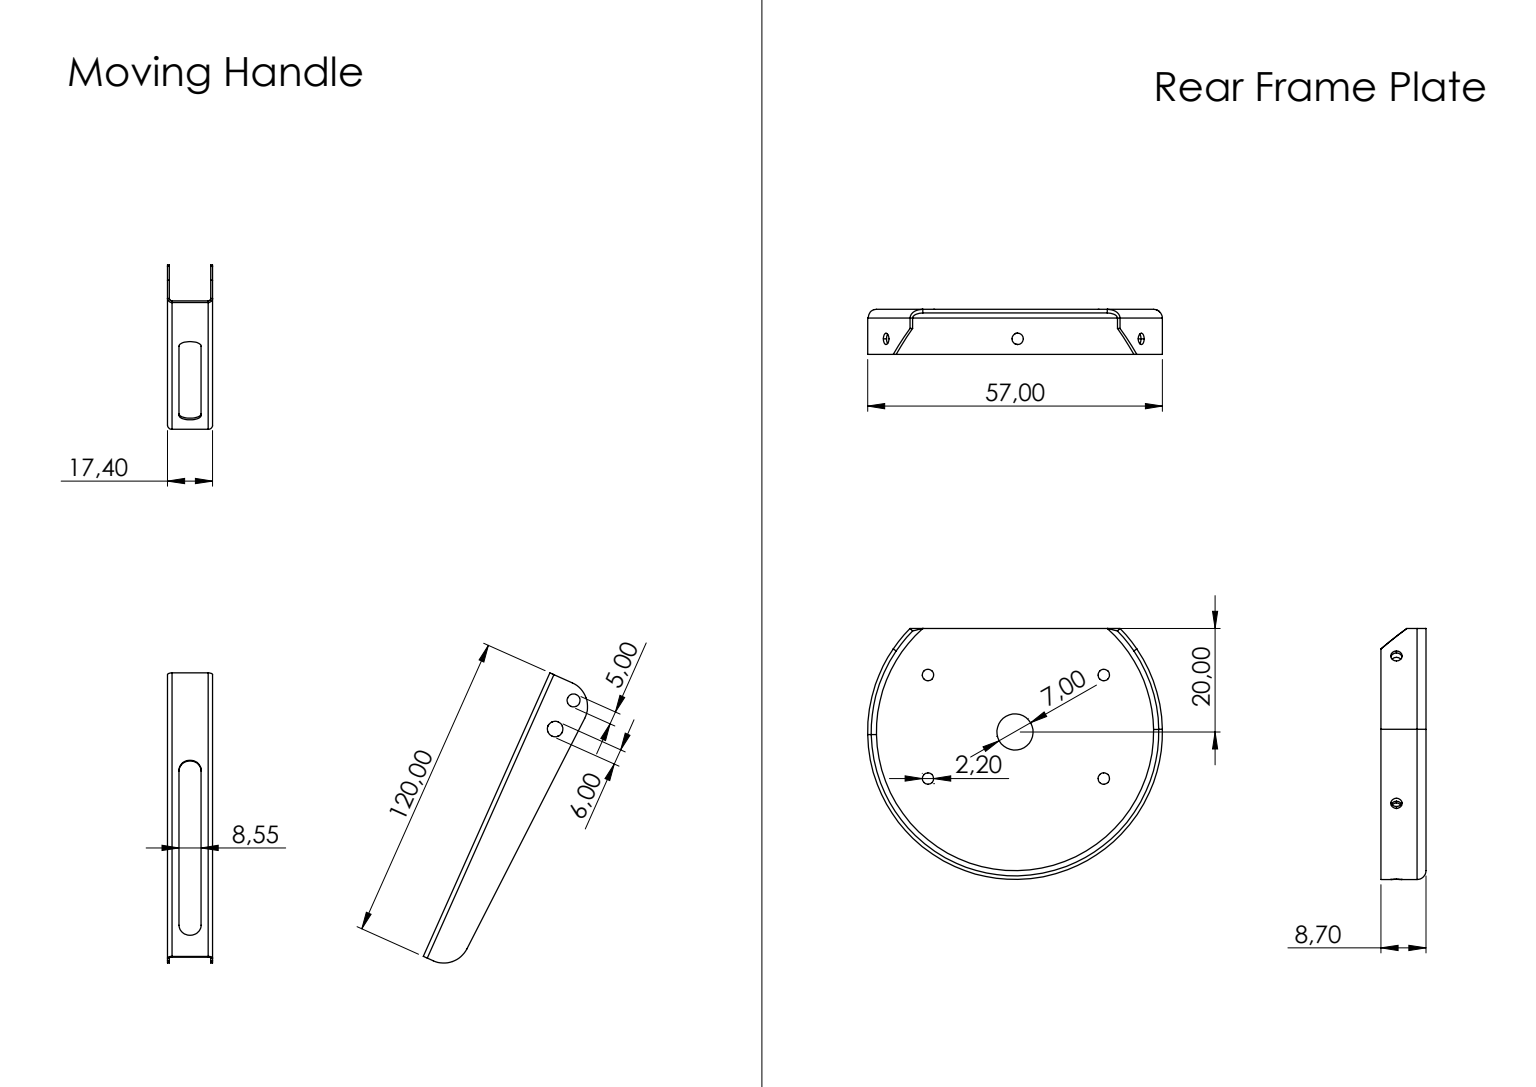
ISO-10303-21;
HEADER;
FILE_DESCRIPTION (('STEP AP214'),
    '1' );
FILE_NAME ('Rear Frame Plate.step',
    '2026-10-06T09:00:30',
    ( '' ),
    ( '' ),
    'SwSTEP 2.0',
    'SolidWorks 2020',
    '' );
FILE_SCHEMA (( 'AUTOMOTIVE_DESIGN' ));
ENDSEC;

DATA;
#10=CARTESIAN_POINT ( 'NONE',  ( -15.86372219731129896, -9.538245303637634009, -0.6999999999999785283 ) ) ;
#12=ORIENTED_EDGE ( 'NONE', *, *, #12651, .T. ) ;
#13=CARTESIAN_POINT ( 'NONE',  ( 25.25401215818320821, -13.21081861402980273, 4.098596794000014754 ) ) ;
#24=FACE_OUTER_BOUND ( 'NONE', #15323, .T. ) ;
#26=CARTESIAN_POINT ( 'NONE',  ( 18.18796211431769549, 19.99998853575082336, -0.6839386825886580867 ) ) ;
#31=ORIENTED_EDGE ( 'NONE', *, *, #12379, .F. ) ;
#36=B_SPLINE_CURVE_WITH_KNOTS ( 'NONE', 3,
 ( #5890, #1034, #22739, #5586, #10623, #27300 ),
 .UNSPECIFIED., .F., .F.,
 ( 4, 2, 4 ),
 ( 0.000000000000000000, 0.5000000000000000000, 1.000000000000000000 ),
 .UNSPECIFIED. ) ;
#37=CARTESIAN_POINT ( 'NONE',  ( 24.70074545475921823, -14.21822122957610368, 6.002806299999996043 ) ) ;
#38=CARTESIAN_POINT ( 'NONE',  ( 19.56389002122311638, 19.56882009050699622, 0.5006759800000037952 ) ) ;
#43=CARTESIAN_POINT ( 'NONE',  ( -24.83401023410189623, -13.98326748962921329, 4.239871886000001311 ) ) ;
#47=CARTESIAN_POINT ( 'NONE',  ( 0.5184513693225318853, -28.49550581263314086, 3.899998581000013509 ) ) ;
#51=CARTESIAN_POINT ( 'NONE',  ( -20.30403093128963476, 20.00000000003735323, 3.000000106999994642 ) ) ;
#65=CARTESIAN_POINT ( 'NONE',  ( 17.83929014045347827, 20.00000000006149392, -1.000005633855494125E-09 ) ) ;
#69=CARTESIAN_POINT ( 'NONE',  ( -18.27629205756926822, 19.99998488772503080, -0.6746503638753708065 ) ) ;
#72=MANIFOLD_SOLID_BREP ( 'PartBody', #5507 ) ;
#77=CARTESIAN_POINT ( 'NONE',  ( 16.21564467631812789, 10.42862492216662318, -0.6999999999999785283 ) ) ;
#88=CARTESIAN_POINT ( 'NONE',  ( -27.88265104574380260, 4.289521473631270787, 0.8585786439999909536 ) ) ;
#92=AXIS2_PLACEMENT_3D ( 'NONE', #8995, #11519, #1614 ) ;
#101=ADVANCED_FACE ( 'NONE', ( #28332 ), #9497, .F. ) ;
#103=CARTESIAN_POINT ( 'NONE',  ( 17.95841148951064525, -9.763538383420391042, -0.6999999999999784173 ) ) ;
#119=CARTESIAN_POINT ( 'NONE',  ( -24.32472894358752313, 13.45989150749028873, 3.899998581000013509 ) ) ;
#123=CARTESIAN_POINT ( 'NONE',  ( 17.93011078765611543, -8.208160914697428368, -0.6999999999999784173 ) ) ;
#126=CARTESIAN_POINT ( 'NONE',  ( 19.80526555972147307, 19.50877392102524155, 1.800000000000023803 ) ) ;
#144=DIRECTION ( 'NONE',  ( -0.6941258031311203780, -0.7198537139083029945, 0.000000000000000000 ) ) ;
#153=CARTESIAN_POINT ( 'NONE',  ( -18.31085446006445494, 19.88197403644849004, 0.02160863700001458554 ) ) ;
#164=FACE_OUTER_BOUND ( 'NONE', #30752, .T. ) ;
#170=VERTEX_POINT ( 'NONE', #24397 ) ;
#171=CARTESIAN_POINT ( 'NONE',  ( -17.59696554489119080, -9.791838634853515799, 0.000000000000000000 ) ) ;
#174=CARTESIAN_POINT ( 'NONE',  ( 23.47715715134837211, -20.00370206646827498, 1.000000000000000888 ) ) ;
#176=CARTESIAN_POINT ( 'NONE',  ( 19.80526555972147307, 19.50877392102524155, 8.000000000000007105 ) ) ;
#178=CARTESIAN_POINT ( 'NONE',  ( 19.37011161855012986, 20.00004249230521935, -0.3429596948707999693 ) ) ;
#179=CARTESIAN_POINT ( 'NONE',  ( -24.00289803497245700, 14.02635913871703011, 5.901399683999997592 ) ) ;
#198=CARTESIAN_POINT ( 'NONE',  ( 16.37473331889771089, 11.76353838340827984, 0.000000000000000000 ) ) ;
#214=CARTESIAN_POINT ( 'NONE',  ( -24.82162973577514364, 12.51998933611906573, 5.310645680000003921 ) ) ;
#219=CARTESIAN_POINT ( 'NONE',  ( 3.040504021322313122, 1.733590290792417887, 0.000000000000000000 ) ) ;
#245=ADVANCED_FACE ( 'NONE', ( #491 ), #28838, .T. ) ;
#250=LINE ( 'NONE', #26663, #23008 ) ;
#254=CARTESIAN_POINT ( 'NONE',  ( -18.80686365405603055, 19.99999823163966184, -0.5856999480000069092 ) ) ;
#257=B_SPLINE_SURFACE_WITH_KNOTS ( 'NONE', 5, 1, ( 
 ( #21157, #21469 ),
 ( #23836, #30754 ),
 ( #16430, #9183 ),
 ( #14231, #2282 ),
 ( #11866, #28394 ),
 ( #6831, #11711 ),
 ( #21312, #7144 ),
 ( #26039, #4479 ),
 ( #11245, #28076 ),
 ( #9342, #20853 ),
 ( #18943, #26346 ),
 ( #4794, #7602 ),
 ( #19727, #10128 ),
 ( #21937, #19414 ),
 ( #26800, #17195 ) ),
 .UNSPECIFIED., .F., .F., .F.,
 ( 6, 3, 3, 3, 6 ),
 ( 2, 2 ),
 ( 0.000000000000000000, 0.5239015562240000312, 1.047803112450000018, 1.571704668670000027, 1.746338520749999956 ),
 ( -0.7000000000009999335, 2.556819966299999618E-06 ),
 .UNSPECIFIED. ) ;
#269=CARTESIAN_POINT ( 'NONE',  ( -23.23277126416379801, -15.26692729116844482, 5.104183903000020450 ) ) ;
#272=STYLED_ITEM ( 'NONE', ( #2224 ), #72 ) ;
#275=CARTESIAN_POINT ( 'NONE',  ( -4.583497702006505747, -30.37373325290905868, -0.6577119969999878357 ) ) ;
#279=CARTESIAN_POINT ( 'NONE',  ( 28.49528339128749366, 0.5184828350247753237, 8.000000000000007105 ) ) ;
#282=CARTESIAN_POINT ( 'NONE',  ( -16.81618662976075740, -7.899504219251200610, 0.000000000000000000 ) ) ;
#283=CARTESIAN_POINT ( 'NONE',  ( 24.86822223037987456, 13.92223202030449691, 5.680679506000013923 ) ) ;
#284=EDGE_CURVE ( 'NONE', #12548, #25224, #27851, .T. ) ;
#286=CARTESIAN_POINT ( 'NONE',  ( 20.30396079662882158, 20.00000000004802203, 2.200000000000007283 ) ) ;
#291=EDGE_CURVE ( 'NONE', #28488, #24538, #21849, .T. ) ;
#295=ORIENTED_EDGE ( 'NONE', *, *, #24858, .F. ) ;
#301=CARTESIAN_POINT ( 'NONE',  ( -27.79539923781684507, -0.5057481689249115897, 6.600000000000022737 ) ) ;
#307=ORIENTED_EDGE ( 'NONE', *, *, #28551, .T. ) ;
#309=CARTESIAN_POINT ( 'NONE',  ( -24.96253706803760153, -13.75225324404262572, 4.689458291000009105 ) ) ;
#325=ORIENTED_EDGE ( 'NONE', *, *, #21114, .F. ) ;
#326=CARTESIAN_POINT ( 'NONE',  ( 25.05552768372066907, -13.58331698798256504, 3.920132093000017193 ) ) ;
#335=CARTESIAN_POINT ( 'NONE',  ( 17.14656078599760392, 12.09981795542235439, -0.6999999999999784173 ) ) ;
#347=CARTESIAN_POINT ( 'NONE',  ( -1.108738578190967550, -3.350312884103880950, 0.000000000000000000 ) ) ;
#349=CARTESIAN_POINT ( 'NONE',  ( 23.83639842146205368, 14.30623132797946084, 6.099998581000020792 ) ) ;
#353=EDGE_CURVE ( 'NONE', #27389, #17896, #14711, .T. ) ;
#365=ORIENTED_EDGE ( 'NONE', *, *, #11993, .F. ) ;
#367=ORIENTED_EDGE ( 'NONE', *, *, #29552, .F. ) ;
#415=CARTESIAN_POINT ( 'NONE',  ( -23.47637529058820860, -14.89020704899713365, 4.098700198000015504 ) ) ;
#416=B_SPLINE_SURFACE_WITH_KNOTS ( 'NONE', 5, 1, ( 
 ( #8599, #18199 ),
 ( #6254, #14591 ),
 ( #24030, #21979 ),
 ( #14278, #7033 ),
 ( #4834, #16622 ),
 ( #17088, #24179 ),
 ( #30954, #26082 ),
 ( #19146, #23884 ),
 ( #18832, #2323 ),
 ( #2471, #16469 ),
 ( #21669, #26392 ),
 ( #16775, #28434 ),
 ( #9549, #14431 ),
 ( #2781, #4521 ),
 ( #14119, #119 ) ),
 .UNSPECIFIED., .F., .F., .F.,
 ( 6, 3, 3, 3, 6 ),
 ( 2, 2 ),
 ( 0.000000000000000000, 0.5239049113340000785, 1.047809822670000113, 1.571714733999999947, 1.746349704450000040 ),
 ( -0.7000000000009999335, 2.557518061549999935E-06 ),
 .UNSPECIFIED. ) ;
#417=CARTESIAN_POINT ( 'NONE',  ( -19.80535397421925481, 19.50875616500616871, 0.9999999989999952543 ) ) ;
#434=CARTESIAN_POINT ( 'NONE',  ( -28.35945636591989683, -7.983396444576476902, 0.7595836940000044724 ) ) ;
#442=VECTOR ( 'NONE', #12389, 1000.000000000000000 ) ;
#443=CARTESIAN_POINT ( 'NONE',  ( 19.80526555962148549, 19.50877392102342256, 1.000000000000000888 ) ) ;
#455=CARTESIAN_POINT ( 'NONE',  ( -16.66884554142874464, -10.09718743908464234, -0.6999999999999783062 ) ) ;
#479=ORIENTED_EDGE ( 'NONE', *, *, #10437, .F. ) ;
#490=CARTESIAN_POINT ( 'NONE',  ( -16.83342759575507586, 10.99999999997565503, -0.6999999999999784173 ) ) ;
#491=FACE_OUTER_BOUND ( 'NONE', #749, .T. ) ;
#510=CARTESIAN_POINT ( 'NONE',  ( 0.5057536231481192246, -27.79562098839016571, 6.099998581000020792 ) ) ;
#511=CARTESIAN_POINT ( 'NONE',  ( -23.81866173682177390, -14.33570044646243247, 3.899998581000013509 ) ) ;
#512=CARTESIAN_POINT ( 'NONE',  ( 16.27478637877570833, 11.65988689034672809, -4.336808689942018722E-16 ) ) ;
#519=B_SPLINE_CURVE_WITH_KNOTS ( 'NONE', 5,
 ( #763, #19799, #26878, #10508, #7824, #14617, #22156, #5319, #27336, #14923, #24519, #22311, #2956, #20108, #29696 ),
 .UNSPECIFIED., .F., .F.,
 ( 6, 3, 3, 3, 6 ),
 ( 0.000000000000000000, 0.3000000000005726419, 0.6000000000000000888, 0.9000000000028631764, 1.000000000000000000 ),
 .UNSPECIFIED. ) ;
#534=CARTESIAN_POINT ( 'NONE',  ( -24.78870452935070290, 12.58522324297991268, 5.507123707999994622 ) ) ;
#535=FACE_BOUND ( 'NONE', #29200, .T. ) ;
#539=AXIS2_PLACEMENT_3D ( 'NONE', #23049, #13598, #18623 ) ;
#556=CARTESIAN_POINT ( 'NONE',  ( -26.39324905318550307, 9.701294701415816846, 8.000000000000007105 ) ) ;
#573=CARTESIAN_POINT ( 'NONE',  ( -25.38146355678814814, 12.59839640969361696, 1.000000000000000888 ) ) ;
#581=CARTESIAN_POINT ( 'NONE',  ( -23.25311087912443853, -15.23597700045676895, 5.310552105000033052 ) ) ;
#586=CARTESIAN_POINT ( 'NONE',  ( -4.785279987089964493, -31.71089578132167119, 1.000000000000000888 ) ) ;
#601=ORIENTED_EDGE ( 'NONE', *, *, #21982, .T. ) ;
#603=CARTESIAN_POINT ( 'NONE',  ( -24.29138540600951046, 13.52003710149997140, 3.901342110999989288 ) ) ;
#609=AXIS2_PLACEMENT_3D ( 'NONE', #4921, #21294, #28527 ) ;
#623=EDGE_CURVE ( 'NONE', #12633, #11464, #6060, .T. ) ;
#654=CARTESIAN_POINT ( 'NONE',  ( 24.92013865993870425, -13.82966158318416738, 6.099998581000020792 ) ) ;
#655=CARTESIAN_POINT ( 'NONE',  ( 24.66346747934004568, 14.28208995973567141, 6.002748562000004284 ) ) ;
#672=ORIENTED_EDGE ( 'NONE', *, *, #1632, .F. ) ;
#678=CARTESIAN_POINT ( 'NONE',  ( -16.06988921231594603, 11.79183908526949054, -0.6999999999999784173 ) ) ;
#681=CARTESIAN_POINT ( 'NONE',  ( -24.83827471527357744, 12.48687850854618198, 4.999998581000003384 ) ) ;
#693=B_SPLINE_CURVE_WITH_KNOTS ( 'NONE', 1,
 ( #19992, #29587 ),
 .UNSPECIFIED., .F., .F.,
 ( 2, 2 ),
 ( -3.500000000000000000, -1.499999893000000029 ),
 .UNSPECIFIED. ) ;
#698=CARTESIAN_POINT ( 'NONE',  ( -3.415131430766694010, -0.8926240818011570433, -0.6999999999999785283 ) ) ;
#699=CARTESIAN_POINT ( 'NONE',  ( 18.26639035964474900, 11.02001161816309072, -0.6999999989999727834 ) ) ;
#704=CARTESIAN_POINT ( 'NONE',  ( -18.48840142452550594, 20.72769736509012262, 0.7069223289999926330 ) ) ;
#711=ORIENTED_EDGE ( 'NONE', *, *, #9275, .F. ) ;
#718=CARTESIAN_POINT ( 'NONE',  ( -28.49528339128749366, -0.5184828350247461248, 0.7595836940000044724 ) ) ;
#732=CARTESIAN_POINT ( 'NONE',  ( 28.49528339128749366, 0.5184828350247212558, 1.000000000000000888 ) ) ;
#736=CARTESIAN_POINT ( 'NONE',  ( -27.29371452669260734, -0.4966198192113812637, -0.6577119969999878357 ) ) ;
#743=ORIENTED_EDGE ( 'NONE', *, *, #1777, .T. ) ;
#748=EDGE_LOOP ( 'NONE', ( #15033, #19487, #856, #4347 ) ) ;
#749=EDGE_LOOP ( 'NONE', ( #24404, #672, #17249, #8267 ) ) ;
#750=CARTESIAN_POINT ( 'NONE',  ( -20.06986697712849121, -20.94709743681733727, 0.2686753820000109538 ) ) ;
#751=EDGE_LOOP ( 'NONE', ( #2180, #29405, #19550, #13095 ) ) ;
#756=CARTESIAN_POINT ( 'NONE',  ( -19.80535357367646654, 19.50875577052770993, 5.200000000000009948 ) ) ;
#763=CARTESIAN_POINT ( 'NONE',  ( 24.98081130624543889, 13.71897605842228529, 4.999998581000003384 ) ) ;
#772=ADVANCED_FACE ( 'NONE', ( #6236 ), #4729, .F. ) ;
#777=CARTESIAN_POINT ( 'NONE',  ( -16.95738181130097288, -10.10243747011873872, -0.6999999999999783062 ) ) ;
#792=CARTESIAN_POINT ( 'NONE',  ( 24.66346747934186112, 14.28208995963568739, 3.997248600000002927 ) ) ;
#795=EDGE_CURVE ( 'NONE', #974, #18728, #25586, .T. ) ;
#805=EDGE_CURVE ( 'NONE', #28870, #3434, #12807, .T. ) ;
#818=ORIENTED_EDGE ( 'NONE', *, *, #11201, .T. ) ;
#830=LINE ( 'NONE', #18100, #19769 ) ;
#833=CARTESIAN_POINT ( 'NONE',  ( 0.5184513693225726305, -28.49550581263314086, 6.099998581000020792 ) ) ;
#834=CARTESIAN_POINT ( 'NONE',  ( 19.76603533419210734, 19.51852340513930173, 0.7754612589999931860 ) ) ;
#847=CARTESIAN_POINT ( 'NONE',  ( -3.046043134630462390, 1.783682052046422939, -0.6999999999999784173 ) ) ;
#850=ORIENTED_EDGE ( 'NONE', *, *, #20772, .T. ) ;
#852=CARTESIAN_POINT ( 'NONE',  ( 26.71513120331084679, 4.908099852734520319, 0.000000000000000000 ) ) ;
#856=ORIENTED_EDGE ( 'NONE', *, *, #2374, .F. ) ;
#862=CARTESIAN_POINT ( 'NONE',  ( 17.18658402241074867, -10.09981795543446736, -0.6999999989999727834 ) ) ;
#865=CARTESIAN_POINT ( 'NONE',  ( 0.8057560762813021915, -28.48917411425644275, 6.073787920303829857 ) ) ;
#867=CARTESIAN_POINT ( 'NONE',  ( -27.61404081990094994, 9.332834367751024374, 0.7595836940000044724 ) ) ;
#884=CARTESIAN_POINT ( 'NONE',  ( 14.58748419594687817, -28.00135611681330516, 0.5017677510000262409 ) ) ;
#887=ORIENTED_EDGE ( 'NONE', *, *, #20994, .F. ) ;
#904=CARTESIAN_POINT ( 'NONE',  ( 14.23756994129695030, -27.32973605077160073, 0.7069240339999949274 ) ) ;
#907=CARTESIAN_POINT ( 'NONE',  ( 16.59368952141597831, 11.95034963011661944, -0.6999999999999784173 ) ) ;
#909=CARTESIAN_POINT ( 'NONE',  ( 24.95427444975690889, -13.76797447160702070, 3.899998581000013509 ) ) ;
#921=CARTESIAN_POINT ( 'NONE',  ( 20.30396079652883756, 20.00000000004620304, 1.000000000000000888 ) ) ;
#931=VERTEX_POINT ( 'NONE', #12655 ) ;
#946=CARTESIAN_POINT ( 'NONE',  ( 24.96253706050071131, 13.75225324050492581, 4.689458287000014991 ) ) ;
#948=CARTESIAN_POINT ( 'NONE',  ( 0.5057536231481192246, -27.79562098839016571, 6.099998581000020792 ) ) ;
#960=ADVANCED_FACE ( 'NONE', ( #23523 ), #10927, .F. ) ;
#961=CARTESIAN_POINT ( 'NONE',  ( 18.92356420714367360, 19.72862907665551546, 0.1494310229999962214 ) ) ;
#966=CARTESIAN_POINT ( 'NONE',  ( 25.80996960090668679, 10.85703805089278617, 1.000000000000000888 ) ) ;
#967=EDGE_LOOP ( 'NONE', ( #12615, #17366 ) ) ;
#968=AXIS2_PLACEMENT_3D ( 'NONE', #3100, #14920, #144 ) ;
#974=VERTEX_POINT ( 'NONE', #13912 ) ;
#980=CARTESIAN_POINT ( 'NONE',  ( -17.49331448440255343, 10.10821397335649152, -0.6999999999999784173 ) ) ;
#984=FILL_AREA_STYLE_COLOUR ( '', #18846 ) ;
#986=CARTESIAN_POINT ( 'NONE',  ( -24.70450124751183552, 12.74984379616985386, 5.760266710000017554 ) ) ;
#987=CARTESIAN_POINT ( 'NONE',  ( 4.785280386522178020, 31.71089591180988876, 1.000000000000000888 ) ) ;
#1011=VERTEX_POINT ( 'NONE', #27918 ) ;
#1014=EDGE_LOOP ( 'NONE', ( #29479, #29790, #6627, #16562 ) ) ;
#1021=CARTESIAN_POINT ( 'NONE',  ( -25.96688743241739061, 8.776138983998601262, -0.6999999999999784173 ) ) ;
#1026=ORIENTED_EDGE ( 'NONE', *, *, #11785, .F. ) ;
#1033=CARTESIAN_POINT ( 'NONE',  ( 21.36643726116283659, 17.24662705154594988, 0.02487530000000459651 ) ) ;
#1034=CARTESIAN_POINT ( 'NONE',  ( 16.29899378166743062, -9.691472637822489133, 0.000000000000000000 ) ) ;
#1036=CARTESIAN_POINT ( 'NONE',  ( -23.23277431133845994, -15.26692929363520257, 4.999998581000003384 ) ) ;
#1051=EDGE_LOOP ( 'NONE', ( #1208, #22338, #9654, #26005 ) ) ;
#1053=FACE_OUTER_BOUND ( 'NONE', #3329, .T. ) ;
#1060=CARTESIAN_POINT ( 'NONE',  ( 24.83827472153076599, -12.48687851163286133, 5.104216618000034345 ) ) ;
#1089=CARTESIAN_POINT ( 'NONE',  ( 24.14840829003316003, 13.77363891342296043, 4.098702612000016288 ) ) ;
#1090=CARTESIAN_POINT ( 'NONE',  ( 17.33054985630230505, 9.902801559281119381, -4.336808689942018722E-16 ) ) ;
#1097=CARTESIAN_POINT ( 'NONE',  ( -22.97593529893700648, 15.65128280014837081, 8.000000000000007105 ) ) ;
#1103=FACE_BOUND ( 'NONE', #21065, .T. ) ;
#1108=CARTESIAN_POINT ( 'NONE',  ( 17.99934522968721495, 20.17941515401252417, -0.6999999999999784173 ) ) ;
#1111=EDGE_LOOP ( 'NONE', ( #26780, #25862, #20091, #12457 ) ) ;
#1114=CYLINDRICAL_SURFACE ( 'NONE', #26357, 1.100000000000002309 ) ;
#1123=ORIENTED_EDGE ( 'NONE', *, *, #11315, .F. ) ;
#1124=B_SPLINE_CURVE_WITH_KNOTS ( 'NONE', 3,
 ( #23450, #1880, #6119, #11478, #30363, #30677, #8791, #22968, #3599, #6436, #1259, #28303 ),
 .UNSPECIFIED., .F., .F.,
 ( 4, 2, 2, 2, 2, 4 ),
 ( 0.000000000000000000, 0.2500000000000007216, 0.5000000000000014433, 0.6250000000000013323, 0.7500000000000012212, 1.000000000000000000 ),
 .UNSPECIFIED. ) ;
#1129=CARTESIAN_POINT ( 'NONE',  ( -24.34137756212881953, 13.42980562992878646, 6.099998581000020792 ) ) ;
#1130=FACE_OUTER_BOUND ( 'NONE', #3387, .T. ) ;
#1137=DIRECTION ( 'NONE',  ( 0.000000000000000000, 0.000000000000000000, -1.000000000000000000 ) ) ;
#1152=ORIENTED_EDGE ( 'NONE', *, *, #20095, .T. ) ;
#1153=CARTESIAN_POINT ( 'NONE',  ( -25.96688743241757535, 8.776138984008598598, 0.000000000000000000 ) ) ;
#1160=ORIENTED_EDGE ( 'NONE', *, *, #22690, .F. ) ;
#1170=CARTESIAN_POINT ( 'NONE',  ( -24.73836043327892042, 13.50621019268970713, -0.5592437529999827461 ) ) ;
#1171=DIRECTION ( 'NONE',  ( 0.000000000000000000, 0.000000000000000000, -1.000000000000000000 ) ) ;
#1179=CARTESIAN_POINT ( 'NONE',  ( 23.55411374389282386, 16.04538543799059980, 8.000000000000007105 ) ) ;
#1183=CARTESIAN_POINT ( 'NONE',  ( -24.16679028379773797, -15.10730798416152609, 6.002747143000003227 ) ) ;
#1184=CARTESIAN_POINT ( 'NONE',  ( 24.71356588429207690, 13.94368305229924232, 0.8585785770000020634 ) ) ;
#1196=CARTESIAN_POINT ( 'NONE',  ( -16.83342759582943060, -8.999999999996580513, -0.6999999999999784173 ) ) ;
#1207=CARTESIAN_POINT ( 'NONE',  ( 27.11703666554969416, -9.406552224315994692, 0.000000000000000000 ) ) ;
#1208=ORIENTED_EDGE ( 'NONE', *, *, #5748, .F. ) ;
#1211=CARTESIAN_POINT ( 'NONE',  ( 16.37473331889771089, 11.76353838340827984, -0.6999999999999784173 ) ) ;
#1214=CARTESIAN_POINT ( 'NONE',  ( -15.75643827148868681, 10.73282780873525866, -0.6999999999999784173 ) ) ;
#1217=CARTESIAN_POINT ( 'NONE',  ( 25.46368747440213198, -12.80129684534102807, 5.104216618000034345 ) ) ;
#1220=CARTESIAN_POINT ( 'NONE',  ( 4.785280386522178020, 31.71089591180988876, 1.000000000000000888 ) ) ;
#1237=CARTESIAN_POINT ( 'NONE',  ( 18.26639035967037827, -8.979988381807324060, -1.000005633855494125E-09 ) ) ;
#1250=CARTESIAN_POINT ( 'NONE',  ( -17.64325308166371542, -9.745514112911177307, 0.000000000000000000 ) ) ;
#1251=CARTESIAN_POINT ( 'NONE',  ( -0.04427422412647075145, -27.80047756270342063, 5.964026387038768640 ) ) ;
#1259=CARTESIAN_POINT ( 'NONE',  ( 25.46368747440757474, -12.80129684534242074, 5.147587687417541247 ) ) ;
#1260=VECTOR ( 'NONE', #28010, 1000.000000000000000 ) ;
#1268=CYLINDRICAL_SURFACE ( 'NONE', #30824, 1.099999999999999867 ) ;
#1275=CARTESIAN_POINT ( 'NONE',  ( 24.38199545065365115, 14.75707034588002564, 6.098654095000016540 ) ) ;
#1283=ORIENTED_EDGE ( 'NONE', *, *, #28659, .F. ) ;
#1285=B_SPLINE_CURVE_WITH_KNOTS ( 'NONE', 1,
 ( #3231, #27001 ),
 .UNSPECIFIED., .F., .F.,
 ( 2, 2 ),
 ( -2.555885125540000124E-06, 0.7000000000009999335 ),
 .UNSPECIFIED. ) ;
#1291=CARTESIAN_POINT ( 'NONE',  ( -24.63376349509220731, 12.88634507999193701, 5.901400367999992902 ) ) ;
#1301=CARTESIAN_POINT ( 'NONE',  ( 24.36724931188768650, 13.38201648792073684, 4.999998581000003384 ) ) ;
#1317=ORIENTED_EDGE ( 'NONE', *, *, #28659, .T. ) ;
#1334=EDGE_LOOP ( 'NONE', ( #21837, #26282, #22665, #4141 ) ) ;
#1342=CARTESIAN_POINT ( 'NONE',  ( 18.50495734104858414, 20.74627095498905049, 0.8585787200000027930 ) ) ;
#1349=CARTESIAN_POINT ( 'NONE',  ( 24.09407739349445876, -13.86899051613567480, 3.997190862000010725 ) ) ;
#1355=CARTESIAN_POINT ( 'NONE',  ( 26.19759702725205486, 6.104572563141537955, -0.6999999999999784173 ) ) ;
#1364=CARTESIAN_POINT ( 'NONE',  ( -20.24759346773182855, -21.13259110598446355, 0.7069231350000093617 ) ) ;
#1367=CARTESIAN_POINT ( 'NONE',  ( -23.25311087902445450, -15.23597700045494996, 4.689445057000002137 ) ) ;
#1369=CARTESIAN_POINT ( 'NONE',  ( 2.635643612059070051, 2.346759556412466363, 0.000000000000000000 ) ) ;
#1376=LINE ( 'NONE', #30160, #4251 ) ;
#1384=CARTESIAN_POINT ( 'NONE',  ( 17.16657240419154462, 10.99999999996915179, -0.6999999999999784173 ) ) ;
#1385=CARTESIAN_POINT ( 'NONE',  ( -15.76765990785340676, -8.693620616903867671, -0.6999999999999785283 ) ) ;
#1391=CARTESIAN_POINT ( 'NONE',  ( -17.37135892817496696, 10.02943855699536613, -0.000000000000000000 ) ) ;
#1406=CARTESIAN_POINT ( 'NONE',  ( -17.92646393081800582, -9.131743399318690280, 0.000000000000000000 ) ) ;
#1422=CARTESIAN_POINT ( 'NONE',  ( -14.55829176637774935, -23.98013756361786974, 8.000000000000007105 ) ) ;
#1426=CARTESIAN_POINT ( 'NONE',  ( 0.1319790757220171973, -27.80015609199433158, 3.957670871000018575 ) ) ;
#1430=CARTESIAN_POINT ( 'NONE',  ( 23.87963657767028280, 15.55698410313905988, 5.506989593000027661 ) ) ;
#1460=B_SPLINE_CURVE_WITH_KNOTS ( 'NONE', 3,
 ( #24696, #12889, #8581, #3131, #3879, #3285 ),
 .UNSPECIFIED., .F., .F.,
 ( 4, 2, 4 ),
 ( 0.000000000000000000, 0.5000000000000000000, 1.000000000000000000 ),
 .UNSPECIFIED. ) ;
#1482=EDGE_CURVE ( 'NONE', #3709, #30998, #2661, .T. ) ;
#1494=CARTESIAN_POINT ( 'NONE',  ( -25.25401215124432852, 13.21081861195569296, 4.098596794000014754 ) ) ;
#1504=CARTESIAN_POINT ( 'NONE',  ( 18.32611613475859258, 20.54576746904009710, 0.2686742950000209351 ) ) ;
#1525=CARTESIAN_POINT ( 'NONE',  ( -24.64719444845753671, -14.72745526642161451, 0.08279798700003282441 ) ) ;
#1531=LINE ( 'NONE', #30484, #20482 ) ;
#1532=CARTESIAN_POINT ( 'NONE',  ( -0.4969045691571343237, -28.49594262166996828, 4.493528488000025689 ) ) ;
#1549=CARTESIAN_POINT ( 'NONE',  ( -17.59696597919420213, 10.20816091468181774, 0.000000000000000000 ) ) ;
#1550=CARTESIAN_POINT ( 'NONE',  ( 17.95841148948556310, 10.23646161652002817, -0.6999999999999784173 ) ) ;
#1557=VERTEX_POINT ( 'NONE', #11725 ) ;
#1565=CARTESIAN_POINT ( 'NONE',  ( -0.1620084139599508588, -27.79990535609617197, 5.886603267324479027 ) ) ;
#1580=CARTESIAN_POINT ( 'NONE',  ( -19.06860189597471944, 19.69237645765742073, 0.2003674019999956979 ) ) ;
#1581=CARTESIAN_POINT ( 'NONE',  ( 25.74138181328865826, -11.15269228347309038, 8.000000000000007105 ) ) ;
#1583=CARTESIAN_POINT ( 'NONE',  ( -23.23277431133845994, -15.26692929363520257, 4.999998581000003384 ) ) ;
#1614=DIRECTION ( 'NONE',  ( 0.7198537139083028835, -0.6941258031311204890, 0.000000000000000000 ) ) ;
#1619=CARTESIAN_POINT ( 'NONE',  ( -17.72558663072204155, 11.65945330601512175, -0.6999999999999783062 ) ) ;
#1625=EDGE_CURVE ( 'NONE', #3626, #8936, #3622, .T. ) ;
#1632=EDGE_CURVE ( 'NONE', #30700, #30026, #3779, .T. ) ;
#1637=EDGE_LOOP ( 'NONE', ( #5645, #24469, #17522, #7195 ) ) ;
#1647=VERTEX_POINT ( 'NONE', #27238 ) ;
#1657=CARTESIAN_POINT ( 'NONE',  ( 26.79556473285982321, 0.4875557887249727385, 0.000000000000000000 ) ) ;
#1660=CARTESIAN_POINT ( 'NONE',  ( -23.76534794678204321, -14.42397063190348483, 6.095965061000018892 ) ) ;
#1664=CARTESIAN_POINT ( 'NONE',  ( -17.83930458849792089, 19.99999999999597478, -1.000005633855494125E-09 ) ) ;
#1666=EDGE_CURVE ( 'NONE', #17343, #27013, #22991, .T. ) ;
#1667=CARTESIAN_POINT ( 'NONE',  ( 3.046043134278133557, -1.783682052637085125, -0.6999999999999784173 ) ) ;
#1674=CARTESIAN_POINT ( 'NONE',  ( 24.77037083723135780, -12.62110030509766645, 4.441416311653765270 ) ) ;
#1682=DIRECTION ( 'NONE',  ( 0.000000000000000000, 0.000000000000000000, -1.000000000000000000 ) ) ;
#1683=CARTESIAN_POINT ( 'NONE',  ( 0.5057536231481327693, -27.79562098839016571, 3.899998581000013509 ) ) ;
#1684=CARTESIAN_POINT ( 'NONE',  ( -16.09019580745308176, -9.813945847455975979, 0.000000000000000000 ) ) ;
#1686=ORIENTED_EDGE ( 'NONE', *, *, #20758, .T. ) ;
#1687=FACE_BOUND ( 'NONE', #30689, .T. ) ;
#1688=CARTESIAN_POINT ( 'NONE',  ( 27.51770821245201759, 4.728187301810311105, 8.000000000000007105 ) ) ;
#1698=CARTESIAN_POINT ( 'NONE',  ( 27.08859402333790101, 0.4928875713652651203, 0.02487529600000981667 ) ) ;
#1725=LINE ( 'NONE', #21080, #29557 ) ;
#1731=CARTESIAN_POINT ( 'NONE',  ( 27.55801272791059731, 0.5014288284349825986, -0.5592437529999827461 ) ) ;
#1734=CARTESIAN_POINT ( 'NONE',  ( -28.34732274966954790, -3.134629491153491987, 8.000000000000007105 ) ) ;
#1740=CARTESIAN_POINT ( 'NONE',  ( -0.5944614571882205212, -27.79380703160649446, 4.895947184000021046 ) ) ;
#1761=CARTESIAN_POINT ( 'NONE',  ( -24.29089620838935204, -14.90695587844356673, 3.920145809000019632 ) ) ;
#1763=CARTESIAN_POINT ( 'NONE',  ( -0.3076636919694037964, -28.49867017228337573, 4.240370246000018994 ) ) ;
#1764=EDGE_CURVE ( 'NONE', #30855, #1904, #14298, .T. ) ;
#1773=FACE_BOUND ( 'NONE', #1786, .T. ) ;
#1777=EDGE_CURVE ( 'NONE', #23829, #25431, #8605, .T. ) ;
#1779=CARTESIAN_POINT ( 'NONE',  ( 0.8794532062938354988, -27.78659480101258694, 6.042323509000024906 ) ) ;
#1783=CARTESIAN_POINT ( 'NONE',  ( -23.83437493864195389, -15.62616283475966661, 5.290530235267004500 ) ) ;
#1786=EDGE_LOOP ( 'NONE', ( #12509, #4725, #14097, #22822, #2263, #20982, #11767, #26636 ) ) ;
#1799=CARTESIAN_POINT ( 'NONE',  ( 27.79539923781684507, 0.5057481689249235801, 8.000000000000007105 ) ) ;
#1804=EDGE_CURVE ( 'NONE', #13930, #18290, #10758, .T. ) ;
#1821=CARTESIAN_POINT ( 'NONE',  ( 16.37473331889771089, 11.76353838340827984, -0.6999999999999784173 ) ) ;
#1826=CARTESIAN_POINT ( 'NONE',  ( 1.335589245615521836, -3.267430459516901475, -0.6999999999999783062 ) ) ;
#1839=CARTESIAN_POINT ( 'NONE',  ( 0.5184513693225318853, -28.49550581263314086, 3.899998581000013509 ) ) ;
#1843=ORIENTED_EDGE ( 'NONE', *, *, #15798, .F. ) ;
#1844=CARTESIAN_POINT ( 'NONE',  ( -28.68577476999353237, 9.950727454195712696, 1.000000000000000888 ) ) ;
#1847=CARTESIAN_POINT ( 'NONE',  ( -16.01886467873034547, -9.739971655381781446, 0.000000000000000000 ) ) ;
#1854=DIRECTION ( 'NONE',  ( 0.000000000000000000, 0.000000000000000000, -1.000000000000000000 ) ) ;
#1875=CARTESIAN_POINT ( 'NONE',  ( -16.99740504728543655, 12.09719844076589013, -4.336808689942018722E-16 ) ) ;
#1880=CARTESIAN_POINT ( 'NONE',  ( 25.00848081462686068, -13.67001763210799758, 6.099998580999997699 ) ) ;
#1885=CARTESIAN_POINT ( 'NONE',  ( 1.498515220174240659, -28.61801908170006925, 8.000000000000007105 ) ) ;
#1889=CARTESIAN_POINT ( 'NONE',  ( 26.79556473285982321, 0.4875557887249821198, -0.6999999999999784173 ) ) ;
#1897=CARTESIAN_POINT ( 'NONE',  ( -17.83908356944316864, -8.536708948802910868, 0.000000000000000000 ) ) ;
#1904=VERTEX_POINT ( 'NONE', #22573 ) ;
#1908=CARTESIAN_POINT ( 'NONE',  ( 23.77307027441306531, -14.41181805765238444, 4.999998581000003384 ) ) ;
#1909=CARTESIAN_POINT ( 'NONE',  ( 24.41841038956698640, 14.69667349781389376, 3.899998581000013509 ) ) ;
#1910=CARTESIAN_POINT ( 'NONE',  ( -24.21906834513991313, -15.02342241408235068, 3.957526371000025023 ) ) ;
#1913=B_SPLINE_CURVE_WITH_KNOTS ( 'NONE', 1,
 ( #30730, #51 ),
 .UNSPECIFIED., .F., .F.,
 ( 2, 2 ),
 ( -0.0003775010496399999857, 0.7000000000080000007 ),
 .UNSPECIFIED. ) ;
#1915=VECTOR ( 'NONE', #13110, 1000.000000000000000 ) ;
#1927=FACE_OUTER_BOUND ( 'NONE', #29291, .T. ) ;
#1928=DIRECTION ( 'NONE',  ( -3.018418848199642865E-16, -1.000000000000000000, 0.000000000000000000 ) ) ;
#1931=CARTESIAN_POINT ( 'NONE',  ( 1.645560275461343203, -28.45273235261698019, 5.104056378000016103 ) ) ;
#1935=CARTESIAN_POINT ( 'NONE',  ( -24.43008698341936835, 14.67811372381255630, 5.507121130000014020 ) ) ;
#1937=CARTESIAN_POINT ( 'NONE',  ( 1.186786632755666426, -28.47586096821117252, 4.099089508000003157 ) ) ;
#1940=CARTESIAN_POINT ( 'NONE',  ( -17.83930458849792089, 19.99999999999597478, -1.000005633855494125E-09 ) ) ;
#1946=EDGE_LOOP ( 'NONE', ( #26278, #25673, #20554, #24299 ) ) ;
#1948=CARTESIAN_POINT ( 'NONE',  ( 24.43008698959658176, -14.67811372800087000, 5.507121129000008608 ) ) ;
#1955=CARTESIAN_POINT ( 'NONE',  ( -17.83930458829795640, 19.99999999999961631, -0.6999999999999784173 ) ) ;
#1956=FACE_OUTER_BOUND ( 'NONE', #2093, .T. ) ;
#1960=CARTESIAN_POINT ( 'NONE',  ( -19.00669913905015918, 20.00027147608937028, -0.5056402829912918229 ) ) ;
#1962=EDGE_CURVE ( 'NONE', #4471, #28870, #27131, .T. ) ;
#1976=CARTESIAN_POINT ( 'NONE',  ( 16.06675444873834380, 10.97998838177521286, -0.6999999989999727834 ) ) ;
#1984=CARTESIAN_POINT ( 'NONE',  ( 17.83931306984926835, 20.00000000000176570, -0.6999999999999784173 ) ) ;
#1997=CARTESIAN_POINT ( 'NONE',  ( -23.23955040174346465, -15.25661106733265981, 4.791628272000025390 ) ) ;
#2000=CARTESIAN_POINT ( 'NONE',  ( -0.5821515579339680002, -27.79407096281863687, 4.791896188000022150 ) ) ;
#2013=AXIS2_PLACEMENT_3D ( 'NONE', #490, #2676, #5037 ) ;
#2015=CARTESIAN_POINT ( 'NONE',  ( 27.24406355354254217, 0.4957164003247224726, 0.08279779300002232389 ) ) ;
#2023=EDGE_CURVE ( 'NONE', #2398, #16829, #7123, .T. ) ;
#2032=CARTESIAN_POINT ( 'NONE',  ( -27.07233446963630996, 8.380005019355408535, 3.799999999999998046 ) ) ;
#2035=CARTESIAN_POINT ( 'NONE',  ( -4.667733413579616908, -30.93201666723582122, 1.000000000000000888 ) ) ;
#2039=ORIENTED_EDGE ( 'NONE', *, *, #17060, .F. ) ;
#2044=CARTESIAN_POINT ( 'NONE',  ( 27.47617339892474675, -9.531132158558678569, -0.6577119969999878357 ) ) ;
#2046=CARTESIAN_POINT ( 'NONE',  ( -26.07456367145396214, -11.88770200349126327, 8.000000000000007105 ) ) ;
#2048=CARTESIAN_POINT ( 'NONE',  ( 28.45300238704230367, 0.5177135156027404816, 0.5017677510000262409 ) ) ;
#2052=ORIENTED_EDGE ( 'NONE', *, *, #16040, .T. ) ;
#2065=ORIENTED_EDGE ( 'NONE', *, *, #19134, .T. ) ;
#2067=CARTESIAN_POINT ( 'NONE',  ( 23.25311087529421172, 15.23597699658644800, 4.689445052000001724 ) ) ;
#2070=CARTESIAN_POINT ( 'NONE',  ( 18.62828648731074921, 19.99998815318511092, -0.6147320732107522945 ) ) ;
#2086=CARTESIAN_POINT ( 'NONE',  ( 0.5537481963840298338, -28.49486543565700813, 6.099998581000020792 ) ) ;
#2087=CARTESIAN_POINT ( 'NONE',  ( -17.93324555108848628, -9.020011617866936504, 0.000000000000000000 ) ) ;
#2091=CARTESIAN_POINT ( 'NONE',  ( 18.26639035964474900, 11.02001161816309072, -1.000005633855494125E-09 ) ) ;
#2093=EDGE_LOOP ( 'NONE', ( #29555, #27466, #14678, #7835 ) ) ;
#2095=CARTESIAN_POINT ( 'NONE',  ( 24.38199545065365115, 14.75707034588002564, 3.901343066999990228 ) ) ;
#2097=ORIENTED_EDGE ( 'NONE', *, *, #25278, .F. ) ;
#2099=VERTEX_POINT ( 'NONE', #11390 ) ;
#2100=CARTESIAN_POINT ( 'NONE',  ( 24.93720649360215802, -13.79881813812812297, 6.099998581000020792 ) ) ;
#2140=CARTESIAN_POINT ( 'NONE',  ( 1.311146135404979818, -27.76947565989378219, 4.240358041999986227 ) ) ;
#2141=ORIENTED_EDGE ( 'NONE', *, *, #30800, .T. ) ;
#2144=CARTESIAN_POINT ( 'NONE',  ( -27.63815568848399451, -7.780344951885712845, 0.7069222069999991920 ) ) ;
#2156=CARTESIAN_POINT ( 'NONE',  ( 22.97559295603346285, 15.65128684871516818, 8.000000000000007105 ) ) ;
#2159=CARTESIAN_POINT ( 'NONE',  ( -15.78883365603684474, -9.367159789388974644, 0.000000000000000000 ) ) ;
#2164=DIRECTION ( 'NONE',  ( 0.000000000000000000, 0.000000000000000000, -1.000000000000000000 ) ) ;
#2180=ORIENTED_EDGE ( 'NONE', *, *, #19887, .F. ) ;
#2190=CARTESIAN_POINT ( 'NONE',  ( -19.80535357377644701, 19.50875577052588739, 1.800000043000016259 ) ) ;
#2206=CARTESIAN_POINT ( 'NONE',  ( -24.61381496323305740, -14.36755986783201777, 6.042472825000033687 ) ) ;
#2224=PRESENTATION_STYLE_ASSIGNMENT (( #30702 ) ) ;
#2225=CYLINDRICAL_SURFACE ( 'NONE', #23013, 1.099999999999999867 ) ;
#2227=CARTESIAN_POINT ( 'NONE',  ( 17.83931306984926835, 20.00000000000176570, -0.6999999999999784173 ) ) ;
#2228=CARTESIAN_POINT ( 'NONE',  ( -24.37165444408190851, 14.77472139917419369, 4.999998581000003384 ) ) ;
#2231=CARTESIAN_POINT ( 'NONE',  ( 17.73794748038870139, -9.950927728802978933, -4.336808689942017243E-16 ) ) ;
#2232=ORIENTED_EDGE ( 'NONE', *, *, #3090, .T. ) ;
#2234=EDGE_CURVE ( 'NONE', #29242, #170, #14064, .T. ) ;
#2240=EDGE_CURVE ( 'NONE', #10529, #27389, #10891, .T. ) ;
#2242=CARTESIAN_POINT ( 'NONE',  ( 24.96253706050071131, 13.75225324050492581, 5.310538874999992665 ) ) ;
#2243=CARTESIAN_POINT ( 'NONE',  ( -25.40918998211758861, 12.90916337393047009, 5.498574322615646714 ) ) ;
#2245=CARTESIAN_POINT ( 'NONE',  ( 23.85073401102529900, -14.28298790920352879, 5.558590095350946392 ) ) ;
#2257=VECTOR ( 'NONE', #29780, 1000.000000000000000 ) ;
#2263=ORIENTED_EDGE ( 'NONE', *, *, #25435, .F. ) ;
#2267=ADVANCED_FACE ( 'NONE', ( #12150 ), #16414, .F. ) ;
#2281=CARTESIAN_POINT ( 'NONE',  ( -23.74433668060337155, -14.45919608462527606, 3.899998580999992193 ) ) ;
#2282=CARTESIAN_POINT ( 'NONE',  ( 1.568292632099254291, -27.75603058367145692, 4.689797669000017599 ) ) ;
#2284=CARTESIAN_POINT ( 'NONE',  ( 20.30396079652883756, 20.00000000004620304, 1.000000000000000888 ) ) ;
#2300=CARTESIAN_POINT ( 'NONE',  ( 24.26927060809864400, 14.94229634074801361, 6.073751781078700951 ) ) ;
#2301=CARTESIAN_POINT ( 'NONE',  ( 23.81866167241657806, 14.33570040768432996, 6.099998581000020792 ) ) ;
#2303=EDGE_CURVE ( 'NONE', #25231, #6269, #9777, .T. ) ;
#2308=CARTESIAN_POINT ( 'NONE',  ( 17.33115445884845229, -10.09718743895510151, -0.6999999999999783062 ) ) ;
#2314=CARTESIAN_POINT ( 'NONE',  ( 22.97695743748386832, 16.89262754991261062, 7.000000000000006217 ) ) ;
#2323=CARTESIAN_POINT ( 'NONE',  ( -24.54884434681240890, 13.04717673402245914, 3.997190761000024573 ) ) ;
#2327=CARTESIAN_POINT ( 'NONE',  ( 17.70481771267368032, -8.030294603601026537, -0.6999999999999785283 ) ) ;
#2337=CARTESIAN_POINT ( 'NONE',  ( -15.73360964030186970, 11.02001161816959396, -0.6999999999999784173 ) ) ;
#2345=CARTESIAN_POINT ( 'NONE',  ( 23.47715715134837211, -20.00370206646827498, 1.000000000000000888 ) ) ;
#2346=CARTESIAN_POINT ( 'NONE',  ( -20.30403093128963476, 20.00000000003735323, 2.200000064000007249 ) ) ;
#2374=EDGE_CURVE ( 'NONE', #10752, #5681, #11247, .T. ) ;
#2376=CARTESIAN_POINT ( 'NONE',  ( -17.28486482095781085, -10.01258675972073675, 0.000000000000000000 ) ) ;
#2383=CARTESIAN_POINT ( 'NONE',  ( 19.19680082505102447, 20.00027389960937185, -0.4288677566865453650 ) ) ;
#2384=FACE_OUTER_BOUND ( 'NONE', #17339, .T. ) ;
#2398=VERTEX_POINT ( 'NONE', #7588 ) ;
#2402=B_SPLINE_CURVE_WITH_KNOTS ( 'NONE', 3,
 ( #12371, #5441, #19925, #5297, #24950, #17240 ),
 .UNSPECIFIED., .F., .F.,
 ( 4, 2, 4 ),
 ( 0.000000000000000000, 0.5000000000000000000, 1.000000000000000000 ),
 .UNSPECIFIED. ) ;
#2416=ORIENTED_EDGE ( 'NONE', *, *, #3677, .T. ) ;
#2423=CARTESIAN_POINT ( 'NONE',  ( -18.82786841510930742, 20.00005837762122241, -0.5634673906915752539 ) ) ;
#2428=CARTESIAN_POINT ( 'NONE',  ( 16.40303402075260308, 10.20816091466531716, -0.6999999999999784173 ) ) ;
#2448=EDGE_LOOP ( 'NONE', ( #6764, #479, #13207, #29754 ) ) ;
#2449=CARTESIAN_POINT ( 'NONE',  ( 23.81776757409229361, 15.65134803726813217, 4.999998581000003384 ) ) ;
#2471=CARTESIAN_POINT ( 'NONE',  ( -25.12046394328327281, 13.46291001840482160, 3.957489296000010981 ) ) ;
#2475=B_SPLINE_SURFACE_WITH_KNOTS ( 'NONE', 5, 1, ( 
 ( #9573, #21220 ),
 ( #30821, #28297 ),
 ( #2345, #18314 ),
 ( #11929, #26413 ),
 ( #2035, #24056 ),
 ( #14145, #23445 ),
 ( #19171, #18858 ),
 ( #16342, #4387 ),
 ( #30976, #23910 ) ),
 .UNSPECIFIED., .F., .F., .F.,
 ( 6, 3, 6 ),
 ( 2, 2 ),
 ( 0.000000000000000000, 53.95537973340000093, 92.42745556099998794 ),
 ( -3.500000000000000000, 3.500000000000000000 ),
 .UNSPECIFIED. ) ;
#2477=CARTESIAN_POINT ( 'NONE',  ( 17.82602571118884427, -8.107840965023857649, -0.6999999999999783062 ) ) ;
#2478=CYLINDRICAL_SURFACE ( 'NONE', #7762, 1.100000000000002309 ) ;
#2494=FACE_BOUND ( 'NONE', #9502, .T. ) ;
#2505=CARTESIAN_POINT ( 'NONE',  ( 24.63375101535647360, -12.88633855010671247, 5.901400366999986602 ) ) ;
#2508=CARTESIAN_POINT ( 'NONE',  ( -20.28771362240119913, 20.00000013994726089, 0.7458731309999966363 ) ) ;
#2514=ORIENTED_EDGE ( 'NONE', *, *, #22485, .F. ) ;
#2520=CARTESIAN_POINT ( 'NONE',  ( 24.95427444975690889, -13.76797447160702070, 3.899998581000013509 ) ) ;
#2528=CARTESIAN_POINT ( 'NONE',  ( -4.667733413579616908, -30.93201666723582122, 1.000000000000000888 ) ) ;
#2533=CARTESIAN_POINT ( 'NONE',  ( -24.90302310912370132, 13.86047864606265279, 6.098655051000018368 ) ) ;
#2548=CARTESIAN_POINT ( 'NONE',  ( -23.87170005649112525, -14.24726900567271493, 3.904031772999999816 ) ) ;
#2549=CARTESIAN_POINT ( 'NONE',  ( 16.19548821459394716, 11.53640331831526744, -4.336808689942018722E-16 ) ) ;
#2550=ORIENTED_EDGE ( 'NONE', *, *, #5836, .T. ) ;
#2552=CARTESIAN_POINT ( 'NONE',  ( 17.93011078765611543, -8.208160914697428368, -0.6999999999999784173 ) ) ;
#2559=ORIENTED_EDGE ( 'NONE', *, *, #5934, .F. ) ;
#2566=CARTESIAN_POINT ( 'NONE',  ( -24.83827471527357744, 12.48687850854618198, 4.999998581000003384 ) ) ;
#2575=CARTESIAN_POINT ( 'NONE',  ( 18.05873143933198577, -9.659453306092730784, -0.6999999999999783062 ) ) ;
#2581=CARTESIAN_POINT ( 'NONE',  ( 27.51421515662130446, 9.168494879182089718, 1.000000000000000888 ) ) ;
#2591=ORIENTED_EDGE ( 'NONE', *, *, #25415, .T. ) ;
#2592=CARTESIAN_POINT ( 'NONE',  ( 17.83929014045347827, 20.00000000006149392, -1.000005633855494125E-09 ) ) ;
#2594=VERTEX_POINT ( 'NONE', #5140 ) ;
#2603=CARTESIAN_POINT ( 'NONE',  ( 17.18658402241074867, -10.09981795543446736, -0.6999999999999784173 ) ) ;
#2617=CARTESIAN_POINT ( 'NONE',  ( 24.06826093652101051, -20.50742065841456707, 0.7595836940000044724 ) ) ;
#2623=CARTESIAN_POINT ( 'NONE',  ( -16.37013654256265482, -7.994344025985067326, 0.000000000000000000 ) ) ;
#2627=CARTESIAN_POINT ( 'NONE',  ( 0.000000000000000000, 0.000000000000000000, 0.000000000000000000 ) ) ;
#2640=CARTESIAN_POINT ( 'NONE',  ( -24.37821945910799926, 14.76389285725497125, 4.791564337000009388 ) ) ;
#2649=FACE_OUTER_BOUND ( 'NONE', #5464, .T. ) ;
#2655=B_SPLINE_SURFACE_WITH_KNOTS ( 'NONE', 5, 1, ( 
 ( #19492, #26719 ),
 ( #30830, #18866 ),
 ( #28463, #26112 ),
 ( #6899, #16501 ),
 ( #4550, #14152 ),
 ( #30984, #3107 ),
 ( #17272, #7826 ),
 ( #24367, #29849 ),
 ( #29699, #17878 ) ),
 .UNSPECIFIED., .F., .F., .F.,
 ( 6, 3, 6 ),
 ( 2, 2 ),
 ( 72.29952875009999502, 84.34563975540000058, 88.66903727190000950 ),
 ( -3.307798128770000356E-15, 0.7016521142910000508 ),
 .UNSPECIFIED. ) ;
#2657=CARTESIAN_POINT ( 'NONE',  ( -15.88249986683283232, 11.57137507597117754, -4.336808689942017243E-16 ) ) ;
#2659=CARTESIAN_POINT ( 'NONE',  ( -24.49145440957854802, 14.57548795260905550, 5.680829343999993952 ) ) ;
#2661=B_SPLINE_CURVE_WITH_KNOTS ( 'NONE', 3,
 ( #25590, #4025, #20545, #29978, #4340, #23395, #13622, #13459, #18173, #27774 ),
 .UNSPECIFIED., .F., .F.,
 ( 4, 2, 2, 2, 4 ),
 ( 0.000000000000000000, 0.2500000000000000000, 0.5000000000000000000, 0.7500000000000000000, 1.000000000000000000 ),
 .UNSPECIFIED. ) ;
#2676=DIRECTION ( 'NONE',  ( 0.000000000000000000, 0.000000000000000000, -1.000000000000000000 ) ) ;
#2681=CARTESIAN_POINT ( 'NONE',  ( 18.79419193508953967, 19.99998513589524407, -0.5771770174943486875 ) ) ;
#2682=CARTESIAN_POINT ( 'NONE',  ( -24.92013865347427171, 13.82966157970119525, 6.099998581000020792 ) ) ;
#2687=CARTESIAN_POINT ( 'NONE',  ( 3.350725639037565706, -1.107490566386527986, 0.000000000000000000 ) ) ;
#2688=FACE_OUTER_BOUND ( 'NONE', #11071, .T. ) ;
#2690=CARTESIAN_POINT ( 'NONE',  ( 24.75645985066559263, 14.12045945726143970, 5.901294549000013490 ) ) ;
#2702=CARTESIAN_POINT ( 'NONE',  ( 1.607747500013188446, -28.45491842328731025, 4.689797669000017599 ) ) ;
#2703=CARTESIAN_POINT ( 'NONE',  ( 16.85920661257417663, 12.06595463936088208, -4.336808689942018722E-16 ) ) ;
#2704=VERTEX_POINT ( 'NONE', #2337 ) ;
#2706=CARTESIAN_POINT ( 'NONE',  ( -16.14314806408744118, 10.13116291470765162, -0.6999999999999784173 ) ) ;
#2709=VERTEX_POINT ( 'NONE', #21528 ) ;
#2730=CARTESIAN_POINT ( 'NONE',  ( 18.13627780309760595, -9.538245302789915669, -0.6999999999999785283 ) ) ;
#2732=COLOUR_RGB ( '', 0.09019608, 0.27058824, 0.51372549) ;
#2735=CARTESIAN_POINT ( 'NONE',  ( -24.32472894358752313, 13.45989150749028873, 3.899998581000013509 ) ) ;
#2746=CARTESIAN_POINT ( 'NONE',  ( -27.17362711782706342, 4.180443856937215763, 0.02487529600000981667 ) ) ;
#2750=SHAPE_REPRESENTATION_RELATIONSHIP ( 'NONE' , 'NONE' ,  #3523, #18548 ) ;
#2759=ADVANCED_FACE ( 'NONE', ( #1053 ), #7242, .T. ) ;
#2760=B_SPLINE_SURFACE_WITH_KNOTS ( 'NONE', 5, 1, ( 
 ( #19820, #9748 ),
 ( #19355, #16830 ),
 ( #14939, #5028 ),
 ( #11955, #24539 ),
 ( #7684, #29403 ),
 ( #28946, #21564 ),
 ( #10217, #17441 ),
 ( #13, #22031 ),
 ( #19661, #7542 ),
 ( #29245, #26735 ),
 ( #326, #16984 ),
 ( #17133, #9907 ),
 ( #9596, #2978 ),
 ( #2520, #7838 ),
 ( #4877, #19195 ) ),
 .UNSPECIFIED., .F., .F., .F.,
 ( 6, 3, 3, 3, 6 ),
 ( 2, 2 ),
 ( 0.000000000000000000, 0.5239049114710000454, 1.047809822950000136, 1.571714734409999981, 1.746349704900000077 ),
 ( -0.7000000000009999335, 2.557517314480000010E-06 ),
 .UNSPECIFIED. ) ;
#2766=CARTESIAN_POINT ( 'NONE',  ( 17.18658402241074867, -10.09981795543446736, -1.000005633855494125E-09 ) ) ;
#2773=CARTESIAN_POINT ( 'NONE',  ( -24.36725163763869162, -13.38201776504303986, 4.999998581000003384 ) ) ;
#2776=CARTESIAN_POINT ( 'NONE',  ( -17.15915740090245123, -7.941754552259828515, 0.000000000000000000 ) ) ;
#2777=CARTESIAN_POINT ( 'NONE',  ( -28.31737690039761901, -7.971550764210702411, 0.5017677510000262409 ) ) ;
#2781=CARTESIAN_POINT ( 'NONE',  ( -24.95427444319612675, 13.76797446832583560, 3.899998581000013509 ) ) ;
#2806=CARTESIAN_POINT ( 'NONE',  ( -24.41841039498785193, -14.69667350221323865, 3.899998581000013509 ) ) ;
#2808=CARTESIAN_POINT ( 'NONE',  ( 17.95841148951064525, -9.763538383420391042, 0.000000000000000000 ) ) ;
#2811=CARTESIAN_POINT ( 'NONE',  ( -16.01948174858000229, -8.256768211624056164, 0.000000000000000000 ) ) ;
#2830=CARTESIAN_POINT ( 'NONE',  ( -16.83342759582943060, -8.999999999996580513, -0.6999999999999784173 ) ) ;
#2834=CARTESIAN_POINT ( 'NONE',  ( -24.43008698341936835, 14.67811372381255630, 5.507121130000014020 ) ) ;
#2841=B_SPLINE_CURVE_WITH_KNOTS ( 'NONE', 5,
 ( #7349, #4526, #4984, #24183, #9387, #2623, #18991, #12802, #28597, #26235, #282, #14283 ),
 .UNSPECIFIED., .F., .F.,
 ( 6, 3, 3, 6 ),
 ( 1.224410041430000096, 1.456395031030000009, 2.184590861730000277, 2.448622038789999955 ),
 .UNSPECIFIED. ) ;
#2842=CARTESIAN_POINT ( 'NONE',  ( 24.37821946547973084, -14.76389286113969490, 5.208432824000020389 ) ) ;
#2843=EDGE_CURVE ( 'NONE', #21789, #11577, #18355, .T. ) ;
#2848=ADVANCED_FACE ( 'NONE', ( #20362 ), #16778, .F. ) ;
#2851=CARTESIAN_POINT ( 'NONE',  ( -24.97472003774791816, -13.73006752753317450, 4.791638085000021974 ) ) ;
#2853=ORIENTED_EDGE ( 'NONE', *, *, #9275, .T. ) ;
#2863=EDGE_LOOP ( 'NONE', ( #28361, #29445, #9175, #18503 ) ) ;
#2870=CARTESIAN_POINT ( 'NONE',  ( -25.25401215124432852, 13.21081861195569296, 5.901400367999992902 ) ) ;
#2872=CARTESIAN_POINT ( 'NONE',  ( 28.49528339128749366, 0.5184828350247233653, 1.000000000000000888 ) ) ;
#2885=CARTESIAN_POINT ( 'NONE',  ( -16.83342759575507586, 10.99999999997565503, -0.6999999999999784173 ) ) ;
#2894=CARTESIAN_POINT ( 'NONE',  ( -22.04938731152978448, 17.55153357857029306, 0.7069229489999884208 ) ) ;
#2896=ORIENTED_EDGE ( 'NONE', *, *, #3349, .F. ) ;
#2904=ORIENTED_EDGE ( 'NONE', *, *, #10367, .T. ) ;
#2921=DIRECTION ( 'NONE',  ( 0.000000000000000000, 0.000000000000000000, -1.000000000000000000 ) ) ;
#2926=CARTESIAN_POINT ( 'NONE',  ( -24.69211139838770208, -14.75429553128187798, -0.6577119969999878357 ) ) ;
#2928=CARTESIAN_POINT ( 'NONE',  ( 24.37821946547973084, -14.76389286113969490, 4.791564337000009388 ) ) ;
#2947=CARTESIAN_POINT ( 'NONE',  ( -24.20792486932886689, 13.66932879934886813, 3.920132063000014710 ) ) ;
#2951=CARTESIAN_POINT ( 'NONE',  ( 24.44014313072642963, -13.24968496497942105, 6.079865069000017996 ) ) ;
#2956=CARTESIAN_POINT ( 'NONE',  ( 24.45473033137484720, 14.63622297804190175, 3.901342939999996595 ) ) ;
#2978=CARTESIAN_POINT ( 'NONE',  ( 24.35797964201644561, -13.39969403546014703, 3.901342130000013064 ) ) ;
#2987=CARTESIAN_POINT ( 'NONE',  ( 24.36724935763797006, 13.38201651305720574, 4.999998581000003384 ) ) ;
#2988=CARTESIAN_POINT ( 'NONE',  ( 19.80526555962148549, 19.50877392102342256, 1.000000000000000888 ) ) ;
#3000=CARTESIAN_POINT ( 'NONE',  ( 19.76603533419210734, 19.51852340513930173, 0.7754612589999931860 ) ) ;
#3007=EDGE_LOOP ( 'NONE', ( #29827, #3088, #16719, #9279 ) ) ;
#3010=ORIENTED_EDGE ( 'NONE', *, *, #30863, .T. ) ;
#3011=CARTESIAN_POINT ( 'NONE',  ( 28.43512364494067413, 3.824800618850225931, 8.000000000000007105 ) ) ;
#3019=CARTESIAN_POINT ( 'NONE',  ( -16.56625540809453057, 12.07698932566918160, -0.6999999999999784173 ) ) ;
#3023=CARTESIAN_POINT ( 'NONE',  ( -24.44014312407112399, 13.24968496200000523, 6.079865069000017996 ) ) ;
#3025=CARTESIAN_POINT ( 'NONE',  ( 0.4125558677674681096, -28.49726274111934998, 6.095949245000009675 ) ) ;
#3040=ORIENTED_EDGE ( 'NONE', *, *, #20095, .F. ) ;
#3045=CARTESIAN_POINT ( 'NONE',  ( -18.03439342504434606, 20.21871256385842841, 0.02487531600001147147 ) ) ;
#3051=CARTESIAN_POINT ( 'NONE',  ( -24.37165444408190851, 14.77472139917419369, 4.999998581000003384 ) ) ;
#3056=CARTESIAN_POINT ( 'NONE',  ( -28.45300238704230367, -0.5177135156027357077, 0.5017677510000262409 ) ) ;
#3060=CARTESIAN_POINT ( 'NONE',  ( -27.79539923781770483, -0.5057481688778011630, 1.000000000000000888 ) ) ;
#3073=CARTESIAN_POINT ( 'NONE',  ( -27.42665334337451455, -7.720805503521760649, -0.5592437529999827461 ) ) ;
#3088=ORIENTED_EDGE ( 'NONE', *, *, #24827, .T. ) ;
#3089=CARTESIAN_POINT ( 'NONE',  ( 23.40723432809949855, -19.94412562524615140, 0.5514312830000311916 ) ) ;
#3090=EDGE_CURVE ( 'NONE', #18763, #3434, #12155, .T. ) ;
#3091=ORIENTED_EDGE ( 'NONE', *, *, #11250, .T. ) ;
#3093=CARTESIAN_POINT ( 'NONE',  ( 17.00199035030329497, 12.09718743885649950, -0.6999999999999783062 ) ) ;
#3099=CARTESIAN_POINT ( 'NONE',  ( 24.82162974202869421, -12.51998933900577349, 5.310645680000003921 ) ) ;
#3100=CARTESIAN_POINT ( 'NONE',  ( -16.83342759575507586, 10.99999999997565503, -0.6999999999999784173 ) ) ;
#3104=CARTESIAN_POINT ( 'NONE',  ( -24.92639508767336309, -13.81781708088548122, 4.493023692000025271 ) ) ;
#3107=CARTESIAN_POINT ( 'NONE',  ( 27.65104940643587383, 3.057637721010480814, 8.000000000000007105 ) ) ;
#3108=CARTESIAN_POINT ( 'NONE',  ( -0.6094664100040195764, -28.49364619262437870, 4.999998581000003384 ) ) ;
#3116=VECTOR ( 'NONE', #15262, 1000.000000000000000 ) ;
#3131=CARTESIAN_POINT ( 'NONE',  ( 16.09014176772306826, -8.731615745635396664, -4.336808689942017243E-16 ) ) ;
#3132=CARTESIAN_POINT ( 'NONE',  ( 24.86822223037987456, 13.92223202030449691, 4.319317656000021266 ) ) ;
#3142=CARTESIAN_POINT ( 'NONE',  ( -21.81271764029508731, 17.27884132338922285, 6.000000042999998229 ) ) ;
#3146=CARTESIAN_POINT ( 'NONE',  ( 24.32472894995379420, -13.45989151107506387, 6.099998581000020792 ) ) ;
#3148=FACE_OUTER_BOUND ( 'NONE', #1111, .T. ) ;
#3150=B_SPLINE_CURVE_WITH_KNOTS ( 'NONE', 3,
 ( #8507, #10890, #30082, #13559, #6001, #15915, #27875, #25370, #20639, #15600, #25051, #28026 ),
 .UNSPECIFIED., .F., .F.,
 ( 4, 2, 2, 2, 2, 4 ),
 ( 0.000000000000000000, 0.1250000000000004441, 0.2500000000000008882, 0.5000000000000005551, 0.7500000000000003331, 1.000000000000000000 ),
 .UNSPECIFIED. ) ;
#3153=CARTESIAN_POINT ( 'NONE',  ( 23.80322556508107112, 14.59355840047072661, 1.000000000000000888 ) ) ;
#3169=DIRECTION ( 'NONE',  ( -1.000000000000000000, -8.816454510895967384E-12, 0.000000000000000000 ) ) ;
#3173=CARTESIAN_POINT ( 'NONE',  ( 25.77914806503467560, 15.40383291000323318, 1.000000000000000888 ) ) ;
#3179=VECTOR ( 'NONE', #11020, 1000.000000000000000 ) ;
#3195=B_SPLINE_CURVE_WITH_KNOTS ( 'NONE', 1,
 ( #25574, #11405 ),
 .UNSPECIFIED., .F., .F.,
 ( 2, 2 ),
 ( -2.557517314480000010E-06, 0.7000000000009999335 ),
 .UNSPECIFIED. ) ;
#3196=CARTESIAN_POINT ( 'NONE',  ( -22.00340350502675690, 17.51493346882343261, 0.5514279790000131687 ) ) ;
#3211=CARTESIAN_POINT ( 'NONE',  ( -26.70575606321611062, 9.025857534248860503, -0.5592437529999827461 ) ) ;
#3218=VERTEX_POINT ( 'NONE', #27404 ) ;
#3220=CARTESIAN_POINT ( 'NONE',  ( -24.86822223968197321, -13.92223202027371975, 5.680679499000030219 ) ) ;
#3223=CARTESIAN_POINT ( 'NONE',  ( -23.57322167415998138, -14.73624932338542060, 6.002747143000003227 ) ) ;
#3229=CARTESIAN_POINT ( 'NONE',  ( -24.24144457387483698, -14.48500828217274439, -0.6999999999999784173 ) ) ;
#3231=CARTESIAN_POINT ( 'NONE',  ( 23.81866167241657806, 14.33570040768432996, 6.099998581000020792 ) ) ;
#3232=EDGE_CURVE ( 'NONE', #12806, #10592, #10253, .T. ) ;
#3242=AXIS2_PLACEMENT_3D ( 'NONE', #13971, #16166, #14125 ) ;
#3246=CARTESIAN_POINT ( 'NONE',  ( -19.86374233096328012, -20.73196311662712077, 0.08279834900001836751 ) ) ;
#3247=ORIENTED_EDGE ( 'NONE', *, *, #11490, .F. ) ;
#3254=CARTESIAN_POINT ( 'NONE',  ( 24.37450210455010335, -13.36961646745188759, 6.095967861000000987 ) ) ;
#3257=ORIENTED_EDGE ( 'NONE', *, *, #27456, .F. ) ;
#3271=ADVANCED_FACE ( 'NONE', ( #535, #1130 ), #26340, .F. ) ;
#3273=ORIENTED_EDGE ( 'NONE', *, *, #22485, .T. ) ;
#3285=CARTESIAN_POINT ( 'NONE',  ( 16.06675444876397307, -9.020011618195203695, -1.000005633855494125E-09 ) ) ;
#3286=CARTESIAN_POINT ( 'NONE',  ( 24.22405392119105016, 13.63981656816893739, 4.239871879999995485 ) ) ;
#3307=EDGE_CURVE ( 'NONE', #18124, #11650, #30139, .T. ) ;
#3310=CARTESIAN_POINT ( 'NONE',  ( 23.23955039760055641, 15.25661106415676471, 5.208368893000026034 ) ) ;
#3321=CARTESIAN_POINT ( 'NONE',  ( -17.10181184887932915, 9.923569363214987504, -0.6999999999999785283 ) ) ;
#3325=CARTESIAN_POINT ( 'NONE',  ( -24.50348397099046593, 13.13223627435659857, 6.042507865999996675 ) ) ;
#3329=EDGE_LOOP ( 'NONE', ( #23056, #9288, #9756, #21374 ) ) ;
#3332=CARTESIAN_POINT ( 'NONE',  ( -17.80313298963281099, -8.461754685791088804, -0.6999999999999785283 ) ) ;
#3333=CARTESIAN_POINT ( 'NONE',  ( 24.15903335124918527, 13.75473836089376434, 5.881930534969080249 ) ) ;
#3341=EDGE_CURVE ( 'NONE', #3626, #3424, #23423, .T. ) ;
#3344=CARTESIAN_POINT ( 'NONE',  ( 23.82458380820737531, 13.44211522811278314, 0.000000000000000000 ) ) ;
#3347=CARTESIAN_POINT ( 'NONE',  ( -26.93580492059415121, 9.103810007694223216, 0.8585786479999857335 ) ) ;
#3349=EDGE_CURVE ( 'NONE', #11650, #24241, #8732, .T. ) ;
#3350=ORIENTED_EDGE ( 'NONE', *, *, #26240, .T. ) ;
#3360=CARTESIAN_POINT ( 'NONE',  ( -26.79556473285982321, -0.4875557887250224209, -0.6999999999999784173 ) ) ;
#3365=EDGE_LOOP ( 'NONE', ( #23151, #1317, #5964, #18332 ) ) ;
#3372=CARTESIAN_POINT ( 'NONE',  ( -23.81866173682177390, -14.33570044646243247, 6.099998581000020792 ) ) ;
#3373=CARTESIAN_POINT ( 'NONE',  ( -24.21906834513991313, -15.02342241408235068, 6.042470790000031400 ) ) ;
#3377=CARTESIAN_POINT ( 'NONE',  ( -16.85343921422224156, -7.900182044607009679, 0.000000000000000000 ) ) ;
#3378=CARTESIAN_POINT ( 'NONE',  ( -23.80092421055088892, -14.36517094966330710, 6.099998581000020792 ) ) ;
#3386=CARTESIAN_POINT ( 'NONE',  ( 0.2655682516138271887, -27.79918151443131791, 6.079792140000011891 ) ) ;
#3387=EDGE_LOOP ( 'NONE', ( #2559, #25724, #23401, #3625, #5181 ) ) ;
#3397=CARTESIAN_POINT ( 'NONE',  ( 27.08859402333790101, 0.4928875713652628443, 0.02487529600000981667 ) ) ;
#3404=CARTESIAN_POINT ( 'NONE',  ( -24.16205483806062304, 15.15351638958479086, 8.000000000000007105 ) ) ;
#3406=CARTESIAN_POINT ( 'NONE',  ( 25.44662323365202639, -12.83524168329857318, 5.310645680000003921 ) ) ;
#3424=VERTEX_POINT ( 'NONE', #9450 ) ;
#3427=ORIENTED_EDGE ( 'NONE', *, *, #16208, .F. ) ;
#3434=VERTEX_POINT ( 'NONE', #23785 ) ;
#3444=CARTESIAN_POINT ( 'NONE',  ( -18.52981556209221381, 19.99998962372823996, -0.6359626486881121421 ) ) ;
#3451=CARTESIAN_POINT ( 'NONE',  ( -4.785279987099964494, -31.71089578132184883, 8.000000000000007105 ) ) ;
#3459=EDGE_CURVE ( 'NONE', #4259, #25869, #27510, .T. ) ;
#3479=B_SPLINE_CURVE_WITH_KNOTS ( 'NONE', 5,
 ( #19332, #24516, #14763, #12696, #7663, #16960, #19943, #22153, #21695 ),
 .UNSPECIFIED., .F., .F.,
 ( 6, 3, 6 ),
 ( 0.000000000000000000, 53.95537973340000093, 92.42745556099998794 ),
 .UNSPECIFIED. ) ;
#3480=CARTESIAN_POINT ( 'NONE',  ( -28.49528339128749366, -0.5184828350247786544, 8.000000000000007105 ) ) ;
#3504=CARTESIAN_POINT ( 'NONE',  ( -26.66783967069105898, -7.507193849635574345, -0.6999999999999784173 ) ) ;
#3506=ORIENTED_EDGE ( 'NONE', *, *, #17090, .T. ) ;
#3514=CARTESIAN_POINT ( 'NONE',  ( 1.199983934731101209, -28.47518316922301196, 5.888828386639105794 ) ) ;
#3516=CARTESIAN_POINT ( 'NONE',  ( -27.61404081990094994, 9.332834367751024374, 1.000000000000000888 ) ) ;
#3523=SHAPE_REPRESENTATION ( 'Rear Frame Plate', ( #17722 ), #16292 ) ;
#3533=FACE_OUTER_BOUND ( 'NONE', #23808, .T. ) ;
#3537=CYLINDRICAL_SURFACE ( 'NONE', #29338, 1.100000000000002309 ) ;
#3554=ORIENTED_EDGE ( 'NONE', *, *, #26182, .T. ) ;
#3566=CARTESIAN_POINT ( 'NONE',  ( -28.68577477009351995, 9.950727454193893706, 8.000000000000007105 ) ) ;
#3579=CARTESIAN_POINT ( 'NONE',  ( 18.24300304086109747, -9.268384253839881737, -4.336808689942017243E-16 ) ) ;
#3590=ORIENTED_EDGE ( 'NONE', *, *, #805, .F. ) ;
#3591=CARTESIAN_POINT ( 'NONE',  ( -17.70061747236281491, 10.30810785442435495, -0.6999999999999783062 ) ) ;
#3599=CARTESIAN_POINT ( 'NONE',  ( 25.40918998824096420, -12.90916337733692920, 5.498574324082793119 ) ) ;
#3603=LINE ( 'NONE', #29582, #30262 ) ;
#3605=CARTESIAN_POINT ( 'NONE',  ( 28.49528339128749366, 0.5184828350247823181, 8.000000000000007105 ) ) ;
#3610=CARTESIAN_POINT ( 'NONE',  ( 21.73669719418043300, 17.54549339080899273, -0.5592437529999827461 ) ) ;
#3613=EDGE_LOOP ( 'NONE', ( #6859, #10343, #6323, #8305 ) ) ;
#3616=CARTESIAN_POINT ( 'NONE',  ( 24.06750537016302971, 15.26514225575640360, 5.901296968999991677 ) ) ;
#3622=LINE ( 'NONE', #12921, #23058 ) ;
#3625=ORIENTED_EDGE ( 'NONE', *, *, #23068, .T. ) ;
#3626=VERTEX_POINT ( 'NONE', #8787 ) ;
#3642=CARTESIAN_POINT ( 'NONE',  ( 24.10026512741646698, 13.85771999287294598, 5.960845917926949511 ) ) ;
#3645=CARTESIAN_POINT ( 'NONE',  ( -28.57800709146147256, 4.027926662255243428, 1.000000000000000888 ) ) ;
#3662=CARTESIAN_POINT ( 'NONE',  ( -16.04158851053540857, -9.763538383445707680, -0.6999999999999784173 ) ) ;
#3677=EDGE_CURVE ( 'NONE', #15540, #27013, #17374, .T. ) ;
#3690=CARTESIAN_POINT ( 'NONE',  ( 21.71205242481305930, 17.52560354592457870, 0.2686741030000217023 ) ) ;
#3702=CARTESIAN_POINT ( 'NONE',  ( 24.96433005672375316, 10.36502315879739022, -0.6999999999999784173 ) ) ;
#3709=VERTEX_POINT ( 'NONE', #11623 ) ;
#3712=CARTESIAN_POINT ( 'NONE',  ( -4.667733413672338294, -30.93201666653739323, 0.8585780189999947520 ) ) ;
#3716=CARTESIAN_POINT ( 'NONE',  ( -23.23277126416379801, -15.26692729116844482, 4.999998581000003384 ) ) ;
#3734=CARTESIAN_POINT ( 'NONE',  ( 27.79539923781684507, 0.5057481689249130330, 1.000000000000000888 ) ) ;
#3751=ADVANCED_FACE ( 'NONE', ( #25950, #21384, #14457, #13833 ), #2475, .T. ) ;
#3760=CARTESIAN_POINT ( 'NONE',  ( 28.49528339128749366, 0.5184828350247212558, 1.000000000000000888 ) ) ;
#3761=CARTESIAN_POINT ( 'NONE',  ( -0.5653960855887967263, -27.79447351536211741, 5.289252711543936947 ) ) ;
#3773=CARTESIAN_POINT ( 'NONE',  ( -16.04158851053540857, -9.763538383445707680, -0.6999999999999784173 ) ) ;
#3774=CARTESIAN_POINT ( 'NONE',  ( 18.15349680648220954, 19.92137135063213549, 0.007031429000020628095 ) ) ;
#3779=B_SPLINE_CURVE_WITH_KNOTS ( 'NONE', 1,
 ( #10412, #22530 ),
 .UNSPECIFIED., .F., .F.,
 ( 2, 2 ),
 ( -2.555897717360000054E-06, 0.7000000000009999335 ),
 .UNSPECIFIED. ) ;
#3780=CARTESIAN_POINT ( 'NONE',  ( 23.82458380820737531, 13.44211522811278314, -0.6999999999999784173 ) ) ;
#3781=CARTESIAN_POINT ( 'NONE',  ( 17.95841148948556310, 10.23646161652002817, -0.6999999989999727834 ) ) ;
#3785=FACE_OUTER_BOUND ( 'NONE', #14012, .T. ) ;
#3808=EDGE_CURVE ( 'NONE', #7280, #9797, #18494, .T. ) ;
#3809=VERTEX_POINT ( 'NONE', #26105 ) ;
#3817=CARTESIAN_POINT ( 'NONE',  ( 17.85685193732696519, 10.13116291529594371, -0.6999999999999784173 ) ) ;
#3820=CARTESIAN_POINT ( 'NONE',  ( -17.89998469250338431, 10.69382497388279063, -0.000000000000000000 ) ) ;
#3833=ORIENTED_EDGE ( 'NONE', *, *, #13547, .T. ) ;
#3847=CARTESIAN_POINT ( 'NONE',  ( -25.46368746804859740, 12.80129684245613575, 4.999998581000003384 ) ) ;
#3853=CARTESIAN_POINT ( 'NONE',  ( -24.29089620838935204, -14.90695587844356673, 6.079851352000009257 ) ) ;
#3854=EDGE_CURVE ( 'NONE', #14604, #25327, #26740, .T. ) ;
#3856=CARTESIAN_POINT ( 'NONE',  ( 16.37473331892315542, -8.236461616552139375, -0.6999999989999727834 ) ) ;
#3857=CARTESIAN_POINT ( 'NONE',  ( -17.57665938409742523, -8.186054152995293265, 0.000000000000000000 ) ) ;
#3874=DIRECTION ( 'NONE',  ( 0.000000000000000000, 0.000000000000000000, -1.000000000000000000 ) ) ;
#3879=CARTESIAN_POINT ( 'NONE',  ( 16.06413493411159976, -8.876045783929967570, -4.336808689942017736E-16 ) ) ;
#3881=DIRECTION ( 'NONE',  ( 0.000000000000000000, 0.000000000000000000, -1.000000000000000000 ) ) ;
#3883=CARTESIAN_POINT ( 'NONE',  ( 0.1319790757220171973, -27.80015609199433158, 3.957670871000018575 ) ) ;
#3887=ORIENTED_EDGE ( 'NONE', *, *, #1625, .T. ) ;
#3888=CARTESIAN_POINT ( 'NONE',  ( 20.77600629922060449, 21.68409807857484140, 1.000000000000000888 ) ) ;
#3892=CARTESIAN_POINT ( 'NONE',  ( -17.93392337644938905, -8.982759033125498505, 0.000000000000000000 ) ) ;
#3896=CARTESIAN_POINT ( 'NONE',  ( 22.63260994176697238, -19.28417101125922883, 0.000000000000000000 ) ) ;
#3934=CARTESIAN_POINT ( 'NONE',  ( 22.55330502899744616, -17.67890025412993182, 8.000000000000007105 ) ) ;
#3940=ORIENTED_EDGE ( 'NONE', *, *, #14083, .F. ) ;
#4011=CARTESIAN_POINT ( 'NONE',  ( 27.62942886422533917, 5.076074465521874579, 0.5514269430000329208 ) ) ;
#4021=B_SPLINE_CURVE_WITH_KNOTS ( 'NONE', 5,
 ( #3060, #12656, #19907, #573, #26524, #417 ),
 .UNSPECIFIED., .F., .F.,
 ( 6, 6 ),
 ( 0.000000000000000000, 22.42544452799999988 ),
 .UNSPECIFIED. ) ;
#4025=CARTESIAN_POINT ( 'NONE',  ( -24.25455085227292784, 13.58673930470784796, 6.099998580999935527 ) ) ;
#4031=CARTESIAN_POINT ( 'NONE',  ( 24.46020335245677657, -13.21278628519231546, 3.926747916559686136 ) ) ;
#4033=CARTESIAN_POINT ( 'NONE',  ( -27.52676963214412353, -0.5008603480660347440, 0.2686740700000300741 ) ) ;
#4038=CARTESIAN_POINT ( 'NONE',  ( -3.040504021322313122, -1.733590290792417887, 0.000000000000000000 ) ) ;
#4039=CARTESIAN_POINT ( 'NONE',  ( 0.1352650258312465548, -28.50015511220833986, 3.957670871000018575 ) ) ;
#4045=EDGE_CURVE ( 'NONE', #1904, #17421, #22788, .T. ) ;
#4054=CARTESIAN_POINT ( 'NONE',  ( -15.73360964037622622, -8.979988381802643360, -0.6999999999999784173 ) ) ;
#4058=CARTESIAN_POINT ( 'NONE',  ( 18.03376228222516886, 11.69189214368329743, -4.336808689942017736E-16 ) ) ;
#4067=ORIENTED_EDGE ( 'NONE', *, *, #15423, .T. ) ;
#4078=CARTESIAN_POINT ( 'NONE',  ( -16.85343921394901301, 12.09981795542885585, -1.000005633855494125E-09 ) ) ;
#4088=CARTESIAN_POINT ( 'NONE',  ( 27.83860951759415059, -1.869044369023509899, 8.000000000000007105 ) ) ;
#4107=ORIENTED_EDGE ( 'NONE', *, *, #27923, .T. ) ;
#4109=CARTESIAN_POINT ( 'NONE',  ( 23.23955039760055641, 15.25661106415676471, 4.791628269000009155 ) ) ;
#4110=CARTESIAN_POINT ( 'NONE',  ( -23.83861932771936765, -15.61961844720760340, 4.689445057000002137 ) ) ;
#4118=B_SPLINE_CURVE_WITH_KNOTS ( 'NONE', 5,
 ( #30487, #6703, #10967, #6078, #27957, #16307, #13638, #1684, #15999 ),
 .UNSPECIFIED., .F., .F.,
 ( 6, 3, 6 ),
 ( 0.000000000000000000, 0.7281981532490000575, 1.224410044450000123 ),
 .UNSPECIFIED. ) ;
#4125=CARTESIAN_POINT ( 'NONE',  ( -25.00848080823378083, 13.67001762859745639, 6.099998581000005693 ) ) ;
#4128=CARTESIAN_POINT ( 'NONE',  ( 1.000415564672181512, -28.48292217092965828, 6.002515439000016606 ) ) ;
#4134=CARTESIAN_POINT ( 'NONE',  ( 18.26900987428666667, 10.87604578382501330, -4.336808689942017736E-16 ) ) ;
#4137=B_SPLINE_CURVE_WITH_KNOTS ( 'NONE', 1,
 ( #28887, #16615 ),
 .UNSPECIFIED., .F., .F.,
 ( 2, 2 ),
 ( -2.557514682700000071E-06, 0.7000000000009999335 ),
 .UNSPECIFIED. ) ;
#4141=ORIENTED_EDGE ( 'NONE', *, *, #13915, .F. ) ;
#4155=CARTESIAN_POINT ( 'NONE',  ( -18.66687140124644984, 20.92780155647522378, -0.2432540810000105580 ) ) ;
#4165=VERTEX_POINT ( 'NONE', #28756 ) ;
#4169=CARTESIAN_POINT ( 'NONE',  ( 26.85610471403804311, 4.933999481336595494, 0.000000000000000000 ) ) ;
#4186=CARTESIAN_POINT ( 'NONE',  ( -25.12347730974626714, -15.01204873981462384, 0.7069225330000039609 ) ) ;
#4192=CARTESIAN_POINT ( 'NONE',  ( -0.3076636919694037964, -28.49867017228337573, 4.240370246000018994 ) ) ;
#4194=CARTESIAN_POINT ( 'NONE',  ( -24.41841039498785193, -14.69667350221323865, 6.099998581000020792 ) ) ;
#4195=ORIENTED_EDGE ( 'NONE', *, *, #30349, .F. ) ;
#4196=CARTESIAN_POINT ( 'NONE',  ( 28.35945635826399780, 7.983396865336832349, 1.000000000000000888 ) ) ;
#4206=CARTESIAN_POINT ( 'NONE',  ( -24.24144457387483698, -14.48500828217274439, 0.000000000000000000 ) ) ;
#4220=ORIENTED_EDGE ( 'NONE', *, *, #9740, .F. ) ;
#4221=VECTOR ( 'NONE', #14826, 1000.000000000000000 ) ;
#4241=ADVANCED_FACE ( 'NONE', ( #10650 ), #14541, .F. ) ;
#4246=CARTESIAN_POINT ( 'NONE',  ( -20.08700151986557358, -19.43868425012845336, 8.000000000000007105 ) ) ;
#4251=VECTOR ( 'NONE', #18365, 1000.000000000000000 ) ;
#4252=CARTESIAN_POINT ( 'NONE',  ( 28.40974773466432168, 5.219434544874079762, 0.7595836940000044724 ) ) ;
#4254=CARTESIAN_POINT ( 'NONE',  ( -17.90985823243290298, 11.26838425369655816, -4.336808689942017243E-16 ) ) ;
#4259=VERTEX_POINT ( 'NONE', #27474 ) ;
#4271=CARTESIAN_POINT ( 'NONE',  ( 23.82471740507292068, 15.64077205896351508, 4.791628269000009155 ) ) ;
#4298=CARTESIAN_POINT ( 'NONE',  ( 0.9015611980529183445, -28.48625233387473799, 3.957673652000032405 ) ) ;
#4308=ORIENTED_EDGE ( 'NONE', *, *, #13149, .T. ) ;
#4309=CARTESIAN_POINT ( 'NONE',  ( 24.92013865993870425, -13.82966158318416738, 6.099998581000020792 ) ) ;
#4318=CARTESIAN_POINT ( 'NONE',  ( -19.98350515471250688, 19.99996606751605555, 0.1429766398601999555 ) ) ;
#4321=ADVANCED_FACE ( 'NONE', ( #25917 ), #9753, .T. ) ;
#4326=CARTESIAN_POINT ( 'NONE',  ( 18.03540948931063070, 11.69027953332313352, -0.6999999999999784173 ) ) ;
#4336=CARTESIAN_POINT ( 'NONE',  ( 24.43008698959658176, -14.67811372800087000, 4.492876031999992748 ) ) ;
#4337=CARTESIAN_POINT ( 'NONE',  ( 16.29938252748853245, -9.691892145436083794, -0.6999999999999783062 ) ) ;
#4339=CARTESIAN_POINT ( 'NONE',  ( 2.484315071036837352, -2.507604248800407554, -0.6999999999999783062 ) ) ;
#4340=CARTESIAN_POINT ( 'NONE',  ( -23.99239029816459734, 14.04409902692776591, 5.882927410969883475 ) ) ;
#4346=CARTESIAN_POINT ( 'NONE',  ( -27.79539923781770483, -0.5057481688778118212, 0.8585786439999909536 ) ) ;
#4347=ORIENTED_EDGE ( 'NONE', *, *, #25464, .F. ) ;
#4357=CARTESIAN_POINT ( 'NONE',  ( 19.80526555972147307, 19.50877392102524155, 3.000000000000002665 ) ) ;
#4387=CARTESIAN_POINT ( 'NONE',  ( -27.66290831536081285, -7.787312998891453120, 8.000000000000007105 ) ) ;
#4399=B_SPLINE_SURFACE_WITH_KNOTS ( 'NONE', 5, 1, ( 
 ( #24970, #24665 ),
 ( #1217, #1060 ),
 ( #17571, #29535 ),
 ( #3406, #3099 ),
 ( #17714, #12695 ),
 ( #13008, #10813 ),
 ( #10651, #27177 ),
 ( #17870, #27475 ),
 ( #7661, #24514 ),
 ( #22307, #20242 ),
 ( #29842, #2951 ),
 ( #5616, #3254 ),
 ( #15216, #24821 ),
 ( #17417, #29377 ),
 ( #22151, #27332 ) ),
 .UNSPECIFIED., .F., .F., .F.,
 ( 6, 3, 3, 3, 6 ),
 ( 2, 2 ),
 ( 0.000000000000000000, 0.5239049114029999954, 1.047809822800000124, 1.571714734209999964, 1.746349704670000058 ),
 ( -0.7000000000009999335, 2.557514682700000071E-06 ),
 .UNSPECIFIED. ) ;
#4400=CARTESIAN_POINT ( 'NONE',  ( 27.95444821424234405, 5.135786986018160860, -0.2432540810000105580 ) ) ;
#4427=CARTESIAN_POINT ( 'NONE',  ( 19.95603390318983372, 20.00015565088524738, 0.1175284324535141589 ) ) ;
#4439=CARTESIAN_POINT ( 'NONE',  ( 24.98081130624543889, 13.71897605842228529, 4.999998581000003384 ) ) ;
#4443=CARTESIAN_POINT ( 'NONE',  ( 24.05407933487299132, -13.93841814072233909, 5.964141603158990002 ) ) ;
#4444=CARTESIAN_POINT ( 'NONE',  ( 0.7646642646963620615, -28.49022165133369455, 6.079790450999988494 ) ) ;
#4446=ORIENTED_EDGE ( 'NONE', *, *, #1962, .T. ) ;
#4448=CARTESIAN_POINT ( 'NONE',  ( -24.74993094845043018, 14.13250375615880117, 6.042507811999997536 ) ) ;
#4450=EDGE_LOOP ( 'NONE', ( #26699, #29595, #28166, #24278 ) ) ;
#4456=CARTESIAN_POINT ( 'NONE',  ( -16.04158851046123502, 10.23646161653652875, -0.6999999999999784173 ) ) ;
#4471=VERTEX_POINT ( 'NONE', #2766 ) ;
#4477=EDGE_LOOP ( 'NONE', ( #20975, #14371, #15583, #26180 ) ) ;
#4478=CARTESIAN_POINT ( 'NONE',  ( -23.31496426210264516, -15.14116962587117143, 4.441687039633147371 ) ) ;
#4479=CARTESIAN_POINT ( 'NONE',  ( 1.157672466085042151, -27.77645868488912484, 4.099089508000003157 ) ) ;
#4480=CARTESIAN_POINT ( 'NONE',  ( 18.26639035964474900, 11.02001161816309072, -0.6999999999999784173 ) ) ;
#4487=ORIENTED_EDGE ( 'NONE', *, *, #353, .T. ) ;
#4501=CARTESIAN_POINT ( 'NONE',  ( 24.83827260354858524, -12.48687744687322621, 4.852954933405435156 ) ) ;
#4505=CARTESIAN_POINT ( 'NONE',  ( -24.36936511100012481, -14.56144439311391636, 0.000000000000000000 ) ) ;
#4511=CARTESIAN_POINT ( 'NONE',  ( 0.4024591535043843260, -27.79733476267318437, 3.904047916000019658 ) ) ;
#4515=DIRECTION ( 'NONE',  ( -0.000000000000000000, 0.000000000000000000, 1.000000000000000000 ) ) ;
#4521=CARTESIAN_POINT ( 'NONE',  ( -24.34137756212881953, 13.42980562992878646, 3.899998581000013509 ) ) ;
#4526=CARTESIAN_POINT ( 'NONE',  ( -16.09345594084761188, -8.185437083264902824, 0.000000000000000000 ) ) ;
#4535=EDGE_CURVE ( 'NONE', #8375, #24893, #22444, .T. ) ;
#4539=CARTESIAN_POINT ( 'NONE',  ( -27.87609112763790975, 3.928995115430390150, 1.000000000000000888 ) ) ;
#4550=CARTESIAN_POINT ( 'NONE',  ( 27.90810418749530086, 6.414199157211339042, 8.000000000000007105 ) ) ;
#4551=CARTESIAN_POINT ( 'NONE',  ( 24.73568148353697183, -12.68911065183860920, 5.680831396999986183 ) ) ;
#4552=B_SPLINE_CURVE_WITH_KNOTS ( 'NONE', 3,
 ( #20897, #8921, #28273, #10979, #20732, #27966, #16008, #25621, #18521, #28123 ),
 .UNSPECIFIED., .F., .F.,
 ( 4, 2, 2, 2, 4 ),
 ( 0.000000000000000000, 0.2500000000000000000, 0.5000000000000000000, 0.7500000000000000000, 1.000000000000000000 ),
 .UNSPECIFIED. ) ;
#4554=CARTESIAN_POINT ( 'NONE',  ( -15.73360964030186970, 11.02001161816959396, -0.6999999999999784173 ) ) ;
#4555=CARTESIAN_POINT ( 'NONE',  ( -19.79264346680938758, 19.51191464210150173, 0.8505138480000007384 ) ) ;
#4556=CARTESIAN_POINT ( 'NONE',  ( 27.55801272791059731, 0.5014288284349612823, -0.5592437529999827461 ) ) ;
#4573=CARTESIAN_POINT ( 'NONE',  ( 23.78314118259453380, 14.39461387841678608, 3.901343066999990228 ) ) ;
#4576=CARTESIAN_POINT ( 'NONE',  ( 20.04888805111184524, 19.99998387947535861, 0.2364017625693574376 ) ) ;
#4583=FACE_BOUND ( 'NONE', #7581, .T. ) ;
#4584=CARTESIAN_POINT ( 'NONE',  ( 24.36724935763797006, 13.38201651305720574, 5.104178997000024864 ) ) ;
#4585=PLANE ( 'NONE',  #21690 ) ;
#4590=CARTESIAN_POINT ( 'NONE',  ( 1.607747500023186893, -28.45491842328712551, 5.310199493000017590 ) ) ;
#4596=DIRECTION ( 'NONE',  ( -0.000000000000000000, 0.000000000000000000, 1.000000000000000000 ) ) ;
#4599=CARTESIAN_POINT ( 'NONE',  ( 23.87963657767028280, 15.55698410313905988, 4.493007569000006640 ) ) ;
#4603=B_SPLINE_CURVE_WITH_KNOTS ( 'NONE', 5,
 ( #13439, #16117, #21309, #13603, #23209, #18320, #16268, #15962, #8714 ),
 .UNSPECIFIED., .F., .F.,
 ( 6, 3, 6 ),
 ( 8.011061266649999624, 9.405960541640000727, 10.80085981660000094 ),
 .UNSPECIFIED. ) ;
#4617=CARTESIAN_POINT ( 'NONE',  ( -20.30403093138962234, 20.00000000003553424, 1.000000000000000888 ) ) ;
#4627=CYLINDRICAL_SURFACE ( 'NONE', #17977, 1.099999999999999867 ) ;
#4629=EDGE_CURVE ( 'NONE', #3424, #13976, #8146, .T. ) ;
#4631=DIRECTION ( 'NONE',  ( 0.000000000000000000, 0.000000000000000000, -1.000000000000000000 ) ) ;
#4632=CYLINDRICAL_SURFACE ( 'NONE', #12252, 1.099999999999999867 ) ;
#4633=VERTEX_POINT ( 'NONE', #20210 ) ;
#4644=CARTESIAN_POINT ( 'NONE',  ( 1.605176535610508326, -27.75389821387976852, 4.895940783000013674 ) ) ;
#4646=CARTESIAN_POINT ( 'NONE',  ( -19.38902494840800017, 18.61775191683619823, 0.000000000000000000 ) ) ;
#4653=CARTESIAN_POINT ( 'NONE',  ( -24.40022624598054435, -14.72688605908970239, 3.899998581000013509 ) ) ;
#4663=CARTESIAN_POINT ( 'NONE',  ( -15.73632211102524181, -9.091892911704846370, 0.000000000000000000 ) ) ;
#4666=CARTESIAN_POINT ( 'NONE',  ( -16.04158851046123502, 10.23646161653652875, -0.6999999999999784173 ) ) ;
#4674=CARTESIAN_POINT ( 'NONE',  ( 24.92639507930385889, 13.81781707913292934, 5.506973475999988210 ) ) ;
#4680=B_SPLINE_CURVE_WITH_KNOTS ( 'NONE', 3,
 ( #24026, #31104, #18669, #9545 ),
 .UNSPECIFIED., .F., .F.,
 ( 4, 4 ),
 ( 0.000000000000000000, 1.000000000000000000 ),
 .UNSPECIFIED. ) ;
#4706=CARTESIAN_POINT ( 'NONE',  ( -16.06988921231594603, 11.79183908526949054, -0.6999999999999784173 ) ) ;
#4708=CARTESIAN_POINT ( 'NONE',  ( 24.37165445055180157, -14.77472140295711434, 4.999998581000003384 ) ) ;
#4711=CARTESIAN_POINT ( 'NONE',  ( -24.96253706803760153, -13.75225324404262572, 5.310538869999992251 ) ) ;
#4725=ORIENTED_EDGE ( 'NONE', *, *, #291, .T. ) ;
#4728=B_SPLINE_CURVE_WITH_KNOTS ( 'NONE', 3,
 ( #24508, #455, #24197, #5001, #19327, #7207 ),
 .UNSPECIFIED., .F., .F.,
 ( 4, 2, 4 ),
 ( 0.000000000000000000, 0.5000000000000000000, 1.000000000000000000 ),
 .UNSPECIFIED. ) ;
#4729=B_SPLINE_SURFACE_WITH_KNOTS ( 'NONE', 5, 1, ( 
 ( #20882, #3716 ),
 ( #13315, #25914 ),
 ( #22926, #1997 ),
 ( #30781, #1367 ),
 ( #25447, #30482 ),
 ( #20557, #11119 ),
 ( #14416, #23710 ),
 ( #21341, #415 ),
 ( #19129, #28880 ),
 ( #4962, #14106 ),
 ( #7478, #11890 ),
 ( #26216, #26522 ),
 ( #21493, #7329 ),
 ( #4653, #16914 ),
 ( #16608, #24162 ) ),
 .UNSPECIFIED., .F., .F., .F.,
 ( 6, 3, 3, 3, 6 ),
 ( 2, 2 ),
 ( 0.000000000000000000, 0.5238999883129999979, 1.047799976630000129, 1.571699964940000083, 1.746333294380000067 ),
 ( -0.7000000000009999335, 2.555882144480000001E-06 ),
 .UNSPECIFIED. ) ;
#4736=CARTESIAN_POINT ( 'NONE',  ( 20.04510529260553042, 19.99998683332297489, 0.2311123248240848915 ) ) ;
#4756=CARTESIAN_POINT ( 'NONE',  ( 23.77307027438277842, -14.41181805763364210, 5.147042609327748153 ) ) ;
#4776=CARTESIAN_POINT ( 'NONE',  ( 28.49528339128749366, 0.5184828350247757678, 0.7595836940000044724 ) ) ;
#4778=CARTESIAN_POINT ( 'NONE',  ( 18.11750013295242212, -8.428624923737988439, -4.336808689942017243E-16 ) ) ;
#4793=CARTESIAN_POINT ( 'NONE',  ( -23.67228571422688788, -14.57675966245750665, 3.926818800612126292 ) ) ;
#4794=CARTESIAN_POINT ( 'NONE',  ( 0.6243462152986178904, -28.49342029039284085, 3.904048352000033528 ) ) ;
#4804=CARTESIAN_POINT ( 'NONE',  ( -16.81341597763548990, -10.09981795544978311, -0.6999999999999784173 ) ) ;
#4813=CARTESIAN_POINT ( 'NONE',  ( 24.06001628433582695, 15.27670955088212068, 5.888744266207340594 ) ) ;
#4828=CARTESIAN_POINT ( 'NONE',  ( -23.81776757772072983, -15.65134804123479917, 4.999998581000003384 ) ) ;
#4834=CARTESIAN_POINT ( 'NONE',  ( -25.41286868644903763, 12.90211872717319430, 4.492873454000012146 ) ) ;
#4839=CARTESIAN_POINT ( 'NONE',  ( 24.61381495442905276, 14.36755986797187923, 6.042472827000016977 ) ) ;
#4854=CARTESIAN_POINT ( 'NONE',  ( -27.87609112763790975, 3.928995115430390150, 2.400000000000013234 ) ) ;
#4877=CARTESIAN_POINT ( 'NONE',  ( 24.93720649360215802, -13.79881813812812297, 3.899998581000013509 ) ) ;
#4888=CARTESIAN_POINT ( 'NONE',  ( 24.36724935763797006, 13.38201651305720574, 4.895818164000031558 ) ) ;
#4892=EDGE_CURVE ( 'NONE', #3434, #19387, #30298, .T. ) ;
#4893=CARTESIAN_POINT ( 'NONE',  ( 19.40982886648660255, 20.00003049653962606, -0.3209631320504065521 ) ) ;
#4897=CYLINDRICAL_SURFACE ( 'NONE', #24062, 1.099999999999999867 ) ;
#4901=CARTESIAN_POINT ( 'NONE',  ( 24.43008698959658176, -14.67811372800087000, 5.507121129000008608 ) ) ;
#4902=CARTESIAN_POINT ( 'NONE',  ( 24.83401022448529005, 13.98326749045440032, 5.760125282000011282 ) ) ;
#4907=CARTESIAN_POINT ( 'NONE',  ( -24.98081131316241255, -13.71897606304888662, 4.895818166000015736 ) ) ;
#4914=CARTESIAN_POINT ( 'NONE',  ( 24.40022624086872938, 14.72688605419589614, 3.899998581000013509 ) ) ;
#4915=ORIENTED_EDGE ( 'NONE', *, *, #25016, .T. ) ;
#4921=CARTESIAN_POINT ( 'NONE',  ( 17.16657240419154462, 10.99999999996915179, -0.6999999999999784173 ) ) ;
#4924=CARTESIAN_POINT ( 'NONE',  ( 26.79556473285982321, 0.4875557887249851730, -0.6999999999999784173 ) ) ;
#4933=CARTESIAN_POINT ( 'NONE',  ( 17.95841148951064525, -9.763538383420391042, -0.6999999999999784173 ) ) ;
#4962=CARTESIAN_POINT ( 'NONE',  ( -24.21906834513991313, -15.02342241408235068, 3.957526371000025023 ) ) ;
#4978=CARTESIAN_POINT ( 'NONE',  ( 23.27660429769468919, -19.83288784532059168, -0.5592437529999827461 ) ) ;
#4984=CARTESIAN_POINT ( 'NONE',  ( -16.11786738712100941, -8.163589694621649073, 0.000000000000000000 ) ) ;
#4987=CARTESIAN_POINT ( 'NONE',  ( 19.80526555972147307, 19.50877392102524155, 1.000000000000000888 ) ) ;
#4989=EDGE_LOOP ( 'NONE', ( #16987, #24151, #27357, #3350 ) ) ;
#5001=CARTESIAN_POINT ( 'NONE',  ( -16.26054471315379857, -9.950349629747549329, -0.6999999999999784173 ) ) ;
#5004=CARTESIAN_POINT ( 'NONE',  ( -20.30403093128963476, 20.00000000003735323, 1.800000043000016259 ) ) ;
#5006=CYLINDRICAL_SURFACE ( 'NONE', #968, 1.099999999999999867 ) ;
#5014=B_SPLINE_SURFACE_WITH_KNOTS ( 'NONE', 5, 1, ( 
 ( #4439, #16543 ),
 ( #26152, #4584 ),
 ( #14192, #23795 ),
 ( #2242, #11832 ),
 ( #12436, #14964 ),
 ( #26762, #19379 ),
 ( #4902, #5197 ),
 ( #2690, #28660 ),
 ( #655, #12291 ),
 ( #21736, #14507 ),
 ( #16691, #29120 ),
 ( #9619, #17010 ),
 ( #21903, #10242 ),
 ( #14814, #349 ),
 ( #24103, #7564 ) ),
 .UNSPECIFIED., .F., .F., .F.,
 ( 6, 3, 3, 3, 6 ),
 ( 2, 2 ),
 ( 0.000000000000000000, 0.5239010159489999596, 1.047802031900000097, 1.571703047840000034, 1.746336719830000161 ),
 ( -0.7000000000009999335, 2.556023102059999913E-06 ),
 .UNSPECIFIED. ) ;
#5022=CARTESIAN_POINT ( 'NONE',  ( -24.39135169139800041, 14.74223402946396000, 5.310643621000004977 ) ) ;
#5028=CARTESIAN_POINT ( 'NONE',  ( 24.83272649506304219, -12.49791454618707398, 4.791562841999996714 ) ) ;
#5031=EDGE_CURVE ( 'NONE', #26158, #6269, #13397, .T. ) ;
#5037=DIRECTION ( 'NONE',  ( 0.6941258031311203780, 0.7198537139083029945, 0.000000000000000000 ) ) ;
#5039=CARTESIAN_POINT ( 'NONE',  ( 27.75695160390876737, 2.618790587933454983, 8.000000000000007105 ) ) ;
#5041=CARTESIAN_POINT ( 'NONE',  ( 19.88917888186078997, 20.00030014464526218, 0.04289124618241111492 ) ) ;
#5042=EDGE_CURVE ( 'NONE', #13946, #7965, #20023, .T. ) ;
#5043=CARTESIAN_POINT ( 'NONE',  ( -23.92481352202500489, 14.15879617713575911, 5.760265123000013254 ) ) ;
#5050=CARTESIAN_POINT ( 'NONE',  ( 23.92481352800953331, -14.15879618172764509, 5.760265122000007842 ) ) ;
#5063=AXIS2_PLACEMENT_3D ( 'NONE', #14348, #25990, #23950 ) ;
#5072=EDGE_LOOP ( 'NONE', ( #26318, #22829 ) ) ;
#5077=CARTESIAN_POINT ( 'NONE',  ( -24.73568147689258367, 12.68911064945909217, 5.680831397999991594 ) ) ;
#5095=CARTESIAN_POINT ( 'NONE',  ( 17.83929014045347827, 20.00000000006149392, -1.000005633855494125E-09 ) ) ;
#5096=CARTESIAN_POINT ( 'NONE',  ( -27.71261514784112379, -0.5042418800003600765, 0.5514269430000329208 ) ) ;
#5101=B_SPLINE_SURFACE_WITH_KNOTS ( 'NONE', 5, 1, ( 
 ( #21847, #21688 ),
 ( #28918, #14757 ),
 ( #2640, #12232 ),
 ( #23368, #9878 ),
 ( #26707, #26410 ),
 ( #10038, #19478 ),
 ( #29069, #7514 ),
 ( #19631, #29214 ),
 ( #17258, #26868 ),
 ( #19790, #5311 ),
 ( #14914, #2947 ),
 ( #12540, #22148 ),
 ( #5459, #603 ),
 ( #10189, #29373 ),
 ( #17412, #27020 ) ),
 .UNSPECIFIED., .F., .F., .F.,
 ( 6, 3, 3, 3, 6 ),
 ( 2, 2 ),
 ( 0.000000000000000000, 0.5239055193140000899, 1.047811038630000136, 1.571716557940000092, 1.746351731040000077 ),
 ( -0.7000000000009999335, 2.557301831960000071E-06 ),
 .UNSPECIFIED. ) ;
#5103=( LENGTH_UNIT ( ) NAMED_UNIT ( * ) SI_UNIT ( .MILLI., .METRE. ) );
#5110=B_SPLINE_CURVE_WITH_KNOTS ( 'NONE', 3,
 ( #18658, #8906, #13472, #1214, #25759, #13791 ),
 .UNSPECIFIED., .F., .F.,
 ( 4, 2, 4 ),
 ( 0.000000000000000000, 0.5000000000000000000, 1.000000000000000000 ),
 .UNSPECIFIED. ) ;
#5116=ORIENTED_EDGE ( 'NONE', *, *, #10597, .F. ) ;
#5125=CARTESIAN_POINT ( 'NONE',  ( -20.77600556904588913, -21.68409854326813146, 1.000000000000000888 ) ) ;
#5130=CARTESIAN_POINT ( 'NONE',  ( -16.06988921231594603, 11.79183908526949054, -0.6999999989999727834 ) ) ;
#5140=CARTESIAN_POINT ( 'NONE',  ( 17.18658402238548533, 9.900182044515950963, -1.000005633855494125E-09 ) ) ;
#5144=CARTESIAN_POINT ( 'NONE',  ( -27.07233446881492611, 8.380004974212880597, 1.000000000000000888 ) ) ;
#5146=B_SPLINE_CURVE_WITH_KNOTS ( 'NONE', 5,
 ( #12288, #9616, #7562, #7408, #14190, #16851, #2687, #21587, #19530, #21900, #16689, #14504, #24101, #9457, #26457, #347, #30873, #7262, #12127, #17153, #9929 ),
 .UNSPECIFIED., .F., .F.,
 ( 6, 3, 3, 3, 3, 3, 6 ),
 ( -15.54987830269999982, -12.96130453750000022, -10.36904362289999959, -7.776782722820000160, -5.184521831719999696, -2.592260920730000251, 0.000000000000000000 ),
 .UNSPECIFIED. ) ;
#5161=CARTESIAN_POINT ( 'NONE',  ( -20.15224477982290452, 20.00000015333570857, 0.3713946529999845314 ) ) ;
#5162=B_SPLINE_SURFACE_WITH_KNOTS ( 'NONE', 5, 1, ( 
 ( #20146, #3605 ),
 ( #25019, #15115 ),
 ( #17763, #10396 ),
 ( #5819, #18075 ),
 ( #15417, #3451 ),
 ( #6126, #8320 ),
 ( #13053, #29894 ),
 ( #17915, #27524 ),
 ( #22200, #22813 ) ),
 .UNSPECIFIED., .F., .F., .F.,
 ( 6, 3, 6 ),
 ( 2, 2 ),
 ( 0.000000000000000000, 55.31395627319999875, 94.75474476520000167 ),
 ( -3.500000000000000000, 3.500000000000000000 ),
 .UNSPECIFIED. ) ;
#5166=CARTESIAN_POINT ( 'NONE',  ( -24.37165444408190851, 14.77472139917419369, 5.104215870000011535 ) ) ;
#5169=ORIENTED_EDGE ( 'NONE', *, *, #9740, .T. ) ;
#5181=ORIENTED_EDGE ( 'NONE', *, *, #23655, .F. ) ;
#5185=CARTESIAN_POINT ( 'NONE',  ( 23.80322556508107112, 14.59355840047072661, 1.000000000000000888 ) ) ;
#5195=CARTESIAN_POINT ( 'NONE',  ( -27.79539923781770128, -0.5057481688779147389, 8.000000000000007105 ) ) ;
#5196=CARTESIAN_POINT ( 'NONE',  ( 23.79228474585360686, -14.38012950158411662, 5.310643619999999565 ) ) ;
#5197=CARTESIAN_POINT ( 'NONE',  ( 24.22405392119105016, 13.63981656816893739, 5.760125282000011282 ) ) ;
#5205=CARTESIAN_POINT ( 'NONE',  ( -24.96253706803760153, -13.75225324404262572, 4.689458291000009105 ) ) ;
#5210=CARTESIAN_POINT ( 'NONE',  ( 1.645560275461343203, -28.45273235261698019, 4.895940783000013674 ) ) ;
#5228=CARTESIAN_POINT ( 'NONE',  ( -25.35851007062240114, 13.00862288638852959, 5.680831397999991594 ) ) ;
#5246=EDGE_CURVE ( 'NONE', #5717, #13930, #5146, .T. ) ;
#5249=DIRECTION ( 'NONE',  ( 0.000000000000000000, 0.000000000000000000, -1.000000000000000000 ) ) ;
#5257=CARTESIAN_POINT ( 'NONE',  ( -26.93580492059415121, 9.103810007694223216, 1.000000000000000888 ) ) ;
#5273=B_SPLINE_CURVE_WITH_KNOTS ( 'NONE', 5,
 ( #9704, #12216, #18992, #7038, #19617, #4839, #11910, #21827, #16628, #283, #4674, #26236, #14284, #19463, #14436 ),
 .UNSPECIFIED., .F., .F.,
 ( 6, 3, 3, 3, 6 ),
 ( 0.000000000000000000, 0.1000000000040084519, 0.3999999999988547716, 0.6999999999999999556, 1.000000000000000000 ),
 .UNSPECIFIED. ) ;
#5274=B_SPLINE_CURVE_WITH_KNOTS ( 'NONE', 1,
 ( #23840, #6678 ),
 .UNSPECIFIED., .F., .F.,
 ( 2, 2 ),
 ( -2.556026163500000058E-06, 0.7000000000009999335 ),
 .UNSPECIFIED. ) ;
#5287=CARTESIAN_POINT ( 'NONE',  ( -23.81776757772072983, -15.65134804123479917, 5.104183903000020450 ) ) ;
#5289=CARTESIAN_POINT ( 'NONE',  ( -23.89302272057183885, -14.21215728459360150, 3.899998580999983311 ) ) ;
#5292=CARTESIAN_POINT ( 'NONE',  ( -26.90707039800299327, -7.574539066456210001, -0.6999999999999784173 ) ) ;
#5297=CARTESIAN_POINT ( 'NONE',  ( 17.43495665862128874, 12.07643063644571946, 1.385610376436474414E-13 ) ) ;
#5299=CARTESIAN_POINT ( 'NONE',  ( 18.26639035964474900, 11.02001161816309072, -0.6999999999999784173 ) ) ;
#5311=CARTESIAN_POINT ( 'NONE',  ( -24.14205448738587023, 13.78537896750705194, 3.957489350000009676 ) ) ;
#5319=CARTESIAN_POINT ( 'NONE',  ( 24.75645985066740806, 14.12045945716145390, 4.098702612000016288 ) ) ;
#5339=VERTEX_POINT ( 'NONE', #28656 ) ;
#5347=CARTESIAN_POINT ( 'NONE',  ( 27.51770821235203357, 4.728187301808492116, 1.000000000000000888 ) ) ;
#5358=CARTESIAN_POINT ( 'NONE',  ( 24.88589369718092215, -13.89120818692358483, 6.095967889000020179 ) ) ;
#5359=CARTESIAN_POINT ( 'NONE',  ( 20.25359293946302941, 20.00000005145030002, 0.6182840029999858711 ) ) ;
#5363=B_SPLINE_SURFACE_WITH_KNOTS ( 'NONE', 5, 1, ( 
 ( #18192, #25454 ),
 ( #1844, #3566 ),
 ( #20563, #6248 ),
 ( #13160, #29995 ),
 ( #1220, #15851 ),
 ( #3888, #27636 ),
 ( #6081, #11127 ),
 ( #4196, #20724 ),
 ( #15679, #25289 ) ),
 .UNSPECIFIED., .F., .F., .F.,
 ( 6, 3, 6 ),
 ( 2, 2 ),
 ( 0.000000000000000000, 55.31395511720000258, 94.75474465359999954 ),
 ( -3.500000000000000000, 3.500000000000000000 ),
 .UNSPECIFIED. ) ;
#5364=CARTESIAN_POINT ( 'NONE',  ( 0.9758793681798838549, -27.78334643822867633, 6.002515439000016606 ) ) ;
#5371=ORIENTED_EDGE ( 'NONE', *, *, #26182, .F. ) ;
#5372=CARTESIAN_POINT ( 'NONE',  ( 23.55411374389282386, 16.04538543799059980, 8.000000000000007105 ) ) ;
#5385=CARTESIAN_POINT ( 'NONE',  ( 0.4478609109052260062, -28.49673184309145668, 6.098651241000007772 ) ) ;
#5397=B_SPLINE_CURVE_WITH_KNOTS ( 'NONE', 5,
 ( #29540, #29384, #21858, #309, #3104, #22466, #7666, #24365, #15073, #29076, #27030, #26717, #7522, #24826, #2806 ),
 .UNSPECIFIED., .F., .F.,
 ( 6, 3, 3, 3, 6 ),
 ( 0.000000000000000000, 0.2999999999994274469, 0.6000000000000000888, 0.8999999999971368680, 1.000000000000000000 ),
 .UNSPECIFIED. ) ;
#5404=CARTESIAN_POINT ( 'NONE',  ( -24.95150188576097960, 13.62250486154599294, 1.000000000000000888 ) ) ;
#5405=EDGE_CURVE ( 'NONE', #931, #3809, #10010, .T. ) ;
#5413=CARTESIAN_POINT ( 'NONE',  ( -24.49145440958036701, 14.57548795270903774, 4.319167817000008291 ) ) ;
#5420=CARTESIAN_POINT ( 'NONE',  ( -22.26220695934820171, 17.72099999758041378, -0.2432540810000105580 ) ) ;
#5425=B_SPLINE_CURVE_WITH_KNOTS ( 'NONE', 3,
 ( #21762, #17182, #24434, #12151, #26479, #10114 ),
 .UNSPECIFIED., .F., .F.,
 ( 4, 2, 4 ),
 ( 0.000000000000000000, 0.5000000000000000000, 1.000000000000000000 ),
 .UNSPECIFIED. ) ;
#5438=CARTESIAN_POINT ( 'NONE',  ( -27.03594125075309762, -0.4919295335571663430, -0.6999999999999784173 ) ) ;
#5441=CARTESIAN_POINT ( 'NONE',  ( 17.82645929468907298, 11.89178602526930817, 1.385610376436474667E-13 ) ) ;
#5443=CARTESIAN_POINT ( 'NONE',  ( -0.1464386042498656837, -27.80011885101298930, 5.900904413000008120 ) ) ;
#5456=CARTESIAN_POINT ( 'NONE',  ( 27.89787437582684859, -9.677414786515893041, 0.5514269430000329208 ) ) ;
#5459=CARTESIAN_POINT ( 'NONE',  ( -24.90302310912370132, 13.86047864606265279, 3.901342110999989288 ) ) ;
#5463=CARTESIAN_POINT ( 'NONE',  ( -23.81866442513004856, -14.33570206453694240, 6.099998581000020792 ) ) ;
#5464=EDGE_LOOP ( 'NONE', ( #6335, #14608, #8373, #8852 ) ) ;
#5485=ORIENTED_EDGE ( 'NONE', *, *, #25016, .F. ) ;
#5494=CARTESIAN_POINT ( 'NONE',  ( 24.45473033137484720, 14.63622297804190175, 3.901342939999996595 ) ) ;
#5503=CARTESIAN_POINT ( 'NONE',  ( -21.02347494288676444, 19.26966991725469214, 4.000000085000010586 ) ) ;
#5507=CLOSED_SHELL ( 'NONE', ( #28429, #14817, #24150, #7508, #9986, #22534, #15077, #15194, #6951, #26124, #12842, #22434, #21444, #14875, #6897, #15867, #20612, #20588, #12531, #20010, #23916, #13038, #2267, #9320, #21326, #960, #26760, #7656, #30412, #18005, #22339, #19436, #18350, #16036, #25526, #20667, #6380, #22676, #16756, #19261, #28327, #245, #101, #30474, #16107, #26480, #18032, #15998, #7988, #11945, #21408, #10580, #8252, #15543, #2848, #18734, #4241, #11078, #2759, #15297, #16883, #21597, #27136, #8346, #27876, #29077, #772, #5621, #28997, #3271, #28612, #15978, #19490, #22543, #3751, #28061, #20941, #4321 ) ) ;
#5508=CARTESIAN_POINT ( 'NONE',  ( 27.79539923781684507, 0.5057481689249235801, 8.000000000000007105 ) ) ;
#5510=FACE_BOUND ( 'NONE', #12271, .T. ) ;
#5516=CARTESIAN_POINT ( 'NONE',  ( -24.92639508767336309, -13.81781708088548122, 4.493023692000025271 ) ) ;
#5519=CARTESIAN_POINT ( 'NONE',  ( 1.344125205454980154, -28.46870209102154448, 4.240358041999986227 ) ) ;
#5529=ORIENTED_EDGE ( 'NONE', *, *, #6615, .F. ) ;
#5536=CARTESIAN_POINT ( 'NONE',  ( -23.89299059146159010, -14.21221066648391052, 6.099998581000002140 ) ) ;
#5543=CARTESIAN_POINT ( 'NONE',  ( 24.26032293416166041, 13.57529002140354812, 5.676497403531009844 ) ) ;
#5555=B_SPLINE_CURVE_WITH_KNOTS ( 'NONE', 5,
 ( #23629, #21254, #21417, #31007, #2376, #7088, #11810, #21573, #171 ),
 .UNSPECIFIED., .F., .F.,
 ( 6, 3, 6 ),
 ( 0.000000000000000000, 0.7281981214720000262, 1.224410003600000074 ),
 .UNSPECIFIED. ) ;
#5556=CARTESIAN_POINT ( 'NONE',  ( -21.63136441776463315, 17.21881425927816878, 0.08279823700002575393 ) ) ;
#5566=CARTESIAN_POINT ( 'NONE',  ( 23.23955039760055641, 15.25661106415676471, 5.208368893000026034 ) ) ;
#5572=CARTESIAN_POINT ( 'NONE',  ( -27.03594125075309762, -0.4919295335570806893, -0.6999999999999784173 ) ) ;
#5578=CARTESIAN_POINT ( 'NONE',  ( 16.85920661228352557, -7.934045360712157269, -4.336808689942018722E-16 ) ) ;
#5586=CARTESIAN_POINT ( 'NONE',  ( 16.10001530720865759, -9.306175026709254894, -0.000000000000000000 ) ) ;
#5588=CARTESIAN_POINT ( 'NONE',  ( 23.68253874081223387, -20.17876519719180095, -0.2432540810000105580 ) ) ;
#5607=CARTESIAN_POINT ( 'NONE',  ( 23.47715715134837211, -20.00370206646827498, 1.000000001000006522 ) ) ;
#5614=CARTESIAN_POINT ( 'NONE',  ( -27.84772847483668912, 6.760385877827641110, 8.000000000000007105 ) ) ;
#5616=CARTESIAN_POINT ( 'NONE',  ( 24.98823331316959440, -13.70626928515100573, 6.095967861000000987 ) ) ;
#5621=ADVANCED_FACE ( 'NONE', ( #26387 ), #14281, .T. ) ;
#5645=ORIENTED_EDGE ( 'NONE', *, *, #19399, .F. ) ;
#5649=CARTESIAN_POINT ( 'NONE',  ( -25.77914833258148164, -15.40383343755785361, 1.000000000000000888 ) ) ;
#5650=CARTESIAN_POINT ( 'NONE',  ( -0.3637587985824408121, -27.79782236981992583, 5.677349366198735758 ) ) ;
#5658=CARTESIAN_POINT ( 'NONE',  ( -26.87967798701711786, 4.135222155429991275, -0.6999999999999784173 ) ) ;
#5663=EDGE_CURVE ( 'NONE', #17781, #4165, #10788, .T. ) ;
#5664=CARTESIAN_POINT ( 'NONE',  ( 17.18658402238548533, 9.900182044515950963, -0.6999999989999727834 ) ) ;
#5668=CARTESIAN_POINT ( 'NONE',  ( 24.26750084572334032, 13.69201430750461412, -0.6577119969999878357 ) ) ;
#5670=CARTESIAN_POINT ( 'NONE',  ( 27.51770821235203357, 4.728187301808492116, 1.000000000000000888 ) ) ;
#5672=CARTESIAN_POINT ( 'NONE',  ( 17.16657240421717390, -9.000000000001264766, -0.6999999999999784173 ) ) ;
#5681=VERTEX_POINT ( 'NONE', #29807 ) ;
#5685=CARTESIAN_POINT ( 'NONE',  ( -17.70061747254754181, -9.691892145441446615, -0.6999999999999783062 ) ) ;
#5686=CARTESIAN_POINT ( 'NONE',  ( 16.06675444876397307, -9.020011618195203695, -0.6999999999999784173 ) ) ;
#5689=LINE ( 'NONE', #19873, #16444 ) ;
#5690=CARTESIAN_POINT ( 'NONE',  ( -24.36725163762951851, -13.38201776504032381, 5.146975365592536988 ) ) ;
#5702=CARTESIAN_POINT ( 'NONE',  ( 1.783682052046414057, 3.046043134630439297, -0.6999999999999784173 ) ) ;
#5707=LINE ( 'NONE', #12952, #2257 ) ;
#5710=CARTESIAN_POINT ( 'NONE',  ( -24.24144457387483698, -14.48500828217274439, -0.6999999999999784173 ) ) ;
#5714=AXIS2_PLACEMENT_3D ( 'NONE', #12100, #17285, #21708 ) ;
#5717=VERTEX_POINT ( 'NONE', #16431 ) ;
#5721=CARTESIAN_POINT ( 'NONE',  ( -24.70074544867652122, 14.21822122508601716, 3.997190861000005313 ) ) ;
#5724=EDGE_CURVE ( 'NONE', #16061, #24893, #3195, .T. ) ;
#5725=CARTESIAN_POINT ( 'NONE',  ( 1.645560275461679600, -28.45273235262772005, 5.147476193076592210 ) ) ;
#5726=B_SPLINE_CURVE_WITH_KNOTS ( 'NONE', 3,
 ( #28802, #21737, #9462, #19064, #17156, #17011 ),
 .UNSPECIFIED., .F., .F.,
 ( 4, 2, 4 ),
 ( 0.000000000000000000, 0.5000000000000000000, 1.000000000000000000 ),
 .UNSPECIFIED. ) ;
#5727=B_SPLINE_CURVE_WITH_KNOTS ( 'NONE', 5,
 ( #15377, #27961, #1688, #27799, #18515, #6249, #25455, #6401, #10655 ),
 .UNSPECIFIED., .F., .F.,
 ( 6, 3, 6 ),
 ( -88.40979499649999696, -77.81866039000000512, -72.24467995679999888 ),
 .UNSPECIFIED. ) ;
#5728=CARTESIAN_POINT ( 'NONE',  ( -21.27524652179786457, 16.93536700441368126, -0.6999999999999784173 ) ) ;
#5733=CARTESIAN_POINT ( 'NONE',  ( 16.37473331892315542, -8.236461616552139375, 0.000000000000000000 ) ) ;
#5736=VERTEX_POINT ( 'NONE', #26040 ) ;
#5738=CARTESIAN_POINT ( 'NONE',  ( -23.85408962131194954, -14.27673465746016213, 6.098654221000004760 ) ) ;
#5742=CARTESIAN_POINT ( 'NONE',  ( 17.14656078599760392, 12.09981795542235439, -0.6999999989999727834 ) ) ;
#5743=CARTESIAN_POINT ( 'NONE',  ( -26.79556473285982321, -0.4875557887250224209, 0.000000000000000000 ) ) ;
#5745=CARTESIAN_POINT ( 'NONE',  ( -4.708590264754340282, -31.20269148734607256, -0.2432540810000105580 ) ) ;
#5748=EDGE_CURVE ( 'NONE', #14021, #14792, #23113, .T. ) ;
#5751=CARTESIAN_POINT ( 'NONE',  ( 0.4125558677674681096, -28.49726274111934998, 6.095949245000009675 ) ) ;
#5753=CARTESIAN_POINT ( 'NONE',  ( 24.98081130624543889, 13.71897605842228529, 4.999998581000003384 ) ) ;
#5760=ORIENTED_EDGE ( 'NONE', *, *, #13547, .F. ) ;
#5763=CARTESIAN_POINT ( 'NONE',  ( 13.88796284031055706, -26.65861513498057178, 0.02487559100000646950 ) ) ;
#5767=CARTESIAN_POINT ( 'NONE',  ( -22.90527192528401201, 16.36193184990112570, 5.200000000000009948 ) ) ;
#5772=CYLINDRICAL_SURFACE ( 'NONE', #29592, 1.099999999999999867 ) ;
#5786=B_SPLINE_CURVE_WITH_KNOTS ( 'NONE', 3,
 ( #4054, #23255, #1385, #10980, #30497, #6561 ),
 .UNSPECIFIED., .F., .F.,
 ( 4, 2, 4 ),
 ( 0.000000000000000000, 0.5000000000000000000, 1.000000000000000000 ),
 .UNSPECIFIED. ) ;
#5804=CARTESIAN_POINT ( 'NONE',  ( 24.43659368183839931, 14.66646236428692340, 3.899998581000013509 ) ) ;
#5806=CARTESIAN_POINT ( 'NONE',  ( 0.2237522039478089808, -27.79962635424878314, 6.073211979320773501 ) ) ;
#5813=CARTESIAN_POINT ( 'NONE',  ( -22.97723753882890918, 16.89265275057793403, 7.000000021000013284 ) ) ;
#5819=CARTESIAN_POINT ( 'NONE',  ( 14.60916111670818474, -28.04296597385482315, 1.000000000000000888 ) ) ;
#5822=CARTESIAN_POINT ( 'NONE',  ( 24.50249477284852517, 13.82460068605435666, -0.5592437529999827461 ) ) ;
#5823=CARTESIAN_POINT ( 'NONE',  ( 27.75695160380879045, 2.618790587931635994, 1.000000000000000888 ) ) ;
#5835=EDGE_LOOP ( 'NONE', ( #4195, #17599, #15897, #3887 ) ) ;
#5836=EDGE_CURVE ( 'NONE', #25912, #6569, #26119, .T. ) ;
#5844=CARTESIAN_POINT ( 'NONE',  ( -24.23284209150707369, -13.62399916074796202, 5.732688422242026682 ) ) ;
#5845=CARTESIAN_POINT ( 'NONE',  ( 19.80526555982327608, 19.50877392092707296, 0.9260799790000162623 ) ) ;
#5862=CARTESIAN_POINT ( 'NONE',  ( 26.97469346668950152, -9.357175201752722771, -0.6999999999999784173 ) ) ;
#5876=CARTESIAN_POINT ( 'NONE',  ( -27.64451936256318376, 4.252886846324511083, -0.5592437529999827461 ) ) ;
#5887=CARTESIAN_POINT ( 'NONE',  ( -24.47278419579111386, -14.60601539740217092, 6.095965388000001539 ) ) ;
#5889=CARTESIAN_POINT ( 'NONE',  ( 23.95030481189679605, 13.51304758006065043, 0.000000000000000000 ) ) ;
#5890=CARTESIAN_POINT ( 'NONE',  ( 16.40303402077768169, -9.791839085275103827, 0.000000000000000000 ) ) ;
#5896=CARTESIAN_POINT ( 'NONE',  ( 23.77947513710800109, -14.40125623032519719, 4.791564337000009388 ) ) ;
#5913=CARTESIAN_POINT ( 'NONE',  ( 13.96766655902600185, -26.81162144411387160, 0.08279888700002402402 ) ) ;
#5934=EDGE_CURVE ( 'NONE', #25869, #27389, #7332, .T. ) ;
#5936=DIRECTION ( 'NONE',  ( 0.000000000000000000, 0.000000000000000000, -1.000000000000000000 ) ) ;
#5940=CARTESIAN_POINT ( 'NONE',  ( 18.13765659380263884, -9.536403318364705228, -4.336808689942018722E-16 ) ) ;
#5953=CARTESIAN_POINT ( 'NONE',  ( 24.97472003062369694, 13.73006752330286595, 4.791638082000004850 ) ) ;
#5954=CARTESIAN_POINT ( 'NONE',  ( 16.06675444873834380, 10.97998838177521286, -1.000005633855494125E-09 ) ) ;
#5964=ORIENTED_EDGE ( 'NONE', *, *, #14825, .T. ) ;
#5974=CARTESIAN_POINT ( 'NONE',  ( 18.94276248278926289, 21.23709850769745699, 0.5017677510000262409 ) ) ;
#5981=CARTESIAN_POINT ( 'NONE',  ( 23.81776757409229361, 15.65134803726813217, 5.104183903999998329 ) ) ;
#5991=AXIS2_PLACEMENT_3D ( 'NONE', #20058, #1171, #12968 ) ;
#5998=CARTESIAN_POINT ( 'NONE',  ( -24.82164231762110163, 12.51999568251545369, 5.310645680000003921 ) ) ;
#5999=CARTESIAN_POINT ( 'NONE',  ( 0.1352650258312465548, -28.50015511220833986, 3.957670871000018575 ) ) ;
#6001=CARTESIAN_POINT ( 'NONE',  ( 23.80349752545914654, -14.36153883977784140, 4.640418250294272795 ) ) ;
#6027=ORIENTED_EDGE ( 'NONE', *, *, #26769, .T. ) ;
#6029=ORIENTED_EDGE ( 'NONE', *, *, #19187, .F. ) ;
#6030=CARTESIAN_POINT ( 'NONE',  ( -24.43008698341936835, 14.67811372381255630, 4.492876031000014869 ) ) ;
#6038=CARTESIAN_POINT ( 'NONE',  ( -24.95427444319612675, 13.76797446832583560, 3.899998581000013509 ) ) ;
#6039=ORIENTED_EDGE ( 'NONE', *, *, #19098, .F. ) ;
#6050=CARTESIAN_POINT ( 'NONE',  ( 24.47471931349485530, 13.80892463682978999, 0.2686738749999861842 ) ) ;
#6057=ORIENTED_EDGE ( 'NONE', *, *, #27575, .T. ) ;
#6060=B_SPLINE_CURVE_WITH_KNOTS ( 'NONE', 3,
 ( #17411, #3093, #13153, #907, #20100, #1211 ),
 .UNSPECIFIED., .F., .F.,
 ( 4, 2, 4 ),
 ( 0.000000000000000000, 0.5000000000000000000, 1.000000000000000000 ),
 .UNSPECIFIED. ) ;
#6063=CARTESIAN_POINT ( 'NONE',  ( 3.254826447334524087, -1.366018022763357376, -0.6999999999999783062 ) ) ;
#6068=VERTEX_POINT ( 'NONE', #22859 ) ;
#6071=CARTESIAN_POINT ( 'NONE',  ( -4.523585141650849017, -29.97671968535647835, 0.000000000000000000 ) ) ;
#6077=CARTESIAN_POINT ( 'NONE',  ( -27.16374144401319057, 6.594388859764479527, 8.000000000000007105 ) ) ;
#6078=CARTESIAN_POINT ( 'NONE',  ( -16.50769779712623730, -10.05824544944950105, 0.000000000000000000 ) ) ;
#6081=CARTESIAN_POINT ( 'NONE',  ( 25.77914806503467560, 15.40383291000323318, 1.000000000000000888 ) ) ;
#6087=LINE ( 'NONE', #30650, #23847 ) ;
#6092=CARTESIAN_POINT ( 'NONE',  ( 18.23252704358327847, 11.30736579158651445, -4.336808689942018722E-16 ) ) ;
#6119=CARTESIAN_POINT ( 'NONE',  ( 25.07525408169050607, -13.54704387006805533, 6.073823031490324098 ) ) ;
#6126=CARTESIAN_POINT ( 'NONE',  ( -20.77600556904588913, -21.68409854326813146, 1.000000000000000888 ) ) ;
#6130=CARTESIAN_POINT ( 'NONE',  ( 22.47598016381227737, 18.14223004260798078, 0.7595836940000044724 ) ) ;
#6165=CARTESIAN_POINT ( 'NONE',  ( 17.33115445853015046, 9.902812560049827795, -0.6999999999999783062 ) ) ;
#6168=CARTESIAN_POINT ( 'NONE',  ( 22.97559295455008765, 15.65128684778802715, 8.000000000000007105 ) ) ;
#6188=CARTESIAN_POINT ( 'NONE',  ( 24.39135169777336287, -14.74223403354865347, 5.310643619999999565 ) ) ;
#6200=CARTESIAN_POINT ( 'NONE',  ( -25.45799949038170240, 12.81261085762170815, 4.791562840999991302 ) ) ;
#6207=CARTESIAN_POINT ( 'NONE',  ( -23.80092421055088892, -14.36517094966330710, 6.099998581000020792 ) ) ;
#6208=CARTESIAN_POINT ( 'NONE',  ( 24.69145217640891232, 13.93120638769218367, 0.7069220679999932422 ) ) ;
#6214=CARTESIAN_POINT ( 'NONE',  ( 24.49145441566124148, -14.57548795709913847, 4.319167818000013703 ) ) ;
#6236=FACE_OUTER_BOUND ( 'NONE', #13002, .T. ) ;
#6238=CARTESIAN_POINT ( 'NONE',  ( 25.46368747440213198, -12.80129684534102807, 4.895780544000027490 ) ) ;
#6243=CARTESIAN_POINT ( 'NONE',  ( -28.49528339128749366, -0.5184828350247780993, 8.000000000000007105 ) ) ;
#6244=B_SPLINE_CURVE_WITH_KNOTS ( 'NONE', 1,
 ( #18878, #11491 ),
 .UNSPECIFIED., .F., .F.,
 ( 2, 2 ),
 ( -2.557520719980000135E-06, 0.7000000000009999335 ),
 .UNSPECIFIED. ) ;
#6248=CARTESIAN_POINT ( 'NONE',  ( -24.06826084733133797, 20.50742046740553093, 8.000000000000007105 ) ) ;
#6249=CARTESIAN_POINT ( 'NONE',  ( 24.71241344867332046, 12.80597785358207297, 8.000000000000007105 ) ) ;
#6254=CARTESIAN_POINT ( 'NONE',  ( -25.46368746804859740, 12.80129684245613575, 4.895780543000022078 ) ) ;
#6255=CARTESIAN_POINT ( 'NONE',  ( -26.79556473285982321, -0.4875557887250224209, 0.000000000000000000 ) ) ;
#6258=CARTESIAN_POINT ( 'NONE',  ( 27.79539923781684507, 0.5057481689249130330, 1.000000000000000888 ) ) ;
#6269=VERTEX_POINT ( 'NONE', #24566 ) ;
#6292=CARTESIAN_POINT ( 'NONE',  ( -27.22236205671638842, -6.258747753008545800, 8.000000000000007105 ) ) ;
#6294=CARTESIAN_POINT ( 'NONE',  ( 25.29825173858419873, 14.27357626363527920, 0.5017677510000262409 ) ) ;
#6318=CARTESIAN_POINT ( 'NONE',  ( 0.03635086285233400660, -28.50041301604787947, 3.997479608999987555 ) ) ;
#6323=ORIENTED_EDGE ( 'NONE', *, *, #10187, .F. ) ;
#6334=CARTESIAN_POINT ( 'NONE',  ( -17.93324555120827668, 10.97998838178171432, -0.6999999999999784173 ) ) ;
#6335=ORIENTED_EDGE ( 'NONE', *, *, #23334, .F. ) ;
#6338=ORIENTED_EDGE ( 'NONE', *, *, #19187, .T. ) ;
#6343=ORIENTED_EDGE ( 'NONE', *, *, #8047, .F. ) ;
#6349=VERTEX_POINT ( 'NONE', #23140 ) ;
#6380=ADVANCED_FACE ( 'NONE', ( #27842 ), #11435, .F. ) ;
#6382=DIRECTION ( 'NONE',  ( 0.000000000000000000, 0.000000000000000000, -1.000000000000000000 ) ) ;
#6396=CARTESIAN_POINT ( 'NONE',  ( -0.3775595308767857317, -28.49777658967402871, 4.319846982000025370 ) ) ;
#6401=CARTESIAN_POINT ( 'NONE',  ( 23.60106408278174328, 14.73312039574607901, 8.000000000000007105 ) ) ;
#6433=CARTESIAN_POINT ( 'NONE',  ( -16.17354070529352583, 11.89178602531050899, -4.336808689942018722E-16 ) ) ;
#6436=CARTESIAN_POINT ( 'NONE',  ( 25.45015930260169412, -12.82831286325064823, 5.290680261490429359 ) ) ;
#6443=CARTESIAN_POINT ( 'NONE',  ( -18.35216541603009688, -21.08443583241201935, 8.000000000000007105 ) ) ;
#6448=CARTESIAN_POINT ( 'NONE',  ( -17.93586506597758046, 11.12395421520594851, -4.336808689942017736E-16 ) ) ;
#6449=EDGE_CURVE ( 'NONE', #27396, #1557, #5425, .T. ) ;
#6458=VERTEX_POINT ( 'NONE', #14531 ) ;
#6488=CARTESIAN_POINT ( 'NONE',  ( -23.94793942741029724, -15.45149538080513452, 5.679609021710654737 ) ) ;
#6503=ORIENTED_EDGE ( 'NONE', *, *, #9442, .T. ) ;
#6513=EDGE_CURVE ( 'NONE', #30472, #3626, #6934, .T. ) ;
#6514=CARTESIAN_POINT ( 'NONE',  ( -20.12248395285567071, 20.00008950071413238, 0.3491021030798783231 ) ) ;
#6516=AXIS2_PLACEMENT_3D ( 'NONE', #2830, #19364, #21419 ) ;
#6527=CARTESIAN_POINT ( 'NONE',  ( -17.52404053647086002, -8.139513033930352748, 0.000000000000000000 ) ) ;
#6548=CARTESIAN_POINT ( 'NONE',  ( -3.350725639047746007, 1.107490566396344356, 0.000000000000000000 ) ) ;
#6550=CARTESIAN_POINT ( 'NONE',  ( -0.6094664100040195764, -28.49364619262437870, 4.999998581000003384 ) ) ;
#6557=CARTESIAN_POINT ( 'NONE',  ( -17.91528966515560484, -8.768795348586470695, 0.000000000000000000 ) ) ;
#6561=CARTESIAN_POINT ( 'NONE',  ( -16.06988921239048551, -8.208160914692745891, -0.6999999999999784173 ) ) ;
#6567=B_SPLINE_CURVE_WITH_KNOTS ( 'NONE', 3,
 ( #10098, #7421, #24420, #22371, #28978, #2552 ),
 .UNSPECIFIED., .F., .F.,
 ( 4, 2, 4 ),
 ( 0.000000000000000000, 0.5000000000000000000, 1.000000000000000000 ),
 .UNSPECIFIED. ) ;
#6569=VERTEX_POINT ( 'NONE', #15289 ) ;
#6570=B_SPLINE_CURVE_WITH_KNOTS ( 'NONE', 3,
 ( #17552, #24802, #23546, #23225, #25436, #6063, #1667, #4339, #21171, #1826, #25267, #25746, #16131, #23394, #11264, #11107, #11417, #18338 ),
 .UNSPECIFIED., .F., .F.,
 ( 4, 2, 2, 2, 2, 2, 2, 2, 4 ),
 ( 0.000000000000000000, 0.1250000000000000000, 0.2500000000000000000, 0.3750000000000000000, 0.5000000000000000000, 0.6250000000000000000, 0.7500000000000000000, 0.8750000000000000000, 1.000000000000000000 ),
 .UNSPECIFIED. ) ;
#6577=APPLICATION_CONTEXT ( 'automotive_design' ) ;
#6579=EDGE_CURVE ( 'NONE', #19663, #28945, #22318, .T. ) ;
#6598=CARTESIAN_POINT ( 'NONE',  ( 8.737549905436626574, -27.40075442753056478, 8.000000000000007105 ) ) ;
#6611=ORIENTED_EDGE ( 'NONE', *, *, #23730, .T. ) ;
#6615=EDGE_CURVE ( 'NONE', #26866, #22866, #830, .T. ) ;
#6622=CARTESIAN_POINT ( 'NONE',  ( 0.4478609109089253248, -28.49673184309138918, 3.901345920999998995 ) ) ;
#6627=ORIENTED_EDGE ( 'NONE', *, *, #795, .T. ) ;
#6635=CARTESIAN_POINT ( 'NONE',  ( -25.39337327098795072, 12.94027895355586288, 5.560810202636621291 ) ) ;
#6637=CARTESIAN_POINT ( 'NONE',  ( 23.83325788290921565, -14.31210125041407899, 5.496144292502794571 ) ) ;
#6642=CARTESIAN_POINT ( 'NONE',  ( -24.37821945910799926, 14.76389285725497125, 5.208432825000025801 ) ) ;
#6645=CARTESIAN_POINT ( 'NONE',  ( 0.6243462152986178904, -28.49342029039284085, 3.904048352000033528 ) ) ;
#6648=CARTESIAN_POINT ( 'NONE',  ( -24.25452752885752261, 13.58678145142700622, 3.899998581000042819 ) ) ;
#6666=CARTESIAN_POINT ( 'NONE',  ( -18.93738424706367951, 20.00019831485299093, -0.5298795608970631177 ) ) ;
#6672=CARTESIAN_POINT ( 'NONE',  ( -23.23277431133845994, -15.26692929363520257, 4.999998581000003384 ) ) ;
#6673=FACE_OUTER_BOUND ( 'NONE', #8686, .T. ) ;
#6676=CARTESIAN_POINT ( 'NONE',  ( -16.83342759582943060, -8.999999999996580513, -0.6999999999999784173 ) ) ;
#6678=CARTESIAN_POINT ( 'NONE',  ( 24.98081130624543889, 13.71897605842228529, 4.999998581000003384 ) ) ;
#6697=ORIENTED_EDGE ( 'NONE', *, *, #29829, .F. ) ;
#6703=CARTESIAN_POINT ( 'NONE',  ( -16.71067332636193115, -10.09794851200387278, 0.000000000000000000 ) ) ;
#6706=ORIENTED_EDGE ( 'NONE', *, *, #23158, .F. ) ;
#6707=CARTESIAN_POINT ( 'NONE',  ( 21.17669550445266680, 18.05242248062137023, 5.000000000000004441 ) ) ;
#6718=CARTESIAN_POINT ( 'NONE',  ( -27.79539923781770483, -0.5057481688778011630, 1.000000000000000888 ) ) ;
#6730=B_SPLINE_CURVE_WITH_KNOTS ( 'NONE', 3,
 ( #26367, #12494, #2300, #10145, #4813, #11883, #21487, #19744, #7162, #16749, #14408, #2449 ),
 .UNSPECIFIED., .F., .F.,
 ( 4, 2, 2, 2, 2, 4 ),
 ( 0.000000000000000000, 0.2500000000000005551, 0.5000000000000011102, 0.6250000000000004441, 0.7499999999999998890, 1.000000000000000000 ),
 .UNSPECIFIED. ) ;
#6736=CARTESIAN_POINT ( 'NONE',  ( -28.49528339128749366, -0.5184828350247674411, 1.000000000000000888 ) ) ;
#6737=CARTESIAN_POINT ( 'NONE',  ( -15.73360964037622622, -8.979988381802643360, -0.6999999999999784173 ) ) ;
#6764=ORIENTED_EDGE ( 'NONE', *, *, #27337, .T. ) ;
#6771=VERTEX_POINT ( 'NONE', #1908 ) ;
#6781=CARTESIAN_POINT ( 'NONE',  ( 23.57322167201500562, 14.73624931484498291, 3.997250016000014838 ) ) ;
#6782=DIRECTION ( 'NONE',  ( 0.000000000000000000, 0.000000000000000000, -1.000000000000000000 ) ) ;
#6784=CARTESIAN_POINT ( 'NONE',  ( 18.06290775522712977, 19.99992683950017636, -0.6936597257213343859 ) ) ;
#6793=FACE_BOUND ( 'NONE', #28632, .T. ) ;
#6801=ORIENTED_EDGE ( 'NONE', *, *, #18098, .F. ) ;
#6818=CARTESIAN_POINT ( 'NONE',  ( 28.45300238704230367, 0.5177135156027677931, 0.5017677510000262409 ) ) ;
#6821=CARTESIAN_POINT ( 'NONE',  ( -18.97090238746602964, 21.26865671882813302, 1.000000000000000888 ) ) ;
#6830=CARTESIAN_POINT ( 'NONE',  ( -23.24877830753397490, -15.24265806274975787, 4.710689436884310410 ) ) ;
#6831=CARTESIAN_POINT ( 'NONE',  ( 1.413941964909729787, -28.46527362969750996, 4.319830470999985295 ) ) ;
#6859=ORIENTED_EDGE ( 'NONE', *, *, #21955, .F. ) ;
#6860=CARTESIAN_POINT ( 'NONE',  ( 21.70992212615148986, 18.50697891487987334, 5.000000000000004441 ) ) ;
#6868=DIRECTION ( 'NONE',  ( 0.7198537139083028835, -0.6941258031311204890, 0.000000000000000000 ) ) ;
#6887=ORIENTED_EDGE ( 'NONE', *, *, #1804, .F. ) ;
#6897=ADVANCED_FACE ( 'NONE', ( #28645 ), #19518, .F. ) ;
#6899=CARTESIAN_POINT ( 'NONE',  ( 26.99674179536344099, 9.610833985112126499, 8.000000000000007105 ) ) ;
#6902=CARTESIAN_POINT ( 'NONE',  ( 22.83564165258658818, -19.45716463537533159, -0.6999999999999784173 ) ) ;
#6909=CARTESIAN_POINT ( 'NONE',  ( 0.4713258872182368164, -27.79624559782057602, 3.899998581000013509 ) ) ;
#6910=EDGE_CURVE ( 'NONE', #14792, #12633, #7794, .T. ) ;
#6929=CARTESIAN_POINT ( 'NONE',  ( -25.14597776469910428, -15.02549348198344603, 1.000000000000000888 ) ) ;
#6930=CARTESIAN_POINT ( 'NONE',  ( 23.62421573330318836, 14.65442405561991634, 3.957526369000014199 ) ) ;
#6934=B_SPLINE_CURVE_WITH_KNOTS ( 'NONE', 3,
 ( #23820, #12460, #24271, #4778, #9802, #16874 ),
 .UNSPECIFIED., .F., .F.,
 ( 4, 2, 4 ),
 ( 0.000000000000000000, 0.5000000000000000000, 1.000000000000000000 ),
 .UNSPECIFIED. ) ;
#6937=EDGE_CURVE ( 'NONE', #19859, #25327, #27302, .T. ) ;
#6949=CARTESIAN_POINT ( 'NONE',  ( -25.26019820782813596, 13.19871658270252723, 5.889015029569602433 ) ) ;
#6951=ADVANCED_FACE ( 'NONE', ( #24396 ), #14646, .F. ) ;
#6955=CARTESIAN_POINT ( 'NONE',  ( 1.311146135488785669, -27.76947565999227763, 5.759639119000015128 ) ) ;
#6958=CARTESIAN_POINT ( 'NONE',  ( -24.81746041937532965, 14.01353061208509310, 6.079865099000020479 ) ) ;
#6970=VERTEX_POINT ( 'NONE', #21575 ) ;
#6985=CARTESIAN_POINT ( 'NONE',  ( -20.19477874851248700, 20.00033066885824695, 0.4884133666381245131 ) ) ;
#6986=VECTOR ( 'NONE', #27795, 1000.000000000000000 ) ;
#7003=CARTESIAN_POINT ( 'NONE',  ( 16.40303402077768169, -9.791839085275103827, -0.6999999999999784173 ) ) ;
#7008=SURFACE_SIDE_STYLE ('',( #14406 ) ) ;
#7011=CARTESIAN_POINT ( 'NONE',  ( 1.592882851206511186, -27.75460863273100998, 4.791883387999989807 ) ) ;
#7013=CARTESIAN_POINT ( 'NONE',  ( 24.78575720336396415, -12.59082710992283793, 4.503870356536896047 ) ) ;
#7019=CARTESIAN_POINT ( 'NONE',  ( -19.80535357367646654, 19.50875577052770993, 2.600000086000031629 ) ) ;
#7020=CARTESIAN_POINT ( 'NONE',  ( -0.5575288593901739365, -27.79459983365126163, 4.689815098000011062 ) ) ;
#7033=CARTESIAN_POINT ( 'NONE',  ( -24.82162973577332465, 12.51998933601907993, 4.689351480999998323 ) ) ;
#7038=CARTESIAN_POINT ( 'NONE',  ( 24.47278418934494937, 14.60601539438439822, 6.095965388000001539 ) ) ;
#7040=CARTESIAN_POINT ( 'NONE',  ( 20.30396079662882158, 20.00000000004802203, 1.800000000000023803 ) ) ;
#7045=EDGE_CURVE ( 'NONE', #13976, #6970, #1460, .T. ) ;
#7046=ORIENTED_EDGE ( 'NONE', *, *, #15676, .F. ) ;
#7082=ORIENTED_EDGE ( 'NONE', *, *, #21478, .T. ) ;
#7088=CARTESIAN_POINT ( 'NONE',  ( -17.43456092915394251, -9.925215865042019914, 0.000000000000000000 ) ) ;
#7094=CARTESIAN_POINT ( 'NONE',  ( 18.49564307673682961, 20.00004823712628266, -0.6418581041093734951 ) ) ;
#7096=FACE_OUTER_BOUND ( 'NONE', #25011, .T. ) ;
#7118=CARTESIAN_POINT ( 'NONE',  ( 23.82471740507292068, 15.64077205896351508, 4.791628269000009155 ) ) ;
#7120=ORIENTED_EDGE ( 'NONE', *, *, #25464, .T. ) ;
#7123=B_SPLINE_CURVE_WITH_KNOTS ( 'NONE', 1,
 ( #16105, #1799 ),
 .UNSPECIFIED., .F., .F.,
 ( 2, 2 ),
 ( 1.257340418068942224E-07, 0.7036780443879999680 ),
 .UNSPECIFIED. ) ;
#7143=CARTESIAN_POINT ( 'NONE',  ( -23.38367611648533639, -15.03487154286002436, 4.267303388019339394 ) ) ;
#7144=CARTESIAN_POINT ( 'NONE',  ( 1.311146135404979818, -27.76947565989378219, 4.240358041999986227 ) ) ;
#7148=CARTESIAN_POINT ( 'NONE',  ( -16.85343921422224156, -7.900182044607009679, 0.000000000000000000 ) ) ;
#7155=CARTESIAN_POINT ( 'NONE',  ( -27.79960709041389677, 4.276745829942281141, 0.5514269430000329208 ) ) ;
#7157=B_SPLINE_CURVE_WITH_KNOTS ( 'NONE', 1,
 ( #11713, #28232 ),
 .UNSPECIFIED., .F., .F.,
 ( 2, 2 ),
 ( -2.555864960449999711E-06, 0.7000000000009999335 ),
 .UNSPECIFIED. ) ;
#7158=CARTESIAN_POINT ( 'NONE',  ( 24.41841038956698640, 14.69667349781389376, 6.099998581000020792 ) ) ;
#7162=CARTESIAN_POINT ( 'NONE',  ( 23.88383647311231428, 15.55037089993357746, 5.498277358143902838 ) ) ;
#7164=CARTESIAN_POINT ( 'NONE',  ( 23.76534794177020871, 14.42397062701149935, 6.095965061000018892 ) ) ;
#7190=CARTESIAN_POINT ( 'NONE',  ( 18.26905192736944983, 10.87373459873798609, -0.6999999999999784173 ) ) ;
#7195=ORIENTED_EDGE ( 'NONE', *, *, #12872, .F. ) ;
#7207=CARTESIAN_POINT ( 'NONE',  ( -16.04158851053540857, -9.763538383445707680, -0.6999999999999784173 ) ) ;
#7208=CARTESIAN_POINT ( 'NONE',  ( -27.79539923781684507, -0.5057481689249136991, 3.799999999999998046 ) ) ;
#7216=ORIENTED_EDGE ( 'NONE', *, *, #14083, .T. ) ;
#7220=CARTESIAN_POINT ( 'NONE',  ( 24.44014313072642963, -13.24968496497942105, 6.079865069000017996 ) ) ;
#7223=CARTESIAN_POINT ( 'NONE',  ( -19.99465714571108066, 19.99999931014700749, 0.1508170869999880814 ) ) ;
#7233=CARTESIAN_POINT ( 'NONE',  ( -17.64799051141838859, -8.260028345153997975, 0.000000000000000000 ) ) ;
#7236=ORIENTED_EDGE ( 'NONE', *, *, #26168, .T. ) ;
#7242=B_SPLINE_SURFACE_WITH_KNOTS ( 'NONE', 5, 5, ( 
 ( #29524, #20096, #3397, #22454, #7963, #29684, #13150, #17707, #22758 ),
 ( #17563, #1207, #27170, #15061, #8268, #5456, #27321, #27469, #29986 ),
 ( #24963, #15207, #8111, #13001, #12852, #3089, #18019, #24810, #5607 ),
 ( #10959, #27015, #5763, #5913, #27625, #15668, #904, #20553, #22612 ),
 ( #24656, #6071, #25279, #10644, #17408, #20236, #15514, #3712, #29831 ),
 ( #25120, #13313, #22924, #3246, #750, #30149, #1364, #11429, #11272 ),
 ( #25600, #4505, #8741, #1525, #21336, #23403, #4186, #23234, #9206 ),
 ( #28104, #21031, #8579, #30477, #30632, #26062, #2144, #8901, #11732 ),
 ( #9058, #18808, #18180, #25911, #4033, #14103, #18351, #4346, #15989 ) ),
 .UNSPECIFIED., .F., .F., .F.,
 ( 6, 3, 6 ),
 ( 6, 3, 6 ),
 ( 0.000000000000000000, 53.20205529499999386, 91.13698440880000362 ),
 ( 8.011061266649999624, 8.831591450809998634, 9.652121634960000307 ),
 .UNSPECIFIED. ) ;
#7246=CARTESIAN_POINT ( 'NONE',  ( 17.82602571120844459, 11.89215903477950853, -0.6999999999999783062 ) ) ;
#7248=CARTESIAN_POINT ( 'NONE',  ( -16.83342759582943060, -8.999999999996580513, -0.6999999999999784173 ) ) ;
#7251=CARTESIAN_POINT ( 'NONE',  ( -24.20792486932886689, 13.66932879934886813, 6.079865099000020479 ) ) ;
#7262=CARTESIAN_POINT ( 'NONE',  ( -2.374791981039476862, -2.610414167372405281, 0.000000000000000000 ) ) ;
#7263=CARTESIAN_POINT ( 'NONE',  ( 23.77947513710800109, -14.40125623032519719, 5.208432824000020389 ) ) ;
#7264=CARTESIAN_POINT ( 'NONE',  ( 19.65705194378976728, 20.00000012267804905, -0.1821635029999879585 ) ) ;
#7269=CARTESIAN_POINT ( 'NONE',  ( -24.31416968206321627, -13.47842985394946780, 4.493023692000025271 ) ) ;
#7272=CARTESIAN_POINT ( 'NONE',  ( 18.05835842950707359, 10.34011310949354367, -4.336808689942018722E-16 ) ) ;
#7280=VERTEX_POINT ( 'NONE', #8903 ) ;
#7282=EDGE_LOOP ( 'NONE', ( #22506, #5529, #3010, #6057 ) ) ;
#7290=CARTESIAN_POINT ( 'NONE',  ( 19.56389002122311638, 19.56882009050699622, 0.5006759800000037952 ) ) ;
#7301=CARTESIAN_POINT ( 'NONE',  ( -23.46764062199439493, -14.90374525705096254, 4.113458908961371563 ) ) ;
#7307=B_SPLINE_CURVE_WITH_KNOTS ( 'NONE', 1,
 ( #12219, #443 ),
 .UNSPECIFIED., .F., .F.,
 ( 2, 2 ),
 ( 1.500000000000000000, 3.500000000000000000 ),
 .UNSPECIFIED. ) ;
#7322=CARTESIAN_POINT ( 'NONE',  ( 0.5401834767574382745, -27.79499634052776358, 3.899998581000013509 ) ) ;
#7329=CARTESIAN_POINT ( 'NONE',  ( -23.78314118791541532, -14.39461388281431375, 3.901343066999990228 ) ) ;
#7332=B_SPLINE_CURVE_WITH_KNOTS ( 'NONE', 5,
 ( #2284, #29307, #11867, #2581, #9657, #21778 ),
 .UNSPECIFIED., .F., .F.,
 ( 6, 6 ),
 ( 71.86404503510000552, 94.75474465359999954 ),
 .UNSPECIFIED. ) ;
#7337=CARTESIAN_POINT ( 'NONE',  ( 21.02336020643863179, 19.26966202639587067, 4.000000000000003553 ) ) ;
#7339=CARTESIAN_POINT ( 'NONE',  ( -23.23277126416379801, -15.26692729116844482, 4.999998581000003384 ) ) ;
#7345=CARTESIAN_POINT ( 'NONE',  ( -16.83342759575507586, 10.99999999997565503, -0.6999999999999784173 ) ) ;
#7349=CARTESIAN_POINT ( 'NONE',  ( -16.06988964647317886, -8.208161364834239748, 0.000000000000000000 ) ) ;
#7350=CARTESIAN_POINT ( 'NONE',  ( 18.24356172875952709, 10.73282780903411293, -0.6999999999999784173 ) ) ;
#7379=CARTESIAN_POINT ( 'NONE',  ( -16.81341597763548990, -10.09981795544978311, -0.6999999989999727834 ) ) ;
#7390=ORIENTED_EDGE ( 'NONE', *, *, #9680, .F. ) ;
#7394=ORIENTED_EDGE ( 'NONE', *, *, #30316, .F. ) ;
#7403=CARTESIAN_POINT ( 'NONE',  ( -21.27524652179786457, 16.93536700441368126, -0.6999999999999784173 ) ) ;
#7408=CARTESIAN_POINT ( 'NONE',  ( 3.455601306038246001, 0.7156333712654180390, 0.000000000000000000 ) ) ;
#7410=CARTESIAN_POINT ( 'NONE',  ( -16.81341597784800967, -10.09981795476353739, 0.000000000000000000 ) ) ;
#7411=CARTESIAN_POINT ( 'NONE',  ( 19.06888577842656574, 19.69230313816537148, 0.2004941630000256492 ) ) ;
#7418=CARTESIAN_POINT ( 'NONE',  ( -24.00926694310947695, -14.01467022312833421, 3.957524336000023624 ) ) ;
#7420=VERTEX_POINT ( 'NONE', #12654 ) ;
#7421=CARTESIAN_POINT ( 'NONE',  ( 18.26375984360044313, -8.835417945884492141, -0.6999999999999783062 ) ) ;
#7425=CARTESIAN_POINT ( 'NONE',  ( -16.81341597756113515, 9.900182044522454206, -0.6999999999999784173 ) ) ;
#7434=CARTESIAN_POINT ( 'NONE',  ( 27.55801272791059731, 0.5014288284349769365, -0.5592437529999827461 ) ) ;
#7452=CARTESIAN_POINT ( 'NONE',  ( -24.73806702658698953, 12.68469578970483269, 4.322438790421920807 ) ) ;
#7460=CARTESIAN_POINT ( 'NONE',  ( -27.08859402333790456, -0.4928875713652468016, 0.02487529600000981667 ) ) ;
#7462=CARTESIAN_POINT ( 'NONE',  ( 23.80092420482279891, 14.36517094565843777, 6.099998581000020792 ) ) ;
#7475=B_SPLINE_CURVE_WITH_KNOTS ( 'NONE', 3,
 ( #2428, #12019, #77, #9655, #19258, #16270 ),
 .UNSPECIFIED., .F., .F.,
 ( 4, 2, 4 ),
 ( 0.000000000000000000, 0.5000000000000000000, 1.000000000000000000 ),
 .UNSPECIFIED. ) ;
#7478=CARTESIAN_POINT ( 'NONE',  ( -24.29089620838935204, -14.90695587844356673, 3.920145809000019632 ) ) ;
#7484=CARTESIAN_POINT ( 'NONE',  ( -15.75699695929680821, 10.73161574548146824, -1.384526174263989162E-13 ) ) ;
#7492=CARTESIAN_POINT ( 'NONE',  ( -25.77914833258148164, -15.40383343755785361, 0.7595836940000044724 ) ) ;
#7494=CARTESIAN_POINT ( 'NONE',  ( -20.77600556914587315, -21.68409854326995045, 8.000000000000007105 ) ) ;
#7499=CARTESIAN_POINT ( 'NONE',  ( -16.83342759575507586, 10.99999999997565503, -0.6999999999999784173 ) ) ;
#7508=ADVANCED_FACE ( 'NONE', ( #20205 ), #18146, .F. ) ;
#7514=CARTESIAN_POINT ( 'NONE',  ( -23.92481352202682388, 14.15879617723574313, 4.239732039000021047 ) ) ;
#7522=CARTESIAN_POINT ( 'NONE',  ( -24.45473033751197178, -14.63622298155413226, 3.901342939999996595 ) ) ;
#7527=B_SPLINE_SURFACE_WITH_KNOTS ( 'NONE', 5, 1, ( 
 ( #24881, #27387 ),
 ( #5981, #8173 ),
 ( #22983, #3310 ),
 ( #25182, #22667 ),
 ( #1430, #11024 ),
 ( #30056, #29904 ),
 ( #15575, #30211 ),
 ( #3616, #22524 ),
 ( #8644, #13210 ),
 ( #18241, #27852 ),
 ( #22823, #20302 ),
 ( #20154, #8327 ),
 ( #1275, #10872 ),
 ( #17623, #7462 ),
 ( #7158, #12178 ) ),
 .UNSPECIFIED., .F., .F., .F.,
 ( 6, 3, 3, 3, 6 ),
 ( 2, 2 ),
 ( 0.000000000000000000, 0.5238999881950000548, 1.047799976390000110, 1.571699964580000053, 1.746333293980000034 ),
 ( -0.7000000000009999335, 2.555885125540000124E-06 ),
 .UNSPECIFIED. ) ;
#7530=CARTESIAN_POINT ( 'NONE',  ( -15.83793381061078875, -8.512024964203421362, 0.000000000000000000 ) ) ;
#7542=CARTESIAN_POINT ( 'NONE',  ( 24.54884435356041905, -13.04717673660012522, 3.997190761000024573 ) ) ;
#7562=CARTESIAN_POINT ( 'NONE',  ( 3.361572482953519625, 1.073845131765873484, 0.000000000000000000 ) ) ;
#7564=CARTESIAN_POINT ( 'NONE',  ( 23.81866173088643635, 14.33570044285385947, 6.099998581000020792 ) ) ;
#7567=B_SPLINE_CURVE_WITH_KNOTS ( 'NONE', 3,
 ( #16350, #23287, #26115, #16195, #25960, #30369, #25809, #30527, #24177, #13843 ),
 .UNSPECIFIED., .F., .F.,
 ( 4, 2, 2, 2, 4 ),
 ( 0.000000000000000000, 0.2500000000000000000, 0.5000000000000000000, 0.7500000000000000000, 1.000000000000000000 ),
 .UNSPECIFIED. ) ;
#7569=CARTESIAN_POINT ( 'NONE',  ( -24.43659368756648576, -14.66646236829179450, 3.899998581000013509 ) ) ;
#7575=VERTEX_POINT ( 'NONE', #15334 ) ;
#7581=EDGE_LOOP ( 'NONE', ( #5169, #26566, #29104, #30158, #25041, #10558, #14365, #10874 ) ) ;
#7588=CARTESIAN_POINT ( 'NONE',  ( 28.49528339128749366, 0.5184828350247753237, 8.000000000000007105 ) ) ;
#7595=ORIENTED_EDGE ( 'NONE', *, *, #22132, .F. ) ;
#7602=CARTESIAN_POINT ( 'NONE',  ( 0.6090474298383116158, -27.79358669172298946, 3.904048352000033528 ) ) ;
#7605=CARTESIAN_POINT ( 'NONE',  ( -3.496762477156740268, 0.4822370985009253319, -0.6999999999999784173 ) ) ;
#7611=CARTESIAN_POINT ( 'NONE',  ( -22.06913545133442511, 17.56725181239296774, 0.9999999989999952543 ) ) ;
#7615=B_SPLINE_SURFACE_WITH_KNOTS ( 'NONE', 5, 1, ( 
 ( #26610, #17464 ),
 ( #19845, #12290 ),
 ( #2842, #7263 ),
 ( #12435, #5196 ),
 ( #4901, #28967 ),
 ( #9931, #10241 ),
 ( #29119, #5050 ),
 ( #27070, #22054 ),
 ( #37, #10089 ),
 ( #15113, #26921 ),
 ( #19683, #29268 ),
 ( #5358, #14962 ),
 ( #24710, #16854 ),
 ( #654, #29426 ),
 ( #7860, #3146 ) ),
 .UNSPECIFIED., .F., .F., .F.,
 ( 6, 3, 3, 3, 6 ),
 ( 2, 2 ),
 ( 0.000000000000000000, 0.5239055192570000186, 1.047811038520000126, 1.571716557770000078, 1.746351730860000062 ),
 ( -0.7000000000009999335, 2.557314091049999969E-06 ),
 .UNSPECIFIED. ) ;
#7623=B_SPLINE_CURVE_WITH_KNOTS ( 'NONE', 5,
 ( #22976, #16045, #13526, #28158, #30203, #30833, #25810, #30528, #1580, #18231, #23138, #16351, #25657, #23609, #26116 ),
 .UNSPECIFIED., .F., .F.,
 ( 6, 3, 3, 3, 6 ),
 ( 0.000000000000000000, 0.1999999999996538436, 0.4000000000006923018, 0.6999999999986153965, 1.000000000000000000 ),
 .UNSPECIFIED. ) ;
#7635=CARTESIAN_POINT ( 'NONE',  ( 28.49528339128749366, 0.5184828350247753237, 8.000000000000007105 ) ) ;
#7637=CARTESIAN_POINT ( 'NONE',  ( -24.09747192797636828, -13.86256885946331430, 4.035710821950520888 ) ) ;
#7640=CARTESIAN_POINT ( 'NONE',  ( -20.44304571761251665, -21.33658544107177590, -0.2432540810000105580 ) ) ;
#7646=FACE_OUTER_BOUND ( 'NONE', #17212, .T. ) ;
#7656=ADVANCED_FACE ( 'NONE', ( #1956 ), #11550, .F. ) ;
#7659=CARTESIAN_POINT ( 'NONE',  ( -22.90527192528401201, 16.36193184990112570, 1.000000000000000888 ) ) ;
#7661=CARTESIAN_POINT ( 'NONE',  ( 25.16696686177538567, -13.37570800333111087, 6.002806400000004317 ) ) ;
#7663=CARTESIAN_POINT ( 'NONE',  ( -4.667733413567799694, -30.93201666733562405, 8.000000000000007105 ) ) ;
#7666=CARTESIAN_POINT ( 'NONE',  ( -24.83401023410189623, -13.98326748962921329, 4.239871886000001311 ) ) ;
#7684=CARTESIAN_POINT ( 'NONE',  ( 25.41286869299526074, -12.90211872965451079, 4.492873455000018446 ) ) ;
#7686=ORIENTED_EDGE ( 'NONE', *, *, #6579, .T. ) ;
#7692=ORIENTED_EDGE ( 'NONE', *, *, #9169, .T. ) ;
#7698=CARTESIAN_POINT ( 'NONE',  ( 22.62517538422034136, 16.36045799713766158, 1.000000000000000888 ) ) ;
#7710=FACE_OUTER_BOUND ( 'NONE', #18304, .T. ) ;
#7717=CARTESIAN_POINT ( 'NONE',  ( 1.379247882482921517, -27.76613141686462782, 5.680166690000016061 ) ) ;
#7718=CARTESIAN_POINT ( 'NONE',  ( -24.66346748855670867, -14.28208995890320665, 3.997248602000014195 ) ) ;
#7741=CARTESIAN_POINT ( 'NONE',  ( 28.49528339128749366, 0.5184828350247835393, 8.000000000000007105 ) ) ;
#7746=CARTESIAN_POINT ( 'NONE',  ( -17.93324555128263142, -9.020011618190519442, -0.6999999999999784173 ) ) ;
#7750=CARTESIAN_POINT ( 'NONE',  ( -24.41841039498785193, -14.69667350221323865, 6.099998581000020792 ) ) ;
#7752=CARTESIAN_POINT ( 'NONE',  ( -24.46167596951645251, 13.21010012949721535, 3.927763967234794595 ) ) ;
#7753=EDGE_CURVE ( 'NONE', #26866, #4633, #26309, .T. ) ;
#7762=AXIS2_PLACEMENT_3D ( 'NONE', #7499, #12068, #26544 ) ;
#7765=CARTESIAN_POINT ( 'NONE',  ( -24.05392374927932053, 13.13253365033636477, 0.000000000000000000 ) ) ;
#7772=CARTESIAN_POINT ( 'NONE',  ( 23.29312071241426096, 15.17488100587054767, 5.506989593000027661 ) ) ;
#7773=ORIENTED_EDGE ( 'NONE', *, *, #16488, .F. ) ;
#7778=AXIS2_PLACEMENT_3D ( 'NONE', #1196, #29672, #8102 ) ;
#7787=CARTESIAN_POINT ( 'NONE',  ( -24.36130770023045145, -13.39283555876519749, 5.208359076000035337 ) ) ;
#7794=B_SPLINE_CURVE_WITH_KNOTS ( 'NONE', 3,
 ( #24233, #7246, #16840, #26445, #28489, #335 ),
 .UNSPECIFIED., .F., .F.,
 ( 4, 2, 4 ),
 ( 0.000000000000000000, 0.5000000000000000000, 1.000000000000000000 ),
 .UNSPECIFIED. ) ;
#7795=CARTESIAN_POINT ( 'NONE',  ( -26.79556473285982321, -0.4875557887251147915, -0.6999999999999784173 ) ) ;
#7802=CARTESIAN_POINT ( 'NONE',  ( -0.5575288593801756010, -27.79459983365108044, 5.310182064000024127 ) ) ;
#7816=LINE ( 'NONE', #16798, #442 ) ;
#7824=CARTESIAN_POINT ( 'NONE',  ( 24.92639507930385889, 13.81781707913292934, 4.493023686000019445 ) ) ;
#7826=CARTESIAN_POINT ( 'NONE',  ( 27.73177268570753640, 2.208741748110918390, 8.000000000000007105 ) ) ;
#7835=ORIENTED_EDGE ( 'NONE', *, *, #14700, .F. ) ;
#7838=CARTESIAN_POINT ( 'NONE',  ( 24.34137756859324853, -13.42980563341176037, 3.899998581000013509 ) ) ;
#7845=ORIENTED_EDGE ( 'NONE', *, *, #8063, .F. ) ;
#7847=CARTESIAN_POINT ( 'NONE',  ( -20.77600556904588913, -21.68409854326813146, 1.000000000000000888 ) ) ;
#7849=CARTESIAN_POINT ( 'NONE',  ( 21.28666574344908469, 18.00484885041732142, 8.000000000000007105 ) ) ;
#7860=CARTESIAN_POINT ( 'NONE',  ( 24.93720649360215802, -13.79881813812812297, 6.099998581000020792 ) ) ;
#7862=CARTESIAN_POINT ( 'NONE',  ( 18.03085807409719621, 20.00000000003992540, -0.6999999999999784173 ) ) ;
#7875=CARTESIAN_POINT ( 'NONE',  ( 0.5057536231481327693, -27.79562098839016571, 3.899998581000013509 ) ) ;
#7879=ORIENTED_EDGE ( 'NONE', *, *, #18098, .T. ) ;
#7904=CARTESIAN_POINT ( 'NONE',  ( -3.529820002201436324, 0.01646793492178095022, -0.6999999999999783062 ) ) ;
#7912=CARTESIAN_POINT ( 'NONE',  ( -24.87718597855597125, 13.58193782283921536, 0.5514320120000304470 ) ) ;
#7921=B_SPLINE_CURVE_WITH_KNOTS ( 'NONE', 1,
 ( #20413, #921 ),
 .UNSPECIFIED., .F., .F.,
 ( 2, 2 ),
 ( 1.500000000000000000, 3.500000000000000000 ),
 .UNSPECIFIED. ) ;
#7927=CARTESIAN_POINT ( 'NONE',  ( -28.58473218748631339, 4.397531023511127124, 0.7595836940000044724 ) ) ;
#7934=CARTESIAN_POINT ( 'NONE',  ( 24.74993095443131352, -14.13250376055072266, 3.957489350000009676 ) ) ;
#7938=CARTESIAN_POINT ( 'NONE',  ( -24.36724936496760918, -13.38201651699120021, 4.999998581000003384 ) ) ;
#7939=CARTESIAN_POINT ( 'NONE',  ( -22.97723753882890918, 16.89265275057793403, 7.000000021000013284 ) ) ;
#7945=CARTESIAN_POINT ( 'NONE',  ( 13.73773747404255552, -26.37022765825810922, -0.6999999999999784173 ) ) ;
#7950=CARTESIAN_POINT ( 'NONE',  ( 0.2722179827725955126, -28.49915599500044650, 6.079792140000011891 ) ) ;
#7951=VERTEX_POINT ( 'NONE', #24401 ) ;
#7963=CARTESIAN_POINT ( 'NONE',  ( 27.52676963214367944, 0.5008603480904590954, 0.2686740700000300741 ) ) ;
#7965=VERTEX_POINT ( 'NONE', #26450 ) ;
#7968=CARTESIAN_POINT ( 'NONE',  ( -19.80535357367646654, 19.50875577052770993, 8.000000000000007105 ) ) ;
#7988=ADVANCED_FACE ( 'NONE', ( #2384 ), #18712, .F. ) ;
#7997=EDGE_LOOP ( 'NONE', ( #5760, #17935, #24723, #4487 ) ) ;
#8002=CARTESIAN_POINT ( 'NONE',  ( -4.785279987089964493, -31.71089578132167119, 1.000000000000000888 ) ) ;
#8012=CARTESIAN_POINT ( 'NONE',  ( -19.80535357367646654, 19.50875577052770993, 3.000000106999994642 ) ) ;
#8016=DIRECTION ( 'NONE',  ( 0.000000000000000000, 0.000000000000000000, -1.000000000000000000 ) ) ;
#8018=CARTESIAN_POINT ( 'NONE',  ( 18.41918092979155119, 20.00000737198188716, -0.6632381549999954995 ) ) ;
#8020=CARTESIAN_POINT ( 'NONE',  ( 27.79539923781684507, 0.5057481689249235801, 8.000000000000007105 ) ) ;
#8023=CARTESIAN_POINT ( 'NONE',  ( 0.5746121234326042604, -27.79431838510023312, 6.098651075000017130 ) ) ;
#8025=CARTESIAN_POINT ( 'NONE',  ( -0.5944614571882205212, -27.79380703160649446, 4.999998581000003384 ) ) ;
#8038=CARTESIAN_POINT ( 'NONE',  ( 16.89916710682537371, -10.07620797776944777, -0.000000000000000000 ) ) ;
#8043=CARTESIAN_POINT ( 'NONE',  ( -24.32472894358752313, 13.45989150749028873, 6.099998581000020792 ) ) ;
#8045=CARTESIAN_POINT ( 'NONE',  ( -14.60916135985672071, 28.04296594682689658, 1.000000000000000888 ) ) ;
#8047=EDGE_CURVE ( 'NONE', #14390, #13946, #28920, .T. ) ;
#8049=B_SPLINE_CURVE_WITH_KNOTS ( 'NONE', 5,
 ( #4038, #13636, #18508, #23241, #10809, #28110, #6548, #25284, #11434, #16145, #30638, #9063, #20403, #29990, #15672, #13317, #8424, #22928, #1369, #10964, #219 ),
 .UNSPECIFIED., .F., .F.,
 ( 6, 3, 3, 3, 3, 3, 6 ),
 ( -15.54987830269999982, -12.96130453750000022, -10.36904362289999959, -7.776782722830000161, -5.184521831730000585, -2.592260920730000251, 0.000000000000000000 ),
 .UNSPECIFIED. ) ;
#8057=CARTESIAN_POINT ( 'NONE',  ( 0.01646793492177278315, 3.529820002201416784, -0.6999999999999783062 ) ) ;
#8063=EDGE_CURVE ( 'NONE', #28983, #14390, #24415, .T. ) ;
#8066=CARTESIAN_POINT ( 'NONE',  ( -4.499842235593497719, -29.81936866046843093, -0.6999999999999784173 ) ) ;
#8073=CARTESIAN_POINT ( 'NONE',  ( 23.39354070784786543, 15.01969649483752001, 5.760134169000008519 ) ) ;
#8079=CARTESIAN_POINT ( 'NONE',  ( -27.17149341551030162, 9.183264753288028714, -0.2432540810000105580 ) ) ;
#8096=CARTESIAN_POINT ( 'NONE',  ( -28.49528339128749366, -0.5184828350247674411, 1.000000000000000888 ) ) ;
#8102=DIRECTION ( 'NONE',  ( -0.6941258031311203780, -0.7198537139083029945, 0.000000000000000000 ) ) ;
#8111=CARTESIAN_POINT ( 'NONE',  ( 22.88013437149966833, -19.49504814935155039, 0.02487579700000130956 ) ) ;
#8112=ORIENTED_EDGE ( 'NONE', *, *, #11935, .F. ) ;
#8114=CARTESIAN_POINT ( 'NONE',  ( 25.46368747440213198, -12.80129684534102807, 4.999998581000003384 ) ) ;
#8117=CARTESIAN_POINT ( 'NONE',  ( -27.62819771675075486, 4.248502122600195996, 8.000000000000007105 ) ) ;
#8143=ORIENTED_EDGE ( 'NONE', *, *, #15472, .T. ) ;
#8146=B_SPLINE_CURVE_WITH_KNOTS ( 'NONE', 3,
 ( #15640, #19909, #5578, #25251, #29655, #5733 ),
 .UNSPECIFIED., .F., .F.,
 ( 4, 2, 4 ),
 ( 0.000000000000000000, 0.5000000000000000000, 1.000000000000000000 ),
 .UNSPECIFIED. ) ;
#8170=CARTESIAN_POINT ( 'NONE',  ( 19.80526555962148549, 19.50877392102342256, 1.000000000000000888 ) ) ;
#8173=CARTESIAN_POINT ( 'NONE',  ( 23.23277125981546476, 15.26692728828886025, 5.104183903999998329 ) ) ;
#8177=B_SPLINE_CURVE_WITH_KNOTS ( 'NONE', 3,
 ( #17233, #6165, #15766, #25380, #3817, #13404 ),
 .UNSPECIFIED., .F., .F.,
 ( 4, 2, 4 ),
 ( 0.000000000000000000, 0.5000000000000000000, 1.000000000000000000 ),
 .UNSPECIFIED. ) ;
#8181=ORIENTED_EDGE ( 'NONE', *, *, #22299, .F. ) ;
#8187=CARTESIAN_POINT ( 'NONE',  ( -16.85343921394901301, 12.09981795542885585, -0.6999999999999784173 ) ) ;
#8191=CARTESIAN_POINT ( 'NONE',  ( -0.3775595308337927891, -28.49777658967324356, 5.680150179000031940 ) ) ;
#8213=CARTESIAN_POINT ( 'NONE',  ( -24.90119785323401302, 12.82531120033124594, 8.000000000000007105 ) ) ;
#8227=CARTESIAN_POINT ( 'NONE',  ( 16.40303402075260308, 10.20816091466531716, 0.000000000000000000 ) ) ;
#8232=CARTESIAN_POINT ( 'NONE',  ( -25.46368746804859740, 12.80129684245613575, 4.895780543000022078 ) ) ;
#8239=CARTESIAN_POINT ( 'NONE',  ( 16.47629287236006590, -8.131162914937760888, -0.6999999999999784173 ) ) ;
#8242=CARTESIAN_POINT ( 'NONE',  ( -23.78314118801539934, -14.39461388281613097, 6.098654095000016540 ) ) ;
#8244=CARTESIAN_POINT ( 'NONE',  ( 25.72310959295360533, 9.312057329555777585, 0.000000000000000000 ) ) ;
#8252=ADVANCED_FACE ( 'NONE', ( #16646 ), #25760, .F. ) ;
#8257=CARTESIAN_POINT ( 'NONE',  ( 0.4831567132655384955, -28.49614615030703391, 6.099998581000020792 ) ) ;
#8267=ORIENTED_EDGE ( 'NONE', *, *, #28720, .T. ) ;
#8268=CARTESIAN_POINT ( 'NONE',  ( 27.71078648026139390, -9.612516398576929078, 0.2686740700000300741 ) ) ;
#8274=MECHANICAL_DESIGN_GEOMETRIC_PRESENTATION_REPRESENTATION('',(#272),#28405);
#8293=CARTESIAN_POINT ( 'NONE',  ( 17.95841148951064525, -9.763538383420391042, 0.000000000000000000 ) ) ;
#8305=ORIENTED_EDGE ( 'NONE', *, *, #19824, .F. ) ;
#8306=CARTESIAN_POINT ( 'NONE',  ( 24.25742563242670613, 13.58028021435546684, 4.319317656000021266 ) ) ;
#8315=CARTESIAN_POINT ( 'NONE',  ( -16.04158851046123502, 10.23646161653652875, 0.000000000000000000 ) ) ;
#8319=CARTESIAN_POINT ( 'NONE',  ( 17.99591112602217891, 19.96082062028142090, 0.000000000000000000 ) ) ;
#8320=CARTESIAN_POINT ( 'NONE',  ( -20.77600556914587315, -21.68409854326995045, 8.000000000000007105 ) ) ;
#8327=CARTESIAN_POINT ( 'NONE',  ( 23.76534794177020871, 14.42397062701149935, 6.095965061000018892 ) ) ;
#8345=LINE ( 'NONE', #17941, #26001 ) ;
#8346=ADVANCED_FACE ( 'NONE', ( #14918 ), #4399, .T. ) ;
#8354=CARTESIAN_POINT ( 'NONE',  ( -17.93590711870954379, -8.873734598641418003, -0.6999999999999784173 ) ) ;
#8373=ORIENTED_EDGE ( 'NONE', *, *, #2023, .F. ) ;
#8375=VERTEX_POINT ( 'NONE', #29692 ) ;
#8379=CARTESIAN_POINT ( 'NONE',  ( -24.37821945910799926, 14.76389285725497125, 4.791564337000009388 ) ) ;
#8385=CARTESIAN_POINT ( 'NONE',  ( 16.21708932071647524, 10.42683423810934862, -0.000000000000000000 ) ) ;
#8394=CARTESIAN_POINT ( 'NONE',  ( 16.59368952254167340, -8.049650370620115680, -0.6999999999999784173 ) ) ;
#8395=CARTESIAN_POINT ( 'NONE',  ( -22.36193249936582816, 17.71394520520996707, 6.000000042999998229 ) ) ;
#8396=CARTESIAN_POINT ( 'NONE',  ( 18.13790330320517086, 20.33475721090277233, 0.08279788800003018423 ) ) ;
#8401=FACE_OUTER_BOUND ( 'NONE', #17485, .T. ) ;
#8408=CARTESIAN_POINT ( 'NONE',  ( -0.5716039299945605556, -28.49445895580190324, 5.310182064000024127 ) ) ;
#8424=CARTESIAN_POINT ( 'NONE',  ( 1.790201522669007561, 3.063245535112757434, 0.000000000000000000 ) ) ;
#8453=VERTEX_POINT ( 'NONE', #30320 ) ;
#8459=EDGE_CURVE ( 'NONE', #16870, #29062, #4118, .T. ) ;
#8460=CARTESIAN_POINT ( 'NONE',  ( -17.93324555108848628, -9.020011617866936504, 0.000000000000000000 ) ) ;
#8479=FACE_OUTER_BOUND ( 'NONE', #4477, .T. ) ;
#8489=ORIENTED_EDGE ( 'NONE', *, *, #22964, .T. ) ;
#8507=CARTESIAN_POINT ( 'NONE',  ( 23.77307027441306531, -14.41181805765238444, 4.999998581000003384 ) ) ;
#8512=B_SPLINE_CURVE_WITH_KNOTS ( 'NONE', 5,
 ( #8025, #1740, #20769, #11173, #20931, #21091, #28163, #27848, #8964, #1426, #30686, #23459, #18236, #6909, #21241 ),
 .UNSPECIFIED., .F., .F.,
 ( 6, 3, 3, 3, 6 ),
 ( 0.000000000000000000, 0.5239017171269999551, 1.047803434249999999, 1.571705151379999998, 1.746339057089999924 ),
 .UNSPECIFIED. ) ;
#8516=CARTESIAN_POINT ( 'NONE',  ( -23.48198671369468116, 16.77395784647688970, 1.000000000000000888 ) ) ;
#8541=CARTESIAN_POINT ( 'NONE',  ( 17.16657240419154462, 10.99999999996915179, -0.6999999999999784173 ) ) ;
#8550=CARTESIAN_POINT ( 'NONE',  ( -24.93720648713954446, 13.79881813474513486, 3.899998581000013509 ) ) ;
#8557=CARTESIAN_POINT ( 'NONE',  ( -24.05769994060051786, -13.93129956160059102, 6.002748559000014694 ) ) ;
#8558=CARTESIAN_POINT ( 'NONE',  ( -23.76534794678204321, -14.42397063190348483, 6.095965061000018892 ) ) ;
#8559=CARTESIAN_POINT ( 'NONE',  ( 21.13530760622424864, 17.06006193249097436, 0.000000000000000000 ) ) ;
#8560=B_SPLINE_CURVE_WITH_KNOTS ( 'NONE', 5,
 ( #26212, #28571, #25753, #21490, #9056, #23554, #31087, #4646, #28251 ),
 .UNSPECIFIED., .F., .F.,
 ( 6, 3, 6 ),
 ( 0.000000000000000000, 18.10919428740000114, 32.96201648640000315 ),
 .UNSPECIFIED. ) ;
#8566=CARTESIAN_POINT ( 'NONE',  ( 24.92013865993870425, -13.82966158318416738, 3.899998581000013509 ) ) ;
#8569=CARTESIAN_POINT ( 'NONE',  ( 26.56187606716263971, 4.248286909032550795, -0.6999999999999784173 ) ) ;
#8571=AXIS2_PLACEMENT_3D ( 'NONE', #24031, #2164, #6868 ) ;
#8579=CARTESIAN_POINT ( 'NONE',  ( -26.95947219337181266, -7.589290548446620654, 0.02487529600000981667 ) ) ;
#8581=CARTESIAN_POINT ( 'NONE',  ( 16.19548821478059963, -8.463596681405142874, -4.336808689942018722E-16 ) ) ;
#8599=CARTESIAN_POINT ( 'NONE',  ( -25.46368746804859740, 12.80129684245613575, 4.999998581000003384 ) ) ;
#8600=CARTESIAN_POINT ( 'NONE',  ( 26.97469346668950152, -9.357175201752722771, 0.000000000000000000 ) ) ;
#8602=CARTESIAN_POINT ( 'NONE',  ( 27.77052805885498898, 0.5052956280874453254, 0.7069222069999991920 ) ) ;
#8605=B_SPLINE_CURVE_WITH_KNOTS ( 'NONE', 5,
 ( #2301, #31085, #9525, #7164, #12647, #29646, #12963, #26976, #8073, #20358, #7772, #15329, #5566, #24771, #17669 ),
 .UNSPECIFIED., .F., .F.,
 ( 6, 3, 3, 3, 6 ),
 ( 0.000000000000000000, 0.1000000000011452422, 0.3999999999988547161, 0.6999999999994274136, 1.000000000000000000 ),
 .UNSPECIFIED. ) ;
#8634=CARTESIAN_POINT ( 'NONE',  ( 27.29371452669260734, 0.4966198192113280285, -0.6577119969999878357 ) ) ;
#8636=CARTESIAN_POINT ( 'NONE',  ( -23.76243112480983655, -16.20069438324207667, 8.000000000000007105 ) ) ;
#8644=CARTESIAN_POINT ( 'NONE',  ( 24.16679028237082960, 15.10730797463399000, 6.002747145999992817 ) ) ;
#8658=ORIENTED_EDGE ( 'NONE', *, *, #26240, .F. ) ;
#8664=CARTESIAN_POINT ( 'NONE',  ( -0.5716039299945605556, -28.49445895580190324, 5.310182064000024127 ) ) ;
#8676=CARTESIAN_POINT ( 'NONE',  ( -25.45015929631789220, 12.82831286024188699, 5.290680260628121800 ) ) ;
#8686=EDGE_LOOP ( 'NONE', ( #19715, #24689, #17839, #9706 ) ) ;
#8692=ORIENTED_EDGE ( 'NONE', *, *, #623, .F. ) ;
#8714=CARTESIAN_POINT ( 'NONE',  ( -28.49528339128749366, -0.5184828350247674411, 1.000000000000000888 ) ) ;
#8715=ORIENTED_EDGE ( 'NONE', *, *, #29248, .F. ) ;
#8719=CARTESIAN_POINT ( 'NONE',  ( 17.93344943624471810, 20.10553870840068313, 0.000000000000000000 ) ) ;
#8726=CARTESIAN_POINT ( 'NONE',  ( 24.88589369718092215, -13.89120818692358483, 3.904029272000009154 ) ) ;
#8729=VECTOR ( 'NONE', #5249, 1000.000000000000000 ) ;
#8732=B_SPLINE_CURVE_WITH_KNOTS ( 'NONE', 5,
 ( #13871, #20636, #11507, #30231, #25682, #15596, #1763, #20950, #6318, #5999, #15912, #13711, #6622, #25521, #23479 ),
 .UNSPECIFIED., .F., .F.,
 ( 6, 3, 3, 3, 6 ),
 ( 0.000000000000000000, 0.5239017171269999551, 1.047803434249999999, 1.571705151379999998, 1.746339057089999924 ),
 .UNSPECIFIED. ) ;
#8733=CYLINDRICAL_SURFACE ( 'NONE', #17768, 1.099999999999999867 ) ;
#8741=CARTESIAN_POINT ( 'NONE',  ( -24.50654363593514873, -14.64341241029205065, 0.02487534799999746582 ) ) ;
#8750=VECTOR ( 'NONE', #25131, 1000.000000000000000 ) ;
#8767=FACE_OUTER_BOUND ( 'NONE', #5835, .T. ) ;
#8787=CARTESIAN_POINT ( 'NONE',  ( 17.93011078765611543, -8.208160914697428368, 0.000000000000000000 ) ) ;
#8791=CARTESIAN_POINT ( 'NONE',  ( 25.35557883893859810, -13.01417686066516488, 5.679894690497184762 ) ) ;
#8798=CARTESIAN_POINT ( 'NONE',  ( 28.49528339128749366, 0.5184828350247745465, 1.000000000000000888 ) ) ;
#8800=CARTESIAN_POINT ( 'NONE',  ( 14.96238942309071085, -23.61101023361229068, 8.000000000000007105 ) ) ;
#8804=CARTESIAN_POINT ( 'NONE',  ( -19.80535357377644701, 19.50875577052588739, 3.000000106999994642 ) ) ;
#8837=CARTESIAN_POINT ( 'NONE',  ( 0.9015611980579174567, -28.48625233387464561, 6.042323509000024906 ) ) ;
#8846=ORIENTED_EDGE ( 'NONE', *, *, #25062, .F. ) ;
#8850=B_SPLINE_CURVE_WITH_KNOTS ( 'NONE', 5,
 ( #47, #28812, #28203, #6645, #25860, #4298, #23503, #1937, #5519, #19545, #24574, #2702, #21746, #5210, #10255 ),
 .UNSPECIFIED., .F., .F.,
 ( 6, 3, 3, 3, 6 ),
 ( 0.000000000000000000, 0.1000000000028630903, 0.3999999999999999667, 0.7000000000005727196, 1.000000000000000000 ),
 .UNSPECIFIED. ) ;
#8851=ORIENTED_EDGE ( 'NONE', *, *, #13098, .T. ) ;
#8852=ORIENTED_EDGE ( 'NONE', *, *, #23068, .F. ) ;
#8877=CARTESIAN_POINT ( 'NONE',  ( 27.24406355354269849, 0.4957164003158900378, 0.08279779300002232389 ) ) ;
#8880=CARTESIAN_POINT ( 'NONE',  ( -23.69427943501400691, -14.54081806258934861, 6.079851352000009257 ) ) ;
#8883=CARTESIAN_POINT ( 'NONE',  ( 24.52721838744982463, -14.51532614974687796, 4.239732040000027347 ) ) ;
#8900=ORIENTED_EDGE ( 'NONE', *, *, #29829, .T. ) ;
#8901=CARTESIAN_POINT ( 'NONE',  ( -27.66290831536099759, -7.787312998881454895, 0.8585786439999909536 ) ) ;
#8902=EDGE_LOOP ( 'NONE', ( #10969, #23510, #21139, #28446, #10907 ) ) ;
#8903=CARTESIAN_POINT ( 'NONE',  ( 19.80526555972147307, 19.50877392102524155, 3.000000000000002665 ) ) ;
#8906=CARTESIAN_POINT ( 'NONE',  ( -15.94126856105729573, 10.34054669365686152, -0.6999999999999783062 ) ) ;
#8908=CARTESIAN_POINT ( 'NONE',  ( -0.6094664100040195764, -28.49364619262437870, 4.895947184000021046 ) ) ;
#8912=PLANE ( 'NONE',  #8965 ) ;
#8921=CARTESIAN_POINT ( 'NONE',  ( 23.74378135472953488, 14.46011237893922008, 3.899998580999998854 ) ) ;
#8936=VERTEX_POINT ( 'NONE', #22752 ) ;
#8959=CARTESIAN_POINT ( 'NONE',  ( -3.397257074621320871, -28.55879647729619109, 8.000000000000007105 ) ) ;
#8962=CARTESIAN_POINT ( 'NONE',  ( 0.5184513693225726305, -28.49550581263314086, 6.099998581000020792 ) ) ;
#8964=CARTESIAN_POINT ( 'NONE',  ( 0.03549436698350039859, -27.80040766163043031, 3.997479608999987555 ) ) ;
#8965=AXIS2_PLACEMENT_3D ( 'NONE', #28116, #13798, #23414 ) ;
#8974=ORIENTED_EDGE ( 'NONE', *, *, #21946, .T. ) ;
#8980=CARTESIAN_POINT ( 'NONE',  ( 24.38199545065365115, 14.75707034588002564, 3.901343066999990228 ) ) ;
#8981=CARTESIAN_POINT ( 'NONE',  ( -16.83342759582943060, -8.999999999996580513, -0.6999999999999784173 ) ) ;
#8982=CARTESIAN_POINT ( 'NONE',  ( -16.06988921231594603, 11.79183908526949054, -0.6999999999999784173 ) ) ;
#8995=CARTESIAN_POINT ( 'NONE',  ( -16.83342759575507586, 10.99999999997565503, -0.6999999999999784173 ) ) ;
#8999=FACE_OUTER_BOUND ( 'NONE', #28176, .T. ) ;
#9009=CARTESIAN_POINT ( 'NONE',  ( -24.18586237362070435, 13.70852494847550673, 3.927704946426889610 ) ) ;
#9017=CARTESIAN_POINT ( 'NONE',  ( 24.37165445055180157, -14.77472140295711434, 5.104215870000011535 ) ) ;
#9033=CARTESIAN_POINT ( 'NONE',  ( -23.35870914495593809, -15.07359600611589912, 4.322692715549829146 ) ) ;
#9038=DIRECTION ( 'NONE',  ( 0.000000000000000000, 0.000000000000000000, -1.000000000000000000 ) ) ;
#9039=B_SPLINE_CURVE_WITH_KNOTS ( 'NONE', 5,
 ( #20190, #5862, #29317, #17660, #8066, #15469, #5710, #3504, #29164 ),
 .UNSPECIFIED., .F., .F.,
 ( 6, 3, 6 ),
 ( 0.000000000000000000, 54.03331039209999886, 92.56095350929999199 ),
 .UNSPECIFIED. ) ;
#9056=CARTESIAN_POINT ( 'NONE',  ( -24.49554752220392118, 11.47491990610730106, 0.000000000000000000 ) ) ;
#9058=CARTESIAN_POINT ( 'NONE',  ( -26.79556473285982321, -0.4875557887251112388, 0.000000000000000000 ) ) ;
#9063=CARTESIAN_POINT ( 'NONE',  ( -1.074123786107241241, 3.361570641823106165, 0.000000000000000000 ) ) ;
#9076=CYLINDRICAL_SURFACE ( 'NONE', #29343, 1.100000000000002309 ) ;
#9091=ORIENTED_EDGE ( 'NONE', *, *, #12521, .T. ) ;
#9093=CARTESIAN_POINT ( 'NONE',  ( 19.80526555962148549, 19.50877392102342256, 1.000000000000000888 ) ) ;
#9108=FACE_OUTER_BOUND ( 'NONE', #7997, .T. ) ;
#9110=CARTESIAN_POINT ( 'NONE',  ( 27.62819777866805637, -4.248501485358312735, 8.000000000000007105 ) ) ;
#9115=CARTESIAN_POINT ( 'NONE',  ( -17.62526668104891314, 11.76353838341477953, 0.000000000000000000 ) ) ;
#9130=( NAMED_UNIT ( * ) SI_UNIT ( $, .STERADIAN. ) SOLID_ANGLE_UNIT ( ) );
#9131=DIRECTION ( 'NONE',  ( 0.6941258031311203780, 0.7198537139083029945, 0.000000000000000000 ) ) ;
#9148=CARTESIAN_POINT ( 'NONE',  ( 24.18731408344101297, -13.70592755508744531, 6.073251382590931335 ) ) ;
#9149=CARTESIAN_POINT ( 'NONE',  ( 1.605176535610508326, -27.75389821387976852, 5.104056378000016103 ) ) ;
#9162=ORIENTED_EDGE ( 'NONE', *, *, #24734, .T. ) ;
#9167=CARTESIAN_POINT ( 'NONE',  ( 28.03861306157277866, 0.5101735396241771081, -0.2432540810000105580 ) ) ;
#9169=EDGE_CURVE ( 'NONE', #24538, #6269, #250, .T. ) ;
#9175=ORIENTED_EDGE ( 'NONE', *, *, #4629, .T. ) ;
#9176=CARTESIAN_POINT ( 'NONE',  ( -18.64452468818404540, 19.99990995005524752, -0.6110695939093615525 ) ) ;
#9183=CARTESIAN_POINT ( 'NONE',  ( 1.592882851206511186, -27.75460863273100998, 4.791883387999989807 ) ) ;
#9197=CARTESIAN_POINT ( 'NONE',  ( 19.73189145681168100, 18.31187121618595270, -0.6999999999999784173 ) ) ;
#9205=CARTESIAN_POINT ( 'NONE',  ( 24.32472724076343695, -13.45989056521276872, 3.899998581000013509 ) ) ;
#9206=CARTESIAN_POINT ( 'NONE',  ( -25.14597776469910428, -15.02549348198344603, 1.000000001000006522 ) ) ;
#9214=ORIENTED_EDGE ( 'NONE', *, *, #19248, .T. ) ;
#9222=CARTESIAN_POINT ( 'NONE',  ( -15.89343021241115039, -9.582866096052068627, 0.000000000000000000 ) ) ;
#9225=FACE_OUTER_BOUND ( 'NONE', #15375, .T. ) ;
#9229=B_SPLINE_CURVE_WITH_KNOTS ( 'NONE', 1,
 ( #11392, #20989 ),
 .UNSPECIFIED., .F., .F.,
 ( 2, 2 ),
 ( -2.555882144480000001E-06, 0.7000000000009999335 ),
 .UNSPECIFIED. ) ;
#9254=EDGE_LOOP ( 'NONE', ( #1686, #28328, #28141, #7595 ) ) ;
#9259=EDGE_CURVE ( 'NONE', #29063, #18612, #6730, .T. ) ;
#9275=EDGE_CURVE ( 'NONE', #25912, #7575, #25872, .T. ) ;
#9279=ORIENTED_EDGE ( 'NONE', *, *, #17819, .F. ) ;
#9288=ORIENTED_EDGE ( 'NONE', *, *, #29785, .F. ) ;
#9291=CARTESIAN_POINT ( 'NONE',  ( 23.98258507289250474, 15.39789216307533160, 4.239862992999999136 ) ) ;
#9294=CARTESIAN_POINT ( 'NONE',  ( 19.67976622696308198, 20.00040984567383617, -0.1488513631577831065 ) ) ;
#9308=B_SPLINE_CURVE_WITH_KNOTS ( 'NONE', 5,
 ( #510, #27227, #8023, #9783, #10248, #21741, #5364, #29273, #29123, #7717, #10094, #21908, #19384, #24416, #29431 ),
 .UNSPECIFIED., .F., .F.,
 ( 6, 3, 3, 3, 6 ),
 ( 0.000000000000000000, 0.1000000000028630903, 0.3999999999999999667, 0.7000000000005727196, 1.000000000000000000 ),
 .UNSPECIFIED. ) ;
#9310=CARTESIAN_POINT ( 'NONE',  ( 0.5401834767575381946, -27.79499634052776358, 6.099998581000020792 ) ) ;
#9316=FACE_OUTER_BOUND ( 'NONE', #12687, .T. ) ;
#9320=ADVANCED_FACE ( 'NONE', ( #30112 ), #17523, .F. ) ;
#9322=ORIENTED_EDGE ( 'NONE', *, *, #15087, .T. ) ;
#9342=CARTESIAN_POINT ( 'NONE',  ( 0.9015611980529183445, -28.48625233387473799, 3.957673652000032405 ) ) ;
#9347=CARTESIAN_POINT ( 'NONE',  ( -16.83342759582943060, -8.999999999996580513, -0.6999999999999784173 ) ) ;
#9350=CARTESIAN_POINT ( 'NONE',  ( -17.52370712817340248, -8.131162915109298339, -0.6999999999999784173 ) ) ;
#9352=CARTESIAN_POINT ( 'NONE',  ( -27.79539923781684863, -0.5057481689248937151, 0.8585786439999909536 ) ) ;
#9361=B_SPLINE_CURVE_WITH_KNOTS ( 'NONE', 5,
 ( #25214, #3645, #24483, #30090, #8516, #18117 ),
 .UNSPECIFIED., .F., .F.,
 ( 6, 6 ),
 ( 0.000000000000000000, 24.02090357630000028 ),
 .UNSPECIFIED. ) ;
#9371=CARTESIAN_POINT ( 'NONE',  ( 23.55411374389464285, 16.04538543789061933, 8.000000000000007105 ) ) ;
#9387=CARTESIAN_POINT ( 'NONE',  ( -16.25056150175689496, -8.060002615884259924, 0.000000000000000000 ) ) ;
#9395=EDGE_CURVE ( 'NONE', #19325, #7575, #10085, .T. ) ;
#9416=CARTESIAN_POINT ( 'NONE',  ( 24.50348397774029152, -13.13223627703424690, 6.042507865999996675 ) ) ;
#9424=CARTESIAN_POINT ( 'NONE',  ( -24.45473033751197178, -14.63622298155413226, 6.098654221000004760 ) ) ;
#9440=ORIENTED_EDGE ( 'NONE', *, *, #11935, .T. ) ;
#9442=EDGE_CURVE ( 'NONE', #1647, #8375, #21677, .T. ) ;
#9450=CARTESIAN_POINT ( 'NONE',  ( 17.14656078602323319, -7.900182044548062166, -1.000005633855494125E-09 ) ) ;
#9457=CARTESIAN_POINT ( 'NONE',  ( -0.01829671460840276778, -3.547951512854698564, 0.000000000000000000 ) ) ;
#9462=CARTESIAN_POINT ( 'NONE',  ( -17.13980697764020178, 12.06576768890603013, -0.6999999999999785283 ) ) ;
#9495=CARTESIAN_POINT ( 'NONE',  ( -20.05890038391583730, 19.99998511269691193, 0.2505997993269546975 ) ) ;
#9497=B_SPLINE_SURFACE_WITH_KNOTS ( 'NONE', 5, 1, ( 
 ( #23783, #16376 ),
 ( #18731, #21420 ),
 ( #4271, #4109 ),
 ( #21258, #2067 ),
 ( #11658, #20947 ),
 ( #19048, #30857 ),
 ( #9291, #28490 ),
 ( #20790, #31010 ),
 ( #13868, #6781 ),
 ( #23475, #6930 ),
 ( #16529, #30551 ),
 ( #25678, #26140 ),
 ( #8980, #4573 ),
 ( #23313, #14178 ),
 ( #1909, #28646 ) ),
 .UNSPECIFIED., .F., .F., .F.,
 ( 6, 3, 3, 3, 6 ),
 ( 2, 2 ),
 ( 0.000000000000000000, 0.5238999882350000581, 1.047799976470000116, 1.571699964700000063, 1.746333294120000046 ),
 ( -0.7000000000009999335, 2.555897717360000054E-06 ),
 .UNSPECIFIED. ) ;
#9502=EDGE_LOOP ( 'NONE', ( #12697, #13548, #2550, #16189 ) ) ;
#9518=CARTESIAN_POINT ( 'NONE',  ( -26.87967798701711786, 4.135222155429991275, 0.000000000000000000 ) ) ;
#9522=FILL_AREA_STYLE ('',( #19429 ) ) ;
#9525=CARTESIAN_POINT ( 'NONE',  ( 23.78314118259453380, 14.39461387841678608, 6.098654095000016540 ) ) ;
#9545=CARTESIAN_POINT ( 'NONE',  ( 19.80526555972147307, 19.50877392102524155, 3.000000000000002665 ) ) ;
#9549=CARTESIAN_POINT ( 'NONE',  ( -24.97129468253034545, 13.73710443232325495, 3.901342130000013064 ) ) ;
#9566=ORIENTED_EDGE ( 'NONE', *, *, #11639, .F. ) ;
#9570=CARTESIAN_POINT ( 'NONE',  ( -17.62526623054365871, -8.236462051082252600, 0.000000000000000000 ) ) ;
#9573=CARTESIAN_POINT ( 'NONE',  ( 27.79539923781684507, 0.5057481689249165857, 1.000000000000000888 ) ) ;
#9585=CARTESIAN_POINT ( 'NONE',  ( -20.25360395112956269, 20.00000005254026192, 0.6180758210000136810 ) ) ;
#9587=DIRECTION ( 'NONE',  ( 0.000000000000000000, 0.000000000000000000, -1.000000000000000000 ) ) ;
#9592=CARTESIAN_POINT ( 'NONE',  ( -17.66983789954736750, -8.284439791107988782, 0.000000000000000000 ) ) ;
#9596=CARTESIAN_POINT ( 'NONE',  ( 24.97129468909112404, -13.73710443560444183, 3.901342130000013064 ) ) ;
#9609=CARTESIAN_POINT ( 'NONE',  ( 18.39548692765703208, 20.00005474883426970, -0.6591334621046254227 ) ) ;
#9610=CARTESIAN_POINT ( 'NONE',  ( -24.52721838146529620, 14.51532614515499020, 5.760265123000013254 ) ) ;
#9616=CARTESIAN_POINT ( 'NONE',  ( 3.221827467136498591, 1.415571281914143720, 0.000000000000000000 ) ) ;
#9619=CARTESIAN_POINT ( 'NONE',  ( 24.47278418934494937, 14.60601539438439822, 6.095965388000001539 ) ) ;
#9623=CARTESIAN_POINT ( 'NONE',  ( -24.45473033751197178, -14.63622298155413226, 3.901342939999996595 ) ) ;
#9628=CARTESIAN_POINT ( 'NONE',  ( 17.00259495291042455, 12.09719844080319895, -4.336808689942018722E-16 ) ) ;
#9629=B_SPLINE_CURVE_WITH_KNOTS ( 'NONE', 5,
 ( #29920, #27704, #18103, #27554, #12930, #22227, #25199, #1291, #986, #14992, #24589, #5998, #27250, #15593, #681 ),
 .UNSPECIFIED., .F., .F.,
 ( 6, 3, 3, 3, 6 ),
 ( 0.000000000000000000, 0.1000000000034356601, 0.4000000000022904678, 0.7000000000005727196, 1.000000000000000000 ),
 .UNSPECIFIED. ) ;
#9650=CARTESIAN_POINT ( 'NONE',  ( -17.91543966611209981, 20.00000000001002221, -0.6999999999999785283 ) ) ;
#9654=ORIENTED_EDGE ( 'NONE', *, *, #25278, .T. ) ;
#9655=CARTESIAN_POINT ( 'NONE',  ( 16.10061776519356869, 10.69263420686418442, -0.6999999999999784173 ) ) ;
#9657=CARTESIAN_POINT ( 'NONE',  ( 28.41645191122389846, 4.850979895915015661, 1.000000000000000888 ) ) ;
#9667=CARTESIAN_POINT ( 'NONE',  ( -27.88265104574380260, 4.289521473631270787, 1.000000000000000888 ) ) ;
#9669=ORIENTED_EDGE ( 'NONE', *, *, #23334, .T. ) ;
#9678=CARTESIAN_POINT ( 'NONE',  ( 0.5184513693225726305, -28.49550581263314086, 6.099998581000020792 ) ) ;
#9680=EDGE_CURVE ( 'NONE', #170, #12548, #26968, .T. ) ;
#9689=ORIENTED_EDGE ( 'NONE', *, *, #14130, .F. ) ;
#9693=CARTESIAN_POINT ( 'NONE',  ( -15.73383125209597999, -9.054522205455617367, 0.000000000000000000 ) ) ;
#9704=CARTESIAN_POINT ( 'NONE',  ( 24.41841038956698640, 14.69667349781389376, 6.099998581000020792 ) ) ;
#9706=ORIENTED_EDGE ( 'NONE', *, *, #17557, .T. ) ;
#9733=CARTESIAN_POINT ( 'NONE',  ( -17.83930458829795640, 19.99999999999961631, 0.000000000000000000 ) ) ;
#9740=EDGE_CURVE ( 'NONE', #4471, #6349, #19442, .T. ) ;
#9748=CARTESIAN_POINT ( 'NONE',  ( 24.83827472153076599, -12.48687851163286133, 4.999998581000003384 ) ) ;
#9753=B_SPLINE_SURFACE_WITH_KNOTS ( 'NONE', 5, 1, ( 
 ( #6550, #13952 ),
 ( #8908, #23565 ),
 ( #27956, #2000 ),
 ( #28580, #7020 ),
 ( #1532, #11590 ),
 ( #6396, #18509 ),
 ( #4192, #28420 ),
 ( #25762, #21038 ),
 ( #16147, #30639 ),
 ( #4039, #3883 ),
 ( #15996, #21186 ),
 ( #28111, #4511 ),
 ( #13474, #30486 ),
 ( #13637, #13794 ),
 ( #1839, #1683 ) ),
 .UNSPECIFIED., .F., .F., .F.,
 ( 6, 3, 3, 3, 6 ),
 ( 2, 2 ),
 ( 0.000000000000000000, 0.5239017171269999551, 1.047803434249999999, 1.571705151379999998, 1.746339057089999924 ),
 ( -0.7000000000009999335, 2.556331299420000144E-06 ),
 .UNSPECIFIED. ) ;
#9756=ORIENTED_EDGE ( 'NONE', *, *, #19824, .T. ) ;
#9757=CARTESIAN_POINT ( 'NONE',  ( -27.79539923781770483, -0.5057481688778011630, 1.000000000000000888 ) ) ;
#9762=CARTESIAN_POINT ( 'NONE',  ( 20.22062173471788071, 19.99992278450133298, 0.4812210343388954037 ) ) ;
#9763=CARTESIAN_POINT ( 'NONE',  ( -23.88992818679365371, 14.21747995069046588, 5.680829343999993952 ) ) ;
#9776=CARTESIAN_POINT ( 'NONE',  ( -16.85343921394901301, 12.09981795542885585, -0.6999999989999727834 ) ) ;
#9777=B_SPLINE_CURVE_WITH_KNOTS ( 'NONE', 3,
 ( #27400, #5685, #19870, #15442, #10572, #17788 ),
 .UNSPECIFIED., .F., .F.,
 ( 4, 2, 4 ),
 ( 0.000000000000000000, 0.5000000000000000000, 1.000000000000000000 ),
 .UNSPECIFIED. ) ;
#9778=CARTESIAN_POINT ( 'NONE',  ( 20.30396079673062815, 19.99999999994985700, 0.8743359189999910797 ) ) ;
#9779=CARTESIAN_POINT ( 'NONE',  ( -25.46368746804859740, 12.80129684245613575, 4.999998581000003384 ) ) ;
#9783=CARTESIAN_POINT ( 'NONE',  ( 0.6090474298383116158, -27.79358669172298946, 6.095948809000023338 ) ) ;
#9787=( GEOMETRIC_REPRESENTATION_CONTEXT ( 3 ) GLOBAL_UNCERTAINTY_ASSIGNED_CONTEXT ( ( #16610 ) ) GLOBAL_UNIT_ASSIGNED_CONTEXT ( ( #5103, #24153, #14872 ) ) REPRESENTATION_CONTEXT ( 'NONE', 'WORKASPACE' ) );
#9789=CARTESIAN_POINT ( 'NONE',  ( 16.47468026047738121, 11.86718987800275471, -4.336808689942017736E-16 ) ) ;
#9793=CARTESIAN_POINT ( 'NONE',  ( 24.21906834310036771, 15.02342240524378703, 3.957526369000014199 ) ) ;
#9797=VERTEX_POINT ( 'NONE', #11186 ) ;
#9802=CARTESIAN_POINT ( 'NONE',  ( 18.03376228215428156, -8.308107856198580166, -4.336808689942017736E-16 ) ) ;
#9804=CARTESIAN_POINT ( 'NONE',  ( -25.44662322720214576, 12.83524168061546966, 5.310645680000003921 ) ) ;
#9811=CARTESIAN_POINT ( 'NONE',  ( -17.83929479963776288, 19.99998902616253105, -0.6999999999999784173 ) ) ;
#9820=CARTESIAN_POINT ( 'NONE',  ( 3.040504021322313122, 1.733590290792417887, -0.6999999999999784173 ) ) ;
#9832=( NAMED_UNIT ( * ) PLANE_ANGLE_UNIT ( ) SI_UNIT ( $, .RADIAN. ) );
#9847=ORIENTED_EDGE ( 'NONE', *, *, #2240, .F. ) ;
#9849=CARTESIAN_POINT ( 'NONE',  ( -24.36724936496760918, -13.38201651699120021, 5.104178996000019453 ) ) ;
#9850=CARTESIAN_POINT ( 'NONE',  ( -23.39354070939840824, -15.01969650306709170, 5.760134161999996394 ) ) ;
#9856=CARTESIAN_POINT ( 'NONE',  ( -19.89993772616713841, -20.76973888581983019, -0.6577119969999878357 ) ) ;
#9858=CARTESIAN_POINT ( 'NONE',  ( 28.68577476838161644, -9.950727360109466346, 8.000000000000007105 ) ) ;
#9865=EDGE_CURVE ( 'NONE', #16870, #28488, #5555, .T. ) ;
#9876=ORIENTED_EDGE ( 'NONE', *, *, #10187, .T. ) ;
#9878=CARTESIAN_POINT ( 'NONE',  ( -23.79228473957821777, 14.38012949749760416, 4.689353541000001790 ) ) ;
#9879=CARTESIAN_POINT ( 'NONE',  ( -27.87609112763809449, 3.928995115440388375, 5.200000000000009948 ) ) ;
#9880=B_SPLINE_SURFACE_WITH_KNOTS ( 'NONE', 5, 1, ( 
 ( #11594, #4357 ),
 ( #7337, #26529 ),
 ( #6860, #6707 ),
 ( #26385, #19139 ),
 ( #2314, #14581 ),
 ( #9371, #2156 ) ),
 .UNSPECIFIED., .F., .F., .F.,
 ( 6, 6 ),
 ( 2, 2 ),
 ( 0.000000000000000000, 7.118175366610000054 ),
 ( -0.7000000000080000007, 0.0003774914509440000041 ),
 .UNSPECIFIED. ) ;
#9907=CARTESIAN_POINT ( 'NONE',  ( 24.37450210455010335, -13.36961646745188759, 3.904029301000005781 ) ) ;
#9918=CARTESIAN_POINT ( 'NONE',  ( -27.66290831536099759, -7.787312998881454895, 1.000000000000000888 ) ) ;
#9922=B_SPLINE_CURVE_WITH_KNOTS ( 'NONE', 5,
 ( #21050, #8600, #3896, #16318, #25929, #22941, #4206, #30168, #6255 ),
 .UNSPECIFIED., .F., .F.,
 ( 6, 3, 6 ),
 ( 0.000000000000000000, 53.20205529499999386, 91.13698440880000362 ),
 .UNSPECIFIED. ) ;
#9924=CARTESIAN_POINT ( 'NONE',  ( -24.93720648713954446, 13.79881813474513486, 6.099998581000020792 ) ) ;
#9926=CARTESIAN_POINT ( 'NONE',  ( -17.83929479963776288, 19.99998902616253105, -0.6999999999999784173 ) ) ;
#9929=CARTESIAN_POINT ( 'NONE',  ( -3.040504021322313122, -1.733590290792417887, 0.000000000000000000 ) ) ;
#9931=CARTESIAN_POINT ( 'NONE',  ( 24.49145441566124148, -14.57548795709913847, 5.680829342999987652 ) ) ;
#9938=CARTESIAN_POINT ( 'NONE',  ( -24.61381496313306982, -14.36755986783020056, 3.957524336000023624 ) ) ;
#9944=LINE ( 'NONE', #17777, #17335 ) ;
#9945=LINE ( 'NONE', #24885, #24281 ) ;
#9949=B_SPLINE_SURFACE_WITH_KNOTS ( 'NONE', 5, 1, ( 
 ( #17239, #27454 ),
 ( #20079, #24489 ),
 ( #2928, #5896 ),
 ( #29669, #25107 ),
 ( #4336, #25432 ),
 ( #6214, #18167 ),
 ( #8883, #27936 ),
 ( #18488, #15974 ),
 ( #20697, #1349 ),
 ( #15653, #10786 ),
 ( #27770, #20384 ),
 ( #8726, #30135 ),
 ( #15823, #13615 ),
 ( #8566, #28086 ),
 ( #23220, #22744 ) ),
 .UNSPECIFIED., .F., .F., .F.,
 ( 6, 3, 3, 3, 6 ),
 ( 2, 2 ),
 ( 0.000000000000000000, 0.5239055193860000514, 1.047811038770000147, 1.571716558150000109, 1.746351731290000098 ),
 ( -0.7000000000009999335, 2.557300549769999790E-06 ),
 .UNSPECIFIED. ) ;
#9959=ORIENTED_EDGE ( 'NONE', *, *, #1666, .F. ) ;
#9984=AXIS2_PLACEMENT_3D ( 'NONE', #19017, #28620, #29075 ) ;
#9986=ADVANCED_FACE ( 'NONE', ( #30147 ), #12422, .F. ) ;
#9989=ORIENTED_EDGE ( 'NONE', *, *, #23655, .T. ) ;
#10010=B_SPLINE_CURVE_WITH_KNOTS ( 'NONE', 1,
 ( #30327, #5195 ),
 .UNSPECIFIED., .F., .F.,
 ( 2, 2 ),
 ( -2.393070191420000080E-05, 0.7036780443879999680 ),
 .UNSPECIFIED. ) ;
#10014=CARTESIAN_POINT ( 'NONE',  ( -27.55801272791059731, -0.5014288284350322256, -0.5592437529999827461 ) ) ;
#10038=CARTESIAN_POINT ( 'NONE',  ( -24.49145440958036701, 14.57548795270903774, 4.319167817000008291 ) ) ;
#10053=CARTESIAN_POINT ( 'NONE',  ( -23.77307140041805411, 14.41181874028064591, 4.999998581000003384 ) ) ;
#10054=CARTESIAN_POINT ( 'NONE',  ( -15.76765990766156733, 11.30637938232363204, -0.6999999999999785283 ) ) ;
#10057=CARTESIAN_POINT ( 'NONE',  ( -15.96623771770940969, 11.69189214367815843, -4.336808689942017736E-16 ) ) ;
#10085=B_SPLINE_CURVE_WITH_KNOTS ( 'NONE', 5,
 ( #3051, #10603, #8379, #27281, #6030, #5413, #17976, #20198, #5721, #24927, #29791, #27589, #17825, #13108, #25079 ),
 .UNSPECIFIED., .F., .F.,
 ( 6, 3, 3, 3, 6 ),
 ( 0.000000000000000000, 0.3000000000011452950, 0.6000000000034357850, 0.9000000000022905233, 1.000000000000000000 ),
 .UNSPECIFIED. ) ;
#10089=CARTESIAN_POINT ( 'NONE',  ( 24.09407739349263622, -13.86899051603569255, 6.002806299999996043 ) ) ;
#10092=CARTESIAN_POINT ( 'NONE',  ( -24.37165444408190851, 14.77472139917419369, 4.999998581000003384 ) ) ;
#10094=CARTESIAN_POINT ( 'NONE',  ( 1.495522319900055574, -27.76012052182101542, 5.506490228000010312 ) ) ;
#10098=CARTESIAN_POINT ( 'NONE',  ( 18.26639035967037827, -8.979988381807324060, -0.6999999999999784173 ) ) ;
#10114=CARTESIAN_POINT ( 'NONE',  ( 16.40303402075260308, 10.20816091466531716, -0.6999999999999784173 ) ) ;
#10116=CARTESIAN_POINT ( 'NONE',  ( -25.16696685493285202, 13.37570800105521585, 6.002806401000010617 ) ) ;
#10117=CARTESIAN_POINT ( 'NONE',  ( -14.60916135985672071, 28.04296594682689658, 8.000000000000007105 ) ) ;
#10128=CARTESIAN_POINT ( 'NONE',  ( 0.5746121234323043891, -27.79431838510023667, 3.901346086000012647 ) ) ;
#10129=CARTESIAN_POINT ( 'NONE',  ( -24.82552935800767457, 12.51236512602968887, 4.712680001979744127 ) ) ;
#10136=CARTESIAN_POINT ( 'NONE',  ( -28.49528339128749366, -0.5184828350247674411, 1.000000000000000888 ) ) ;
#10137=CARTESIAN_POINT ( 'NONE',  ( -24.18086174036168856, 13.20182724809068553, 0.000000000000000000 ) ) ;
#10145=CARTESIAN_POINT ( 'NONE',  ( 24.12437077020566534, 15.17512415148409133, 5.965434402546257786 ) ) ;
#10152=CARTESIAN_POINT ( 'NONE',  ( -28.58473218748631339, 4.397531023511127124, 1.000000000000000888 ) ) ;
#10162=CARTESIAN_POINT ( 'NONE',  ( -23.29312071521372118, -15.17488101142239643, 5.506989586000016423 ) ) ;
#10171=EDGE_CURVE ( 'NONE', #16061, #7420, #19051, .T. ) ;
#10174=CARTESIAN_POINT ( 'NONE',  ( -0.5944614571882205212, -27.79380703160649446, 4.999998581000003384 ) ) ;
#10180=B_SPLINE_CURVE_WITH_KNOTS ( 'NONE', 5,
 ( #279, #9858, #19456, #26688, #29049, #7494, #14738, #12370, #23726 ),
 .UNSPECIFIED., .F., .F.,
 ( 6, 3, 6 ),
 ( 0.000000000000000000, 55.31395627320000585, 94.75474476520000167 ),
 .UNSPECIFIED. ) ;
#10182=ORIENTED_EDGE ( 'NONE', *, *, #5246, .F. ) ;
#10187=EDGE_CURVE ( 'NONE', #14604, #22866, #8560, .T. ) ;
#10189=CARTESIAN_POINT ( 'NONE',  ( -24.92013865347427171, 13.82966157970119525, 3.899998581000013509 ) ) ;
#10190=CARTESIAN_POINT ( 'NONE',  ( -28.49530731802708416, -0.5184832703812605192, 8.000000000000007105 ) ) ;
#10203=CARTESIAN_POINT ( 'NONE',  ( -16.14153545196241524, 10.13281012202415177, -4.336808689942017736E-16 ) ) ;
#10217=CARTESIAN_POINT ( 'NONE',  ( 25.32653163311281830, -13.07087917458821202, 4.239730452999995514 ) ) ;
#10241=CARTESIAN_POINT ( 'NONE',  ( 23.88992819277635959, -14.21747995518237317, 5.680829342999987652 ) ) ;
#10242=CARTESIAN_POINT ( 'NONE',  ( 23.85408961476034051, 14.27673465474052072, 6.098654221000004760 ) ) ;
#10248=CARTESIAN_POINT ( 'NONE',  ( 0.7459188900473354700, -27.79046661982714639, 6.079790450999988494 ) ) ;
#10249=CARTESIAN_POINT ( 'NONE',  ( -24.36130770023227043, -13.39283555866521525, 4.791638085000021974 ) ) ;
#10253=B_SPLINE_CURVE_WITH_KNOTS ( 'NONE', 3,
 ( #29612, #5536, #24591, #17640, #24742, #5844, #20323, #29921, #15446, #10424, #5690, #22685 ),
 .UNSPECIFIED., .F., .F.,
 ( 4, 2, 2, 2, 2, 4 ),
 ( 0.000000000000000000, 0.2500000000000002776, 0.5000000000000005551, 0.6250000000000001110, 0.7499999999999996669, 1.000000000000000000 ),
 .UNSPECIFIED. ) ;
#10255=CARTESIAN_POINT ( 'NONE',  ( 1.645560275461343203, -28.45273235261698019, 4.999998581000003384 ) ) ;
#10259=DIRECTION ( 'NONE',  ( 0.000000000000000000, 0.000000000000000000, -1.000000000000000000 ) ) ;
#10271=CARTESIAN_POINT ( 'NONE',  ( -24.98823330661245379, 13.70626928206978690, 6.095967861000000987 ) ) ;
#10306=ORIENTED_EDGE ( 'NONE', *, *, #17676, .F. ) ;
#10309=CARTESIAN_POINT ( 'NONE',  ( -27.57306739230703130, 9.318986405453829391, 0.5017677510000262409 ) ) ;
#10322=CARTESIAN_POINT ( 'NONE',  ( -24.38199545545641911, -14.75707035126829147, 6.098654095000016540 ) ) ;
#10327=CARTESIAN_POINT ( 'NONE',  ( -28.45300238704230367, -0.5177135156027806717, 0.5017677510000262409 ) ) ;
#10343=ORIENTED_EDGE ( 'NONE', *, *, #6615, .T. ) ;
#10367=EDGE_CURVE ( 'NONE', #18124, #17421, #14881, .T. ) ;
#10370=B_SPLINE_CURVE_WITH_KNOTS ( 'NONE', 1,
 ( #21239, #4708 ),
 .UNSPECIFIED., .F., .F.,
 ( 2, 2 ),
 ( -2.557300549769999790E-06, 0.7000000000009999335 ),
 .UNSPECIFIED. ) ;
#10382=CARTESIAN_POINT ( 'NONE',  ( -17.59696597919420213, 10.20816091468181774, -0.6999999999999784173 ) ) ;
#10396=CARTESIAN_POINT ( 'NONE',  ( 24.06826093661917554, -20.50742065831276051, 8.000000000000007105 ) ) ;
#10412=CARTESIAN_POINT ( 'NONE',  ( 23.81866167241657806, 14.33570040768432996, 3.899998581000013509 ) ) ;
#10413=ORIENTED_EDGE ( 'NONE', *, *, #30113, .F. ) ;
#10422=DIRECTION ( 'NONE',  ( 0.000000000000000000, 0.000000000000000000, -1.000000000000000000 ) ) ;
#10424=CARTESIAN_POINT ( 'NONE',  ( -24.35329726287045915, -13.40752173053085983, 5.289304314274809293 ) ) ;
#10437=EDGE_CURVE ( 'NONE', #5736, #15510, #9229, .T. ) ;
#10438=CARTESIAN_POINT ( 'NONE',  ( -1.335589246056437140, 3.267430459342669735, -0.6999999999999783062 ) ) ;
#10445=CARTESIAN_POINT ( 'NONE',  ( -22.97593529893700648, 15.65128280014837081, 8.000000000000007105 ) ) ;
#10453=CARTESIAN_POINT ( 'NONE',  ( -24.93720648713954446, 13.79881813474513486, 3.899998581000013509 ) ) ;
#10460=CARTESIAN_POINT ( 'NONE',  ( -24.50110440319828342, 13.37667737394870748, -0.6577119969999878357 ) ) ;
#10475=CARTESIAN_POINT ( 'NONE',  ( -24.40022624598054435, -14.72688605908970239, 6.099998581000020792 ) ) ;
#10476=CARTESIAN_POINT ( 'NONE',  ( -24.36725163762957536, -13.38201776503690432, 4.926540930971143872 ) ) ;
#10480=CARTESIAN_POINT ( 'NONE',  ( -26.66783967069105898, -7.507193849635574345, -0.6999999999999784173 ) ) ;
#10508=CARTESIAN_POINT ( 'NONE',  ( 24.96253706050071131, 13.75225324050492581, 4.689458287000014991 ) ) ;
#10529=VERTEX_POINT ( 'NONE', #4924 ) ;
#10535=CARTESIAN_POINT ( 'NONE',  ( 24.92639507930385889, 13.81781707913292934, 4.493023686000019445 ) ) ;
#10536=CARTESIAN_POINT ( 'NONE',  ( -0.5944614084144663746, -27.79380475670850359, 5.146930914275719360 ) ) ;
#10551=CARTESIAN_POINT ( 'NONE',  ( 17.83931306984926835, 20.00000000000176570, 0.000000000000000000 ) ) ;
#10553=CARTESIAN_POINT ( 'NONE',  ( 27.79539923781684507, 0.5057481689249130330, 1.000000000000000888 ) ) ;
#10555=FACE_OUTER_BOUND ( 'NONE', #30425, .T. ) ;
#10558=ORIENTED_EDGE ( 'NONE', *, *, #6513, .F. ) ;
#10571=CARTESIAN_POINT ( 'NONE',  ( 16.62864107308872264, -9.970561443424061920, -0.000000000000000000 ) ) ;
#10572=CARTESIAN_POINT ( 'NONE',  ( -17.93062603662948717, -9.163977451850843892, -0.6999999999999784173 ) ) ;
#10574=FILL_AREA_STYLE ('',( #984 ) ) ;
#10576=CARTESIAN_POINT ( 'NONE',  ( 0.1352650258152492124, -28.50015511220863118, 6.042326290000010758 ) ) ;
#10580=ADVANCED_FACE ( 'NONE', ( #26637 ), #20984, .T. ) ;
#10592=VERTEX_POINT ( 'NONE', #12616 ) ;
#10596=CARTESIAN_POINT ( 'NONE',  ( -27.79539923781770128, -0.5057481688779147389, 8.000000000000007105 ) ) ;
#10597=EDGE_CURVE ( 'NONE', #11027, #26158, #8345, .T. ) ;
#10603=CARTESIAN_POINT ( 'NONE',  ( -24.37165444408190851, 14.77472139917419369, 4.895781291000017355 ) ) ;
#10606=EDGE_CURVE ( 'NONE', #3709, #6569, #9629, .T. ) ;
#10609=CARTESIAN_POINT ( 'NONE',  ( -25.54177752991350303, 13.94484553950296934, 0.5017677510000262409 ) ) ;
#10615=CARTESIAN_POINT ( 'NONE',  ( 24.39135169767337885, -14.74223403355047068, 4.689353541000001790 ) ) ;
#10616=EDGE_CURVE ( 'NONE', #23233, #14792, #5689, .T. ) ;
#10618=ORIENTED_EDGE ( 'NONE', *, *, #1632, .T. ) ;
#10622=CARTESIAN_POINT ( 'NONE',  ( 17.83931306984926835, 20.00000000000176570, 0.000000000000000000 ) ) ;
#10623=CARTESIAN_POINT ( 'NONE',  ( 16.06941601916650342, -9.166288768300725920, 0.000000000000000000 ) ) ;
#10644=CARTESIAN_POINT ( 'NONE',  ( -4.575152268165027181, -30.31846920187740224, 0.08279701300001329756 ) ) ;
#10647=CARTESIAN_POINT ( 'NONE',  ( 25.35851007746311581, -13.00862288856444238, 4.319165765000021473 ) ) ;
#10648=CARTESIAN_POINT ( 'NONE',  ( -19.80535357367646654, 19.50875577052770993, 1.000000000000000888 ) ) ;
#10650=FACE_OUTER_BOUND ( 'NONE', #13584, .T. ) ;
#10651=CARTESIAN_POINT ( 'NONE',  ( 25.32653163311281830, -13.07087917458821202, 5.760266709000011254 ) ) ;
#10655=CARTESIAN_POINT ( 'NONE',  ( 22.97559295455008765, 15.65128684778802715, 8.000000000000007105 ) ) ;
#10680=CARTESIAN_POINT ( 'NONE',  ( 24.41841038956698640, 14.69667349781389376, 3.899998581000013509 ) ) ;
#10683=CARTESIAN_POINT ( 'NONE',  ( -27.71261514784184499, -0.5042418799608719970, 0.5514269430000329208 ) ) ;
#10701=CARTESIAN_POINT ( 'NONE',  ( 22.62517538422034136, 16.36045799713766158, 1.000000000000000888 ) ) ;
#10720=CARTESIAN_POINT ( 'NONE',  ( -24.97129468253034545, 13.73710443232325495, 6.098655031999994591 ) ) ;
#10721=CARTESIAN_POINT ( 'NONE',  ( 25.77914806503467560, 15.40383291000323318, 8.000000000000007105 ) ) ;
#10741=CARTESIAN_POINT ( 'NONE',  ( -24.34246741826368066, -14.82285105945933346, 6.099998581000011022 ) ) ;
#10750=AXIS2_PLACEMENT_3D ( 'NONE', #7345, #12211, #21510 ) ;
#10752=VERTEX_POINT ( 'NONE', #8982 ) ;
#10758=LINE ( 'NONE', #19745, #28576 ) ;
#10761=CARTESIAN_POINT ( 'NONE',  ( -22.51305616955001909, 17.92067914158993247, 0.2374258030000131470 ) ) ;
#10765=CARTESIAN_POINT ( 'NONE',  ( -25.32653162617393861, 13.07087917251410403, 4.239730451999990102 ) ) ;
#10779=CARTESIAN_POINT ( 'NONE',  ( 26.68292649568609320, 9.659560297578410726, 0.8585786470000078552 ) ) ;
#10786=CARTESIAN_POINT ( 'NONE',  ( 24.14205449336675713, -13.78537897189897343, 3.957489350000009676 ) ) ;
#10788=B_SPLINE_CURVE_WITH_KNOTS ( 'NONE', 5,
 ( #13289, #29966, #29502, #8395, #7939, #18158 ),
 .UNSPECIFIED., .F., .F.,
 ( 6, 6 ),
 ( 0.000000000000000000, 1.000000000000000000 ),
 .UNSPECIFIED. ) ;
#10789=CARTESIAN_POINT ( 'NONE',  ( 0.1319790757060198549, -27.80015609199462290, 6.042326290000010758 ) ) ;
#10798=VECTOR ( 'NONE', #1854, 1000.000000000000000 ) ;
#10809=CARTESIAN_POINT ( 'NONE',  ( -3.547887315624706162, 0.01749626818370194140, 0.000000000000000000 ) ) ;
#10811=CARTESIAN_POINT ( 'NONE',  ( -28.53958170586710352, 1.916106982190598051, 8.000000000000007105 ) ) ;
#10813=CARTESIAN_POINT ( 'NONE',  ( 24.73568148353697183, -12.68911065183860920, 5.680831396999986183 ) ) ;
#10839=ORIENTED_EDGE ( 'NONE', *, *, #19399, .T. ) ;
#10846=CARTESIAN_POINT ( 'NONE',  ( -17.66508489110463032, -9.721079119778234912, 0.000000000000000000 ) ) ;
#10868=CARTESIAN_POINT ( 'NONE',  ( 18.97091132401531510, 21.26865671844599248, 0.7595836940000044724 ) ) ;
#10872=CARTESIAN_POINT ( 'NONE',  ( 23.78314118259453380, 14.39461387841678608, 6.098654095000016540 ) ) ;
#10874=ORIENTED_EDGE ( 'NONE', *, *, #12521, .F. ) ;
#10887=CARTESIAN_POINT ( 'NONE',  ( 17.14656078602323319, -7.900182044548062166, -1.000005633855494125E-09 ) ) ;
#10890=CARTESIAN_POINT ( 'NONE',  ( 23.77307027438179077, -14.41181805763359947, 4.926507320169768889 ) ) ;
#10891=B_SPLINE_CURVE_WITH_KNOTS ( 'NONE', 5,
 ( #30737, #21454, #23974, #7434, #9167, #31048, #6818, #4776, #12003 ),
 .UNSPECIFIED., .F., .F.,
 ( 6, 3, 6 ),
 ( 8.011061266649999624, 9.405960541640000727, 10.80085981660000094 ),
 .UNSPECIFIED. ) ;
#10906=CARTESIAN_POINT ( 'NONE',  ( -23.88383647328724280, -15.55037090958975909, 5.498277346593025250 ) ) ;
#10907=ORIENTED_EDGE ( 'NONE', *, *, #18448, .T. ) ;
#10915=ORIENTED_EDGE ( 'NONE', *, *, #5042, .F. ) ;
#10922=CARTESIAN_POINT ( 'NONE',  ( 1.645560275461343203, -28.45273235261698019, 4.999998581000003384 ) ) ;
#10927=CYLINDRICAL_SURFACE ( 'NONE', #539, 1.099999999999999867 ) ;
#10936=CARTESIAN_POINT ( 'NONE',  ( 27.68716793528856712, 5.086682278514146560, 0.7069222069999991920 ) ) ;
#10949=CARTESIAN_POINT ( 'NONE',  ( 26.76132339671151072, 2.369424447203797524, -0.6999999999999784173 ) ) ;
#10959=CARTESIAN_POINT ( 'NONE',  ( 13.73773747404255552, -26.37022765825810922, 0.000000000000000000 ) ) ;
#10964=CARTESIAN_POINT ( 'NONE',  ( 2.858922298043036214, 2.052062286655957024, 0.000000000000000000 ) ) ;
#10967=CARTESIAN_POINT ( 'NONE',  ( -16.60814955199252552, -10.08408157955485684, 0.000000000000000000 ) ) ;
#10969=ORIENTED_EDGE ( 'NONE', *, *, #12310, .T. ) ;
#10970=FACE_BOUND ( 'NONE', #9254, .T. ) ;
#10979=CARTESIAN_POINT ( 'NONE',  ( 23.52813227406869245, 14.80830602532641294, 4.039148185435011307 ) ) ;
#10980=CARTESIAN_POINT ( 'NONE',  ( -15.88307796629033852, -8.427117116629231575, -0.6999999999999784173 ) ) ;
#11016=CARTESIAN_POINT ( 'NONE',  ( 12.88923445963852288, -24.80392650440079905, 8.000000000000007105 ) ) ;
#11020=DIRECTION ( 'NONE',  ( 0.000000000000000000, 0.000000000000000000, -1.000000000000000000 ) ) ;
#11024=CARTESIAN_POINT ( 'NONE',  ( 23.29312071241426096, 15.17488100587054767, 5.506989593000027661 ) ) ;
#11025=CARTESIAN_POINT ( 'NONE',  ( 17.95841148948556310, 10.23646161652002817, 0.000000000000000000 ) ) ;
#11027=VERTEX_POINT ( 'NONE', #9570 ) ;
#11045=CARTESIAN_POINT ( 'NONE',  ( 17.29052661994763795, -7.897562529848215718, -4.336808689942017736E-16 ) ) ;
#11049=ORIENTED_EDGE ( 'NONE', *, *, #16873, .F. ) ;
#11071=EDGE_LOOP ( 'NONE', ( #6503, #6801, #14229, #2052 ) ) ;
#11078=ADVANCED_FACE ( 'NONE', ( #2494, #20841 ), #19688, .T. ) ;
#11094=CARTESIAN_POINT ( 'NONE',  ( -24.54452542612009225, -14.48555670042145138, 6.079852602000002548 ) ) ;
#11096=CARTESIAN_POINT ( 'NONE',  ( 18.48839925999793721, 20.72770726368470307, 0.7069223660000067966 ) ) ;
#11107=CARTESIAN_POINT ( 'NONE',  ( -2.507604248437026229, -2.484315071403660813, -0.6999999999999784173 ) ) ;
#11119=CARTESIAN_POINT ( 'NONE',  ( -23.35655559444149887, -15.07705663921310446, 4.319305392000011068 ) ) ;
#11127=CARTESIAN_POINT ( 'NONE',  ( 25.77914806503467560, 15.40383291000323318, 8.000000000000007105 ) ) ;
#11140=CARTESIAN_POINT ( 'NONE',  ( 18.26639035964474900, 11.02001161816309072, -1.000005633855494125E-09 ) ) ;
#11150=AXIS2_PLACEMENT_3D ( 'NONE', #27074, #27224, #13202 ) ;
#11167=CARTESIAN_POINT ( 'NONE',  ( 28.49528339128749366, 0.5184828350247816520, 0.7595836940000044724 ) ) ;
#11169=CARTESIAN_POINT ( 'NONE',  ( 27.16374163455390089, -6.594387936805345518, 8.000000000000007105 ) ) ;
#11171=CARTESIAN_POINT ( 'NONE',  ( 25.72310959295396771, 9.312057329535781136, -0.6999999999999784173 ) ) ;
#11173=CARTESIAN_POINT ( 'NONE',  ( -0.5575288593901739365, -27.79459983365126163, 4.689815098000011062 ) ) ;
#11186=CARTESIAN_POINT ( 'NONE',  ( 20.30396079662882158, 20.00000000004802203, 3.000000000000002665 ) ) ;
#11201=EDGE_CURVE ( 'NONE', #931, #4165, #26519, .T. ) ;
#11214=CARTESIAN_POINT ( 'NONE',  ( -23.97364091617425785, -15.41162529020582994, 5.735001241127421601 ) ) ;
#11224=ORIENTED_EDGE ( 'NONE', *, *, #5724, .F. ) ;
#11241=EDGE_CURVE ( 'NONE', #28672, #11806, #1531, .T. ) ;
#11245=CARTESIAN_POINT ( 'NONE',  ( 1.000415564564199444, -28.48292217093161938, 3.997481721999984750 ) ) ;
#11247=B_SPLINE_CURVE_WITH_KNOTS ( 'NONE', 3,
 ( #678, #24735, #29140, #3019, #15134, #8187 ),
 .UNSPECIFIED., .F., .F.,
 ( 4, 2, 4 ),
 ( 0.000000000000000000, 0.5000000000000000000, 1.000000000000000000 ),
 .UNSPECIFIED. ) ;
#11248=CARTESIAN_POINT ( 'NONE',  ( 26.71513120331084679, 4.908099852734520319, 0.000000000000000000 ) ) ;
#11250=EDGE_CURVE ( 'NONE', #25431, #18612, #19390, .T. ) ;
#11254=EDGE_CURVE ( 'NONE', #14439, #2704, #5110, .T. ) ;
#11264=CARTESIAN_POINT ( 'NONE',  ( -1.783682052191536638, -3.046043134539063946, -0.6999999999999784173 ) ) ;
#11272=CARTESIAN_POINT ( 'NONE',  ( -20.26572724632349320, -21.15151735177849091, 0.9999999979999896205 ) ) ;
#11280=CARTESIAN_POINT ( 'NONE',  ( -28.08055191791969563, 6.526239597828547900, 8.000000000000007105 ) ) ;
#11287=FACE_BOUND ( 'NONE', #27546, .T. ) ;
#11310=ORIENTED_EDGE ( 'NONE', *, *, #29248, .T. ) ;
#11315=EDGE_CURVE ( 'NONE', #13930, #5717, #8049, .T. ) ;
#11330=CARTESIAN_POINT ( 'NONE',  ( -28.47941833768584985, -1.391725289281258160, 8.000000000000007105 ) ) ;
#11332=CARTESIAN_POINT ( 'NONE',  ( 28.35455043824866550, 0.5159221438580620100, 0.2374258030000131470 ) ) ;
#11339=CARTESIAN_POINT ( 'NONE',  ( 17.93011078763067090, 11.79183908526299085, 0.000000000000000000 ) ) ;
#11340=CARTESIAN_POINT ( 'NONE',  ( -23.77307140041805411, 14.41181874028064591, 4.999998581000003384 ) ) ;
#11350=SURFACE_SIDE_STYLE ('',( #27553 ) ) ;
#11369=CARTESIAN_POINT ( 'NONE',  ( 0.5057536231481117861, -27.79562098839016571, 6.099998581000020792 ) ) ;
#11370=CARTESIAN_POINT ( 'NONE',  ( -17.93590711828372974, 11.12626540400258790, -0.6999999999999784173 ) ) ;
#11373=CARTESIAN_POINT ( 'NONE',  ( -24.92013865347427171, 13.82966157970119525, 6.099998581000020792 ) ) ;
#11375=ORIENTED_EDGE ( 'NONE', *, *, #3232, .T. ) ;
#11379=VERTEX_POINT ( 'NONE', #21767 ) ;
#11380=CARTESIAN_POINT ( 'NONE',  ( -23.77307140041805411, 14.41181874028064591, 4.999998581000003384 ) ) ;
#11390=CARTESIAN_POINT ( 'NONE',  ( -25.46368746804859740, 12.80129684245613575, 4.999998581000003384 ) ) ;
#11392=CARTESIAN_POINT ( 'NONE',  ( -23.81866442513186755, -14.33570206443695838, 3.899998581000013509 ) ) ;
#11405=CARTESIAN_POINT ( 'NONE',  ( 24.93720649360215802, -13.79881813812812297, 3.899998581000013509 ) ) ;
#11413=B_SPLINE_CURVE_WITH_KNOTS ( 'NONE', 3,
 ( #16847, #24097, #14349, #2231, #18900, #11825 ),
 .UNSPECIFIED., .F., .F.,
 ( 4, 2, 4 ),
 ( 0.000000000000000000, 0.5000000000000000000, 1.000000000000000000 ),
 .UNSPECIFIED. ) ;
#11417=CARTESIAN_POINT ( 'NONE',  ( -2.813577582307066560, -2.131591337269397979, -0.6999999999999784173 ) ) ;
#11429=CARTESIAN_POINT ( 'NONE',  ( -20.26572724641438228, -21.15151735228022645, 0.8585790890000000175 ) ) ;
#11430=ORIENTED_EDGE ( 'NONE', *, *, #284, .T. ) ;
#11434=CARTESIAN_POINT ( 'NONE',  ( -2.611298560087381038, 2.373819477306434500, 0.000000000000000000 ) ) ;
#11435=B_SPLINE_SURFACE_WITH_KNOTS ( 'NONE', 5, 1, ( 
 ( #30683, #15892 ),
 ( #25495, #26723 ),
 ( #2508, #4555 ),
 ( #9585, #28626 ),
 ( #5161, #16508 ),
 ( #7223, #11637 ),
 ( #23762, #26118 ),
 ( #23922, #12095 ),
 ( #24069, #26576 ),
 ( #21550, #21399 ),
 ( #254, #24213 ),
 ( #16969, #153 ),
 ( #14321, #21703 ),
 ( #17123, #23611 ),
 ( #16813, #9733 ) ),
 .UNSPECIFIED., .F., .F., .F.,
 ( 6, 3, 3, 3, 6 ),
 ( 2, 2 ),
 ( 0.000000000000000000, 0.5778102094429999891, 1.155620418890000112, 2.022335733049999806, 2.889051047220000168 ),
 ( -3.133915349450000281E-11, 0.7031437918980000257 ),
 .UNSPECIFIED. ) ;
#11457=CARTESIAN_POINT ( 'NONE',  ( -17.59696597926837214, -9.791839085300418688, -0.6999999989999727834 ) ) ;
#11464=VERTEX_POINT ( 'NONE', #11951 ) ;
#11478=CARTESIAN_POINT ( 'NONE',  ( 25.20441738229720485, -13.30520055401376922, 5.965619088697175165 ) ) ;
#11486=CARTESIAN_POINT ( 'NONE',  ( 26.91640669801677177, 9.744044393141841454, -0.2432540810000105580 ) ) ;
#11490=EDGE_CURVE ( 'NONE', #17095, #11806, #14488, .T. ) ;
#11491=CARTESIAN_POINT ( 'NONE',  ( -25.46368746804859740, 12.80129684245613575, 4.999998581000003384 ) ) ;
#11505=CARTESIAN_POINT ( 'NONE',  ( -24.16679028379773797, -15.10730798416152609, 3.997250019000003540 ) ) ;
#11507=CARTESIAN_POINT ( 'NONE',  ( -0.5968465743326634154, -28.49391676915515603, 4.791896188000022150 ) ) ;
#11519=DIRECTION ( 'NONE',  ( 0.000000000000000000, 0.000000000000000000, -1.000000000000000000 ) ) ;
#11524=CARTESIAN_POINT ( 'NONE',  ( -16.04158896040112126, -9.763537949678049443, 0.000000000000000000 ) ) ;
#11542=CARTESIAN_POINT ( 'NONE',  ( 24.37821946547973084, -14.76389286113969490, 5.208432824000020389 ) ) ;
#11549=CARTESIAN_POINT ( 'NONE',  ( -18.94275355761817181, 21.23709850871491511, 0.5017677510000262409 ) ) ;
#11550=CYLINDRICAL_SURFACE ( 'NONE', #20064, 1.100000000000002309 ) ;
#11553=CARTESIAN_POINT ( 'NONE',  ( -18.66939278141083136, 19.99991229567540074, -0.6052796912250372197 ) ) ;
#11577=VERTEX_POINT ( 'NONE', #5954 ) ;
#11581=CARTESIAN_POINT ( 'NONE',  ( 24.39448487261446274, -13.33383073951642928, 3.899998581000052145 ) ) ;
#11590=CARTESIAN_POINT ( 'NONE',  ( -0.4846640835643744039, -27.79604706135699033, 4.493528488000025689 ) ) ;
#11594=CARTESIAN_POINT ( 'NONE',  ( 20.30396079662882158, 20.00000000004802203, 3.000000000000002665 ) ) ;
#11604=EDGE_CURVE ( 'NONE', #2594, #25714, #17091, .T. ) ;
#11615=ORIENTED_EDGE ( 'NONE', *, *, #11993, .T. ) ;
#11623=CARTESIAN_POINT ( 'NONE',  ( -24.32472894358752313, 13.45989150749028873, 6.099998581000020792 ) ) ;
#11634=CARTESIAN_POINT ( 'NONE',  ( 28.22605159097494010, -9.791255285991017132, -0.2432540810000105580 ) ) ;
#11636=CARTESIAN_POINT ( 'NONE',  ( -27.79539923781770128, -0.5057481688779102980, 8.000000000000007105 ) ) ;
#11637=CARTESIAN_POINT ( 'NONE',  ( -19.56375666326936269, 19.56885676738829005, 0.5004811919999962999 ) ) ;
#11638=CARTESIAN_POINT ( 'NONE',  ( 28.03861306157277866, 0.5101735396241825482, -0.2432540810000105580 ) ) ;
#11639=EDGE_CURVE ( 'NONE', #24853, #6068, #18196, .T. ) ;
#11645=EDGE_LOOP ( 'NONE', ( #3590, #23663, #9091, #2232 ) ) ;
#11650=VERTEX_POINT ( 'NONE', #30031 ) ;
#11658=CARTESIAN_POINT ( 'NONE',  ( 23.87963657767028280, 15.55698410313905988, 4.493007569000006640 ) ) ;
#11659=CARTESIAN_POINT ( 'NONE',  ( -23.81776757772072983, -15.65134804123479917, 4.999998581000003384 ) ) ;
#11661=CARTESIAN_POINT ( 'NONE',  ( 19.55507467582014414, 20.00006801630439668, -0.2385979495973736264 ) ) ;
#11676=CARTESIAN_POINT ( 'NONE',  ( 1.413941964927726946, -28.46527362969718311, 5.680166690000016061 ) ) ;
#11681=ORIENTED_EDGE ( 'NONE', *, *, #17819, .T. ) ;
#11686=CARTESIAN_POINT ( 'NONE',  ( 24.36375418468539067, 14.78716628296302282, 3.904032100999987875 ) ) ;
#11693=CARTESIAN_POINT ( 'NONE',  ( 24.74993095452947856, -14.13250376044891965, 6.042507811999997536 ) ) ;
#11699=CARTESIAN_POINT ( 'NONE',  ( 17.95841148951064525, -9.763538383420391042, -0.6999999989999727834 ) ) ;
#11704=CARTESIAN_POINT ( 'NONE',  ( -18.63748837690081572, 19.99991059812205307, -0.6126749037462432268 ) ) ;
#11711=CARTESIAN_POINT ( 'NONE',  ( 1.379247882464924579, -27.76613141686495823, 4.319830470999985295 ) ) ;
#11712=CARTESIAN_POINT ( 'NONE',  ( 18.23234009272960776, 11.30637938200976045, -0.6999999999999785283 ) ) ;
#11713=CARTESIAN_POINT ( 'NONE',  ( -23.23277431133845994, -15.26692929363520257, 4.999998581000003384 ) ) ;
#11725=CARTESIAN_POINT ( 'NONE',  ( 16.40303402075260308, 10.20816091466531716, -0.6999999999999784173 ) ) ;
#11729=CARTESIAN_POINT ( 'NONE',  ( 1.495522319887057749, -27.76012052182125345, 4.493506933999996455 ) ) ;
#11732=CARTESIAN_POINT ( 'NONE',  ( -27.66290831536099759, -7.787312998881454895, 1.000000000000000888 ) ) ;
#11735=CARTESIAN_POINT ( 'NONE',  ( 17.73945528632581059, -9.950349630033622716, -0.6999999999999784173 ) ) ;
#11767=ORIENTED_EDGE ( 'NONE', *, *, #23494, .F. ) ;
#11776=CARTESIAN_POINT ( 'NONE',  ( -25.38146355688813216, 12.59839640969179975, 6.600000000000022737 ) ) ;
#11778=CARTESIAN_POINT ( 'NONE',  ( -26.79556473285982321, -0.4875557887250224209, 0.000000000000000000 ) ) ;
#11780=CARTESIAN_POINT ( 'NONE',  ( -19.80535357377644701, 19.50875577052588739, 1.000000000000000888 ) ) ;
#11785=EDGE_CURVE ( 'NONE', #4633, #25869, #26134, .T. ) ;
#11796=CARTESIAN_POINT ( 'NONE',  ( -24.98081131316241255, -13.71897606304888662, 5.104178996000019453 ) ) ;
#11806=VERTEX_POINT ( 'NONE', #6737 ) ;
#11810=CARTESIAN_POINT ( 'NONE',  ( -17.49227996845844402, -9.885041018070451102, 0.000000000000000000 ) ) ;
#11825=CARTESIAN_POINT ( 'NONE',  ( 17.95841148951064525, -9.763538383420391042, 0.000000000000000000 ) ) ;
#11832=CARTESIAN_POINT ( 'NONE',  ( 24.34942395457898101, 13.41447635819141126, 5.310538874999992665 ) ) ;
#11837=CARTESIAN_POINT ( 'NONE',  ( -17.62526668104891314, 11.76353838341477953, -0.6999999999999784173 ) ) ;
#11866=CARTESIAN_POINT ( 'NONE',  ( 1.533144572060379796, -28.45911136072525238, 4.493506933999996455 ) ) ;
#11867=CARTESIAN_POINT ( 'NONE',  ( 25.79280520781986041, 13.25682296313440389, 1.000000000000000888 ) ) ;
#11872=ORIENTED_EDGE ( 'NONE', *, *, #16040, .F. ) ;
#11883=CARTESIAN_POINT ( 'NONE',  ( 23.97364091749897952, 15.41162527761334289, 5.735001252146398443 ) ) ;
#11890=CARTESIAN_POINT ( 'NONE',  ( -23.69427943501400691, -14.54081806258934861, 3.920145809000019632 ) ) ;
#11896=EDGE_CURVE ( 'NONE', #30472, #19387, #7816, .T. ) ;
#11909=CARTESIAN_POINT ( 'NONE',  ( 17.29283780512531621, -7.897520476889244634, -0.6999999999999784173 ) ) ;
#11910=CARTESIAN_POINT ( 'NONE',  ( 24.66346747934004568, 14.28208995973567141, 6.002748562000004284 ) ) ;
#11923=FACE_OUTER_BOUND ( 'NONE', #23120, .T. ) ;
#11929=CARTESIAN_POINT ( 'NONE',  ( 14.25032083441342934, -27.35421241409322946, 1.000000000000000888 ) ) ;
#11935=EDGE_CURVE ( 'NONE', #20235, #17095, #4728, .T. ) ;
#11938=CARTESIAN_POINT ( 'NONE',  ( 18.26639035964474900, 11.02001161816309072, -0.6999999999999784173 ) ) ;
#11945=ADVANCED_FACE ( 'NONE', ( #11923 ), #5101, .T. ) ;
#11951=CARTESIAN_POINT ( 'NONE',  ( 16.37473331889771089, 11.76353838340827984, -0.6999999999999784173 ) ) ;
#11955=CARTESIAN_POINT ( 'NONE',  ( 25.44662323365202639, -12.83524168329857318, 4.689351482000003735 ) ) ;
#11978=CARTESIAN_POINT ( 'NONE',  ( 19.68707593455170368, 19.53815609463533320, 0.6304112420000007599 ) ) ;
#11982=CARTESIAN_POINT ( 'NONE',  ( 23.89202021435673728, -14.21382295584061417, 5.677594575767613172 ) ) ;
#11993=EDGE_CURVE ( 'NONE', #24893, #21140, #26847, .T. ) ;
#11997=ORIENTED_EDGE ( 'NONE', *, *, #17550, .T. ) ;
#12003=CARTESIAN_POINT ( 'NONE',  ( 28.49528339128749366, 0.5184828350247212558, 1.000000000000000888 ) ) ;
#12008=CARTESIAN_POINT ( 'NONE',  ( 18.62349342026574917, 19.80369317695730302, 0.06728435000000199118 ) ) ;
#12018=EDGE_LOOP ( 'NONE', ( #12855, #8143, #20774, #3833 ) ) ;
#12019=CARTESIAN_POINT ( 'NONE',  ( 16.29938252758261186, 10.30810785441514454, -0.6999999999999783062 ) ) ;
#12025=CARTESIAN_POINT ( 'NONE',  ( 0.5184513693225318853, -28.49550581263314086, 3.899998581000013509 ) ) ;
#12055=FACE_OUTER_BOUND ( 'NONE', #12123, .T. ) ;
#12063=B_SPLINE_CURVE_WITH_KNOTS ( 'NONE', 1,
 ( #22161, #3108 ),
 .UNSPECIFIED., .F., .F.,
 ( 2, 2 ),
 ( -2.556331299420000144E-06, 0.7000000000009999335 ),
 .UNSPECIFIED. ) ;
#12068=DIRECTION ( 'NONE',  ( 0.000000000000000000, 0.000000000000000000, -1.000000000000000000 ) ) ;
#12081=CARTESIAN_POINT ( 'NONE',  ( -27.07233446881437899, 8.380004974182886812, 8.000000000000007105 ) ) ;
#12095=CARTESIAN_POINT ( 'NONE',  ( -19.29841003509485375, 19.63499152630128108, 0.3044381840000276451 ) ) ;
#12099=EDGE_CURVE ( 'NONE', #3424, #21696, #30941, .T. ) ;
#12100=CARTESIAN_POINT ( 'NONE',  ( -16.83342759575507586, 10.99999999997565503, -0.6999999999999784173 ) ) ;
#12101=ORIENTED_EDGE ( 'NONE', *, *, #18448, .F. ) ;
#12104=ORIENTED_EDGE ( 'NONE', *, *, #805, .T. ) ;
#12118=CARTESIAN_POINT ( 'NONE',  ( 18.12303402403091113, 19.99995697021033081, -0.6894527066783940894 ) ) ;
#12120=CARTESIAN_POINT ( 'NONE',  ( -24.32472894358752313, 13.45989150749028873, 6.099998581000020792 ) ) ;
#12122=CARTESIAN_POINT ( 'NONE',  ( -24.05392374927932053, 13.13253365033636477, -0.6999999999999784173 ) ) ;
#12123=EDGE_LOOP ( 'NONE', ( #6887, #10182, #29753, #21888 ) ) ;
#12127=CARTESIAN_POINT ( 'NONE',  ( -2.635643612059070051, -2.346759556412466363, 0.000000000000000000 ) ) ;
#12135=CARTESIAN_POINT ( 'NONE',  ( -24.41841039498785193, -14.69667350221323865, 3.899998581000013509 ) ) ;
#12143=CARTESIAN_POINT ( 'NONE',  ( 24.16679028237082960, 15.10730797463399000, 3.997250016000014838 ) ) ;
#12146=ORIENTED_EDGE ( 'NONE', *, *, #24678, .T. ) ;
#12150=FACE_OUTER_BOUND ( 'NONE', #1051, .T. ) ;
#12151=CARTESIAN_POINT ( 'NONE',  ( 16.63016908737474253, 10.02891580959015094, -0.6999999999999784173 ) ) ;
#12153=CARTESIAN_POINT ( 'NONE',  ( -24.83827471527357744, 12.48687850854618198, 5.104216618000034345 ) ) ;
#12155=LINE ( 'NONE', #11699, #22588 ) ;
#12178=CARTESIAN_POINT ( 'NONE',  ( 23.81866173088643635, 14.33570044285385947, 6.099998581000020792 ) ) ;
#12183=APPLICATION_CONTEXT ( 'automotive_design' ) ;
#12192=CARTESIAN_POINT ( 'NONE',  ( 17.47295178719334530, -10.06576768799940247, -0.6999999999999785283 ) ) ;
#12193=B_SPLINE_SURFACE_WITH_KNOTS ( 'NONE', 5, 1, ( 
 ( #23893, #4987 ),
 ( #29202, #14598 ),
 ( #7040, #126 ),
 ( #286, #21829 ),
 ( #17246, #26853 ),
 ( #19466, #24187 ) ),
 .UNSPECIFIED., .F., .F., .F.,
 ( 6, 6 ),
 ( 2, 2 ),
 ( 0.000000000000000000, 2.000000000000000000 ),
 ( -2.345346139519999876E-15, 0.7000000000189999794 ),
 .UNSPECIFIED. ) ;
#12209=CARTESIAN_POINT ( 'NONE',  ( 14.37503218006001049, -27.59354456826596191, -0.2432540810000105580 ) ) ;
#12211=DIRECTION ( 'NONE',  ( 0.000000000000000000, 0.000000000000000000, -1.000000000000000000 ) ) ;
#12216=CARTESIAN_POINT ( 'NONE',  ( 24.43659368183839931, 14.66646236428692340, 6.099998581000020792 ) ) ;
#12219=CARTESIAN_POINT ( 'NONE',  ( 19.80526555972147307, 19.50877392102524155, 3.000000000000002665 ) ) ;
#12225=ORIENTED_EDGE ( 'NONE', *, *, #21114, .T. ) ;
#12229=ORIENTED_EDGE ( 'NONE', *, *, #21977, .T. ) ;
#12232=CARTESIAN_POINT ( 'NONE',  ( -23.77947513073445407, 14.40125622634048774, 4.791564337000009388 ) ) ;
#12236=CARTESIAN_POINT ( 'NONE',  ( -20.30403093128963476, 20.00000000003735323, 3.000000106999994642 ) ) ;
#12246=CARTESIAN_POINT ( 'NONE',  ( -15.77518214703643729, -8.674270198554944855, 0.000000000000000000 ) ) ;
#12252=AXIS2_PLACEMENT_3D ( 'NONE', #9347, #16277, #14237 ) ;
#12271=EDGE_LOOP ( 'NONE', ( #601, #29097, #24843, #5485 ) ) ;
#12288=CARTESIAN_POINT ( 'NONE',  ( 3.040504021322313122, 1.733590290792417887, 0.000000000000000000 ) ) ;
#12290=CARTESIAN_POINT ( 'NONE',  ( 23.77307140678977504, -14.41181874416537134, 5.104215870000011535 ) ) ;
#12291=CARTESIAN_POINT ( 'NONE',  ( 24.05769993097117876, 13.93129956312566620, 6.002748562000004284 ) ) ;
#12296=CARTESIAN_POINT ( 'NONE',  ( -24.36724936496760918, -13.38201651699120021, 4.999998581000003384 ) ) ;
#12310=EDGE_CURVE ( 'NONE', #974, #8453, #13693, .T. ) ;
#12311=ORIENTED_EDGE ( 'NONE', *, *, #29602, .F. ) ;
#12324=ORIENTED_EDGE ( 'NONE', *, *, #17270, .T. ) ;
#12339=CARTESIAN_POINT ( 'NONE',  ( -28.49530731802708416, -0.5184832703812605192, 8.000000000000007105 ) ) ;
#12346=( NAMED_UNIT ( * ) SI_UNIT ( $, .STERADIAN. ) SOLID_ANGLE_UNIT ( ) );
#12349=CARTESIAN_POINT ( 'NONE',  ( 1.157672466085042151, -27.77645868488912484, 4.099089508000003157 ) ) ;
#12365=CARTESIAN_POINT ( 'NONE',  ( -24.36375527493646942, -13.38839014155000129, 4.854229180514668229 ) ) ;
#12367=CARTESIAN_POINT ( 'NONE',  ( -17.32140263436448890, -8.004506215797992041, 0.000000000000000000 ) ) ;
#12368=CARTESIAN_POINT ( 'NONE',  ( -27.16361495901510636, -7.646758255380050606, -0.6577119969999878357 ) ) ;
#12370=CARTESIAN_POINT ( 'NONE',  ( -28.35945636601969611, -7.983396444588293228, 8.000000000000007105 ) ) ;
#12371=CARTESIAN_POINT ( 'NONE',  ( 17.93011078763067090, 11.79183908526299085, 0.000000000000000000 ) ) ;
#12379=EDGE_CURVE ( 'NONE', #6771, #16061, #3150, .T. ) ;
#12380=B_SPLINE_CURVE_WITH_KNOTS ( 'NONE', 5,
 ( #21559, #7233, #9592, #13855, #23463, #1897, #13328, #6557, #20411, #30493, #3892, #22770 ),
 .UNSPECIFIED., .F., .F.,
 ( 6, 3, 3, 6 ),
 ( 1.224410036190000106, 1.456395025189999970, 2.184590866520000230, 2.448622045610000075 ),
 .UNSPECIFIED. ) ;
#12389=DIRECTION ( 'NONE',  ( 0.000000000000000000, 0.000000000000000000, -1.000000000000000000 ) ) ;
#12391=B_SPLINE_SURFACE_WITH_KNOTS ( 'NONE', 5, 1, ( 
 ( #19409, #1097 ),
 ( #5813, #15257 ),
 ( #24704, #3142 ),
 ( #22505, #28998 ),
 ( #5503, #28837 ),
 ( #27517, #8012 ) ),
 .UNSPECIFIED., .F., .F., .F.,
 ( 6, 6 ),
 ( 2, 2 ),
 ( 0.000000000000000000, 7.118283443510000197 ),
 ( -0.7000000000080000007, 0.0003775010496399999857 ),
 .UNSPECIFIED. ) ;
#12403=CARTESIAN_POINT ( 'NONE',  ( -16.06988964647317886, -8.208161364834239748, 0.000000000000000000 ) ) ;
#12406=CARTESIAN_POINT ( 'NONE',  ( -15.73360964030186970, 11.02001161816959396, -1.000005633855494125E-09 ) ) ;
#12422=CYLINDRICAL_SURFACE ( 'NONE', #27043, 1.100000000000002309 ) ;
#12429=CARTESIAN_POINT ( 'NONE',  ( -24.70074544867652122, 14.21822122508601716, 6.002806299999996043 ) ) ;
#12435=CARTESIAN_POINT ( 'NONE',  ( 24.39135169777336287, -14.74223403354865347, 5.310643619999999565 ) ) ;
#12436=CARTESIAN_POINT ( 'NONE',  ( 24.92639507930385889, 13.81781707913292934, 5.506973475999988210 ) ) ;
#12442=CARTESIAN_POINT ( 'NONE',  ( -24.36724936496760918, -13.38201651699120021, 4.895818166000015736 ) ) ;
#12443=CARTESIAN_POINT ( 'NONE',  ( 16.06413493398061476, 11.12395421528300865, -4.336808689942017736E-16 ) ) ;
#12457=ORIENTED_EDGE ( 'NONE', *, *, #3090, .F. ) ;
#12460=CARTESIAN_POINT ( 'NONE',  ( 18.26377084491840463, -8.836022547968246599, -4.336808689942018722E-16 ) ) ;
#12462=CARTESIAN_POINT ( 'NONE',  ( -24.63375100851393640, 12.88633854783081922, 5.901400367999992902 ) ) ;
#12486=CARTESIAN_POINT ( 'NONE',  ( -18.44984504927483471, 20.68447211616248893, 0.5514271140000248650 ) ) ;
#12494=CARTESIAN_POINT ( 'NONE',  ( 24.34246741410084880, 14.82285105323827779, 6.099998581000033226 ) ) ;
#12509=ORIENTED_EDGE ( 'NONE', *, *, #9865, .T. ) ;
#12511=CARTESIAN_POINT ( 'NONE',  ( -24.98081131316241255, -13.71897606304888662, 5.104178996000019453 ) ) ;
#12512=CARTESIAN_POINT ( 'NONE',  ( -23.23955040174346465, -15.25661106733265981, 5.208368890000008911 ) ) ;
#12521=EDGE_CURVE ( 'NONE', #4471, #18763, #11413, .T. ) ;
#12531=ADVANCED_FACE ( 'NONE', ( #28653 ), #4897, .F. ) ;
#12540=CARTESIAN_POINT ( 'NONE',  ( -24.88589369081283920, 13.89120818323882922, 3.904029272000009154 ) ) ;
#12548=VERTEX_POINT ( 'NONE', #24403 ) ;
#12550=CARTESIAN_POINT ( 'NONE',  ( 17.18658402238548533, 9.900182044515950963, -0.6999999999999784173 ) ) ;
#12571=EDGE_LOOP ( 'NONE', ( #21763, #9959, #12324, #17215 ) ) ;
#12577=CARTESIAN_POINT ( 'NONE',  ( 24.98081130624543889, 13.71897605842228529, 4.895818164000031558 ) ) ;
#12578=CARTESIAN_POINT ( 'NONE',  ( 27.75695160380879045, 2.618790587931635994, 1.000000000000000888 ) ) ;
#12592=CARTESIAN_POINT ( 'NONE',  ( 20.15233751852803579, 20.00000015395470498, 0.3716988990000169579 ) ) ;
#12601=CARTESIAN_POINT ( 'NONE',  ( -15.73360964030186970, 11.02001161816959396, -0.6999999989999727834 ) ) ;
#12608=ORIENTED_EDGE ( 'NONE', *, *, #14825, .F. ) ;
#12615=ORIENTED_EDGE ( 'NONE', *, *, #17550, .F. ) ;
#12616=CARTESIAN_POINT ( 'NONE',  ( -24.36725163763869162, -13.38201776504303986, 4.999998581000003384 ) ) ;
#12618=CARTESIAN_POINT ( 'NONE',  ( 0.03635086293632015797, -28.50041301604635180, 6.002517553000020101 ) ) ;
#12620=CARTESIAN_POINT ( 'NONE',  ( -19.80535357367646654, 19.50875577052770993, 1.800000043000016259 ) ) ;
#12633=VERTEX_POINT ( 'NONE', #22192 ) ;
#12636=CARTESIAN_POINT ( 'NONE',  ( -18.50495978126638619, 20.74626080822700658, 0.8585787019999846503 ) ) ;
#12647=CARTESIAN_POINT ( 'NONE',  ( 23.69427943123108093, 14.54081805611945910, 6.079851352999988023 ) ) ;
#12651=EDGE_CURVE ( 'NONE', #26737, #3218, #20045, .T. ) ;
#12653=CARTESIAN_POINT ( 'NONE',  ( -26.44963151265186241, 8.939294038675827281, -0.6577119969999878357 ) ) ;
#12654=CARTESIAN_POINT ( 'NONE',  ( 24.83827260360999389, -12.48687744688666967, 4.999998581000003384 ) ) ;
#12655=CARTESIAN_POINT ( 'NONE',  ( -28.49530731802708416, -0.5184832703812605192, 8.000000000000007105 ) ) ;
#12656=CARTESIAN_POINT ( 'NONE',  ( -27.87609112763790975, 3.928995115430390150, 1.000000000000000888 ) ) ;
#12657=ORIENTED_EDGE ( 'NONE', *, *, #2234, .F. ) ;
#12671=CARTESIAN_POINT ( 'NONE',  ( -20.09263842094486208, -20.97086228454488932, -0.5592437529999827461 ) ) ;
#12677=CARTESIAN_POINT ( 'NONE',  ( -0.5968465743326634154, -28.49391676915515603, 5.208100973000007627 ) ) ;
#12678=ORIENTED_EDGE ( 'NONE', *, *, #6449, .T. ) ;
#12687=EDGE_LOOP ( 'NONE', ( #6706, #1123, #15365, #11997 ) ) ;
#12692=CARTESIAN_POINT ( 'NONE',  ( 25.16696686177720821, -13.37570800343109312, 3.997190761000024573 ) ) ;
#12694=CARTESIAN_POINT ( 'NONE',  ( -27.79539923451739014, -0.5057481688648817197, 8.000000000000007105 ) ) ;
#12695=CARTESIAN_POINT ( 'NONE',  ( 24.78870453580057998, -12.58522324566301620, 5.507123706999989210 ) ) ;
#12696=CARTESIAN_POINT ( 'NONE',  ( 14.25032083441342934, -27.35421241409322946, 8.000000000000007105 ) ) ;
#12697=ORIENTED_EDGE ( 'NONE', *, *, #1482, .T. ) ;
#12704=CARTESIAN_POINT ( 'NONE',  ( -16.66945014389299828, 9.902801559243821217, -4.336808689942018722E-16 ) ) ;
#12727=ORIENTED_EDGE ( 'NONE', *, *, #22408, .T. ) ;
#12732=CARTESIAN_POINT ( 'NONE',  ( 23.94167923218795124, 14.12976891115827627, 3.920144559000027229 ) ) ;
#12739=CARTESIAN_POINT ( 'NONE',  ( -26.79556473285982321, -0.4875557887251183442, -0.6999999999999784173 ) ) ;
#12753=LINE ( 'NONE', #3781, #3179 ) ;
#12755=EDGE_LOOP ( 'NONE', ( #12146, #16252, #29408, #28819 ) ) ;
#12777=CARTESIAN_POINT ( 'NONE',  ( -24.93720648713954446, 13.79881813474513486, 6.099998581000020792 ) ) ;
#12802=CARTESIAN_POINT ( 'NONE',  ( -16.60222294797364029, -7.918137930465035446, 0.000000000000000000 ) ) ;
#12806=VERTEX_POINT ( 'NONE', #5463 ) ;
#12807=B_SPLINE_CURVE_WITH_KNOTS ( 'NONE', 3,
 ( #2603, #2308, #12192, #11735, #21963, #103 ),
 .UNSPECIFIED., .F., .F.,
 ( 4, 2, 4 ),
 ( 0.000000000000000000, 0.5000000000000000000, 1.000000000000000000 ),
 .UNSPECIFIED. ) ;
#12811=DIRECTION ( 'NONE',  ( -0.7198537139083028835, 0.6941258031311204890, 0.000000000000000000 ) ) ;
#12819=CARTESIAN_POINT ( 'NONE',  ( -27.47766015528786454, 9.286741218802717412, 0.2374258030000131470 ) ) ;
#12824=ORIENTED_EDGE ( 'NONE', *, *, #1777, .F. ) ;
#12826=CARTESIAN_POINT ( 'NONE',  ( 24.93720649360215802, -13.79881813812812297, 3.899998581000013509 ) ) ;
#12831=CARTESIAN_POINT ( 'NONE',  ( -24.25742564193969031, -13.58028021372842531, 5.680679499000030219 ) ) ;
#12836=CARTESIAN_POINT ( 'NONE',  ( -28.35945636591989683, -7.983396444576476902, 1.000000000000000888 ) ) ;
#12842=ADVANCED_FACE ( 'NONE', ( #24203 ), #5006, .F. ) ;
#12844=CARTESIAN_POINT ( 'NONE',  ( -0.6094664100040195764, -28.49364619262437870, 5.104049977999985721 ) ) ;
#12852=CARTESIAN_POINT ( 'NONE',  ( 23.25025823367671407, -19.81038070381301353, 0.2686784570000155803 ) ) ;
#12855=ORIENTED_EDGE ( 'NONE', *, *, #23724, .T. ) ;
#12859=CARTESIAN_POINT ( 'NONE',  ( -25.24918301675066346, 13.28546534817111180, 8.000000000000007105 ) ) ;
#12872=EDGE_CURVE ( 'NONE', #16829, #3809, #3479, .T. ) ;
#12889=CARTESIAN_POINT ( 'NONE',  ( 16.27478637889808510, -8.340113109526685164, -4.336808689942018722E-16 ) ) ;
#12890=CARTESIAN_POINT ( 'NONE',  ( 24.75645985066740806, 14.12045945716145390, 4.098702612000016288 ) ) ;
#12899=CARTESIAN_POINT ( 'NONE',  ( -18.25755939615993739, 19.99998186964045743, -0.6768317722208874176 ) ) ;
#12904=CARTESIAN_POINT ( 'NONE',  ( 16.89916710617796625, 9.923792022417691427, -0.000000000000000000 ) ) ;
#12921=CARTESIAN_POINT ( 'NONE',  ( 17.93011078765611543, -8.208160914697428368, -0.6999999989999727834 ) ) ;
#12930=CARTESIAN_POINT ( 'NONE',  ( -24.44015551247796836, 13.24969167840070483, 6.079865069000017996 ) ) ;
#12932=CARTESIAN_POINT ( 'NONE',  ( 20.77600629932058851, 21.68409807857665683, 8.000000000000007105 ) ) ;
#12942=CARTESIAN_POINT ( 'NONE',  ( 24.35364645778183146, 13.40687562030597135, 5.286753706817813203 ) ) ;
#12947=CARTESIAN_POINT ( 'NONE',  ( -2.131591337306473655, 2.813577582285920364, -0.6999999999999784173 ) ) ;
#12952=CARTESIAN_POINT ( 'NONE',  ( 16.40303402075260308, 10.20816091466531716, -0.6999999989999727834 ) ) ;
#12954=CARTESIAN_POINT ( 'NONE',  ( -18.13789968716447731, 20.33475262164161279, 0.08279786600001726171 ) ) ;
#12963=CARTESIAN_POINT ( 'NONE',  ( 23.57322167201318663, 14.73624931494496693, 6.002747145999992817 ) ) ;
#12967=CARTESIAN_POINT ( 'NONE',  ( -26.87967798701711786, 4.135222155429991275, -0.6999999999999784173 ) ) ;
#12968=DIRECTION ( 'NONE',  ( 0.7198537139083028835, -0.6941258031311204890, 0.000000000000000000 ) ) ;
#12977=CARTESIAN_POINT ( 'NONE',  ( -24.41841039498785193, -14.69667350221323865, 6.099998581000020792 ) ) ;
#12982=CARTESIAN_POINT ( 'NONE',  ( -16.95618186250884563, -7.902051487308459521, 0.000000000000000000 ) ) ;
#12983=CARTESIAN_POINT ( 'NONE',  ( -23.57322167415998138, -14.73624932338542060, 6.002747143000003227 ) ) ;
#12985=EDGE_CURVE ( 'NONE', #13797, #11464, #13323, .T. ) ;
#12990=CARTESIAN_POINT ( 'NONE',  ( 0.4024591535012043697, -27.79733476277325721, 6.095949245000009675 ) ) ;
#13001=CARTESIAN_POINT ( 'NONE',  ( 23.01145998759524858, -19.60693125301565232, 0.08279965200003180925 ) ) ;
#13002=EDGE_LOOP ( 'NONE', ( #9322, #12608, #18918, #29972 ) ) ;
#13008=CARTESIAN_POINT ( 'NONE',  ( 25.35851007746311581, -13.00862288856444238, 5.680831396999986183 ) ) ;
#13037=CARTESIAN_POINT ( 'NONE',  ( 24.54452541844319668, 14.48555669908156851, 3.920144559000027229 ) ) ;
#13038=ADVANCED_FACE ( 'NONE', ( #13158 ), #5772, .F. ) ;
#13039=CARTESIAN_POINT ( 'NONE',  ( -0.4442473836104618434, -27.79664838810757743, 5.558326393341954663 ) ) ;
#13053=CARTESIAN_POINT ( 'NONE',  ( -25.77914833258148164, -15.40383343755785361, 1.000000000000000888 ) ) ;
#13083=CARTESIAN_POINT ( 'NONE',  ( -17.62526668104891314, 11.76353838341477953, -0.6999999989999727834 ) ) ;
#13090=B_SPLINE_CURVE_WITH_KNOTS ( 'NONE', 1,
 ( #732, #7635 ),
 .UNSPECIFIED., .F., .F.,
 ( 2, 2 ),
 ( -3.500000000000000000, 3.500000000000000000 ),
 .UNSPECIFIED. ) ;
#13095=ORIENTED_EDGE ( 'NONE', *, *, #21350, .T. ) ;
#13098=EDGE_CURVE ( 'NONE', #12806, #16634, #15865, .T. ) ;
#13100=CARTESIAN_POINT ( 'NONE',  ( -26.25085564088219670, 8.872172082313914743, 0.02487529700001545052 ) ) ;
#13108=CARTESIAN_POINT ( 'NONE',  ( -24.92013865347427171, 13.82966157970119525, 3.899998581000013509 ) ) ;
#13110=DIRECTION ( 'NONE',  ( 0.000000000000000000, 0.000000000000000000, -1.000000000000000000 ) ) ;
#13112=CARTESIAN_POINT ( 'NONE',  ( 1.407377285053368787, -28.46552657486722637, 5.679668080906079553 ) ) ;
#13115=CARTESIAN_POINT ( 'NONE',  ( -24.05392374927932053, 13.13253365033636477, -0.6999999999999784173 ) ) ;
#13119=CARTESIAN_POINT ( 'NONE',  ( -24.97129468253034545, 13.73710443232325495, 3.901342130000013064 ) ) ;
#13126=CARTESIAN_POINT ( 'NONE',  ( 16.37473331892315542, -8.236461616552139375, -0.6999999999999784173 ) ) ;
#13129=CARTESIAN_POINT ( 'NONE',  ( 21.90431914205521124, 17.68079901892130579, 0.7069222299999899928 ) ) ;
#13139=CARTESIAN_POINT ( 'NONE',  ( 0.03635086293632015797, -28.50041301604635180, 6.002517553000020101 ) ) ;
#13149=EDGE_CURVE ( 'NONE', #7951, #4165, #18872, .T. ) ;
#13150=CARTESIAN_POINT ( 'NONE',  ( 27.77052805885498898, 0.5052956280874429940, 0.7069222069999991920 ) ) ;
#13153=CARTESIAN_POINT ( 'NONE',  ( 16.86019302162820921, 12.06576768788192489, -0.6999999999999785283 ) ) ;
#13154=CARTESIAN_POINT ( 'NONE',  ( 25.25401215818320821, -13.21081861402980273, 4.098596794000014754 ) ) ;
#13158=FACE_OUTER_BOUND ( 'NONE', #20162, .T. ) ;
#13160=CARTESIAN_POINT ( 'NONE',  ( -14.60916135985672071, 28.04296594682689658, 1.000000000000000888 ) ) ;
#13182=VERTEX_POINT ( 'NONE', #21041 ) ;
#13184=ORIENTED_EDGE ( 'NONE', *, *, #30800, .F. ) ;
#13189=CARTESIAN_POINT ( 'NONE',  ( -16.29518228631965826, -8.030294604068396680, -0.6999999999999785283 ) ) ;
#13198=CARTESIAN_POINT ( 'NONE',  ( 17.18658402238548533, 9.900182044515950963, -1.000005633855494125E-09 ) ) ;
#13202=DIRECTION ( 'NONE',  ( -0.7198537139083028835, 0.6941258031311204890, 0.000000000000000000 ) ) ;
#13204=CARTESIAN_POINT ( 'NONE',  ( 17.83931306984926835, 20.00000000000176570, -0.6999999999999784173 ) ) ;
#13206=CARTESIAN_POINT ( 'NONE',  ( 21.28666574344908469, 18.00484885041732142, 1.000000000000000888 ) ) ;
#13207=ORIENTED_EDGE ( 'NONE', *, *, #19248, .F. ) ;
#13210=CARTESIAN_POINT ( 'NONE',  ( 23.57322167201318663, 14.73624931494496693, 6.002747145999992817 ) ) ;
#13218=DIRECTION ( 'NONE',  ( 0.000000000000000000, 0.000000000000000000, -1.000000000000000000 ) ) ;
#13222=CARTESIAN_POINT ( 'NONE',  ( 16.40303402077768169, -9.791839085275103827, 0.000000000000000000 ) ) ;
#13226=CARTESIAN_POINT ( 'NONE',  ( -24.37450209798932477, 13.36961646417070249, 6.095967861000000987 ) ) ;
#13289=CARTESIAN_POINT ( 'NONE',  ( -20.30403093128963476, 20.00000000003735323, 3.000000106999994642 ) ) ;
#13291=CARTESIAN_POINT ( 'NONE',  ( 24.71356588429571488, 13.94368305209927428, 1.000000000000000888 ) ) ;
#13312=B_SPLINE_CURVE_WITH_KNOTS ( 'NONE', 1,
 ( #10553, #8020 ),
 .UNSPECIFIED., .F., .F.,
 ( 2, 2 ),
 ( -3.500000000000000000, 3.500000000000000000 ),
 .UNSPECIFIED. ) ;
#13313=CARTESIAN_POINT ( 'NONE',  ( -19.63983047447944941, -20.49826324463772664, 0.000000000000000000 ) ) ;
#13315=CARTESIAN_POINT ( 'NONE',  ( -23.81776757772072983, -15.65134804123479917, 4.895813258999987205 ) ) ;
#13317=CARTESIAN_POINT ( 'NONE',  ( 1.108738578190967550, 3.350312884103880950, 0.000000000000000000 ) ) ;
#13323=LINE ( 'NONE', #29693, #6986 ) ;
#13328=CARTESIAN_POINT ( 'NONE',  ( -17.87802153471533018, -8.632840205466846939, 0.000000000000000000 ) ) ;
#13348=ORIENTED_EDGE ( 'NONE', *, *, #23730, .F. ) ;
#13352=CARTESIAN_POINT ( 'NONE',  ( 23.83639842146205368, 14.30623132797946084, 3.899998581000013509 ) ) ;
#13353=CARTESIAN_POINT ( 'NONE',  ( 17.18658402238548533, 9.900182044515950963, -1.000005633855494125E-09 ) ) ;
#13365=CARTESIAN_POINT ( 'NONE',  ( 19.18333294668393307, 19.99999946087643465, -0.4459674450000006285 ) ) ;
#13367=CARTESIAN_POINT ( 'NONE',  ( -26.33250508584143290, -9.378843469325163440, 8.000000000000007105 ) ) ;
#13371=CARTESIAN_POINT ( 'NONE',  ( 18.97091132402077562, 21.26865671814604752, 1.000000000000000888 ) ) ;
#13385=ORIENTED_EDGE ( 'NONE', *, *, #15472, .F. ) ;
#13392=CARTESIAN_POINT ( 'NONE',  ( 17.70297572270220243, -8.028915810492925687, -4.336808689942018722E-16 ) ) ;
#13397=B_SPLINE_CURVE_WITH_KNOTS ( 'NONE', 3,
 ( #27560, #15453, #3332, #26955, #8354, #7746 ),
 .UNSPECIFIED., .F., .F.,
 ( 4, 2, 4 ),
 ( 0.000000000000000000, 0.5000000000000000000, 1.000000000000000000 ),
 .UNSPECIFIED. ) ;
#13404=CARTESIAN_POINT ( 'NONE',  ( 17.95841148948556310, 10.23646161652002817, -0.6999999999999784173 ) ) ;
#13406=CARTESIAN_POINT ( 'NONE',  ( -17.93058398061198133, 10.83371123202060993, 0.000000000000000000 ) ) ;
#13419=ORIENTED_EDGE ( 'NONE', *, *, #30813, .F. ) ;
#13439=CARTESIAN_POINT ( 'NONE',  ( -26.79556473285982321, -0.4875557887251183442, -0.6999999999999784173 ) ) ;
#13442=CARTESIAN_POINT ( 'NONE',  ( 17.00199034983389978, -7.902812560182772117, -0.6999999999999783062 ) ) ;
#13443=CARTESIAN_POINT ( 'NONE',  ( -24.36375418918093061, -14.78716628874576244, 6.095965061000018892 ) ) ;
#13447=CARTESIAN_POINT ( 'NONE',  ( -23.47637529058820860, -14.89020704899713365, 5.901296963999991263 ) ) ;
#13449=VERTEX_POINT ( 'NONE', #1179 ) ;
#13459=CARTESIAN_POINT ( 'NONE',  ( -23.78789221090044137, 14.38747862758026663, 5.287321609440595260 ) ) ;
#13472=CARTESIAN_POINT ( 'NONE',  ( -15.86372220156776613, 10.46175468665682118, -0.6999999999999785283 ) ) ;
#13474=CARTESIAN_POINT ( 'NONE',  ( 0.4478609109089253248, -28.49673184309138918, 3.901345920999998995 ) ) ;
#13507=ORIENTED_EDGE ( 'NONE', *, *, #20200, .T. ) ;
#13509=CARTESIAN_POINT ( 'NONE',  ( 17.73794748049035874, 10.04907227125707792, -4.336808689942017243E-16 ) ) ;
#13523=VECTOR ( 'NONE', #23062, 1000.000000000000000 ) ;
#13526=CARTESIAN_POINT ( 'NONE',  ( -19.79264346680938758, 19.51191464210150173, 0.8505138480000007384 ) ) ;
#13527=CARTESIAN_POINT ( 'NONE',  ( 3.940320149735934141, -28.38476056077625742, 8.000000000000007105 ) ) ;
#13547=EDGE_CURVE ( 'NONE', #26737, #17896, #4603, .T. ) ;
#13548=ORIENTED_EDGE ( 'NONE', *, *, #22817, .T. ) ;
#13550=( LENGTH_UNIT ( ) NAMED_UNIT ( * ) SI_UNIT ( .MILLI., .METRE. ) );
#13559=CARTESIAN_POINT ( 'NONE',  ( 23.79192443588063455, -14.38068074323726186, 4.711737058110762710 ) ) ;
#13580=CARTESIAN_POINT ( 'NONE',  ( -23.78820481377726281, 14.38695943193400417, 4.711274593993440618 ) ) ;
#13584=EDGE_LOOP ( 'NONE', ( #21289, #23861, #1160, #4308 ) ) ;
#13598=DIRECTION ( 'NONE',  ( 0.000000000000000000, 0.000000000000000000, -1.000000000000000000 ) ) ;
#13603=CARTESIAN_POINT ( 'NONE',  ( -27.55801272791059731, -0.5014288284350311153, -0.5592437529999827461 ) ) ;
#13608=CARTESIAN_POINT ( 'NONE',  ( 27.71196445724500990, 5.091237891590008502, 0.8585786439999909536 ) ) ;
#13615=CARTESIAN_POINT ( 'NONE',  ( 24.29138541237941240, -13.52003710528471281, 3.901342110999989288 ) ) ;
#13621=CARTESIAN_POINT ( 'NONE',  ( 22.88248055069271203, 14.29577554333692468, -0.6999999999999784173 ) ) ;
#13622=CARTESIAN_POINT ( 'NONE',  ( -23.84668919686734156, 14.28982133724830383, 5.560031205887339567 ) ) ;
#13627=ORIENTED_EDGE ( 'NONE', *, *, #9680, .T. ) ;
#13628=CARTESIAN_POINT ( 'NONE',  ( 24.64102059410889822, -12.87216126329460941, 4.113191254464338975 ) ) ;
#13636=CARTESIAN_POINT ( 'NONE',  ( -3.221827467136498591, -1.415571281914143720, 0.000000000000000000 ) ) ;
#13637=CARTESIAN_POINT ( 'NONE',  ( 0.4831567132674381426, -28.49614615030699838, 3.899998581000013509 ) ) ;
#13638=CARTESIAN_POINT ( 'NONE',  ( -16.14281465707167840, -9.860486966977234147, 0.000000000000000000 ) ) ;
#13642=FACE_BOUND ( 'NONE', #18539, .T. ) ;
#13653=CARTESIAN_POINT ( 'NONE',  ( 26.79556473285982321, 0.4875557887249620803, 0.000000000000000000 ) ) ;
#13654=CARTESIAN_POINT ( 'NONE',  ( 17.93011078763067090, 11.79183908526299085, 0.000000000000000000 ) ) ;
#13673=CARTESIAN_POINT ( 'NONE',  ( -16.85343921402336775, -7.900182044543379689, -0.6999999999999784173 ) ) ;
#13686=CARTESIAN_POINT ( 'NONE',  ( -27.65104932737173371, -3.057638586815402348, 8.000000000000007105 ) ) ;
#13693=B_SPLINE_CURVE_WITH_KNOTS ( 'NONE', 5,
 ( #24017, #15299, #12620, #27104, #7019, #22232 ),
 .UNSPECIFIED., .F., .F.,
 ( 6, 6 ),
 ( -3.500000000000000000, -1.499999893000000029 ),
 .UNSPECIFIED. ) ;
#13709=CARTESIAN_POINT ( 'NONE',  ( -24.06750537087913600, -15.26514226587110379, 4.098700198000015504 ) ) ;
#13710=B_SPLINE_CURVE_WITH_KNOTS ( 'NONE', 3,
 ( #28431, #23575, #16315, #28733, #28588, #16619 ),
 .UNSPECIFIED., .F., .F.,
 ( 4, 2, 4 ),
 ( 0.000000000000000000, 0.5000000000000000000, 1.000000000000000000 ),
 .UNSPECIFIED. ) ;
#13711=CARTESIAN_POINT ( 'NONE',  ( 0.4125558677724673329, -28.49726274111925761, 3.904047916000019658 ) ) ;
#13721=FACE_OUTER_BOUND ( 'NONE', #7282, .T. ) ;
#13724=CARTESIAN_POINT ( 'NONE',  ( 1.533144572080375800, -28.45911136072489001, 5.506490228000010312 ) ) ;
#13730=CARTESIAN_POINT ( 'NONE',  ( -24.41841039498785193, -14.69667350221323865, 6.099998581000020792 ) ) ;
#13731=ORIENTED_EDGE ( 'NONE', *, *, #24858, .T. ) ;
#13757=ORIENTED_EDGE ( 'NONE', *, *, #623, .T. ) ;
#13761=CARTESIAN_POINT ( 'NONE',  ( 26.42504859323178934, 9.566195259927013694, 0.2686740800000309015 ) ) ;
#13777=( LENGTH_UNIT ( ) NAMED_UNIT ( * ) SI_UNIT ( .MILLI., .METRE. ) );
#13784=ORIENTED_EDGE ( 'NONE', *, *, #17077, .F. ) ;
#13791=CARTESIAN_POINT ( 'NONE',  ( -15.73360964030186970, 11.02001161816959396, -0.6999999999999784173 ) ) ;
#13794=CARTESIAN_POINT ( 'NONE',  ( 0.4713258872182368164, -27.79624559782057602, 3.899998581000013509 ) ) ;
#13797=VERTEX_POINT ( 'NONE', #29769 ) ;
#13798=DIRECTION ( 'NONE',  ( -0.000000000000000000, 0.000000000000000000, -1.000000000000000000 ) ) ;
#13819=EDGE_CURVE ( 'NONE', #23829, #25281, #29731, .T. ) ;
#13833=FACE_OUTER_BOUND ( 'NONE', #1637, .T. ) ;
#13843=CARTESIAN_POINT ( 'NONE',  ( 23.81866167241657806, 14.33570040768432996, 3.899998581000013509 ) ) ;
#13845=CARTESIAN_POINT ( 'NONE',  ( -27.73177265635928990, -2.208742311170187378, 8.000000000000007105 ) ) ;
#13847=CARTESIAN_POINT ( 'NONE',  ( 28.40974773466432168, 5.219434544874079762, 1.000000000000000888 ) ) ;
#13849=CARTESIAN_POINT ( 'NONE',  ( -17.93324555120827668, 10.97998838178171432, -1.000005633855494125E-09 ) ) ;
#13855=CARTESIAN_POINT ( 'NONE',  ( -17.69076634382037838, -8.309652824054660769, 0.000000000000000000 ) ) ;
#13868=CARTESIAN_POINT ( 'NONE',  ( 24.16679028237082960, 15.10730797463399000, 3.997250016000014838 ) ) ;
#13871=CARTESIAN_POINT ( 'NONE',  ( -0.6094664100040195764, -28.49364619262437870, 4.999998581000003384 ) ) ;
#13875=DIRECTION ( 'NONE',  ( -0.6941258031311203780, -0.7198537139083029945, 0.000000000000000000 ) ) ;
#13905=CARTESIAN_POINT ( 'NONE',  ( 24.52721838744800920, -14.51532614964689394, 5.760265122000007842 ) ) ;
#13912=CARTESIAN_POINT ( 'NONE',  ( -19.80535397421925481, 19.50875616500616871, 0.9999999989999952543 ) ) ;
#13915=EDGE_CURVE ( 'NONE', #11379, #7420, #22603, .T. ) ;
#13921=B_SPLINE_CURVE_WITH_KNOTS ( 'NONE', 5,
 ( #22741, #3378, #20534, #1660, #8880, #20694, #12983, #13447, #15499, #22596, #15650, #28083, #30292, #18163, #1036 ),
 .UNSPECIFIED., .F., .F.,
 ( 6, 3, 3, 3, 6 ),
 ( 0.000000000000000000, 0.1000000000011452422, 0.3999999999988547161, 0.7000000000011451506, 1.000000000000000000 ),
 .UNSPECIFIED. ) ;
#13930=VERTEX_POINT ( 'NONE', #26424 ) ;
#13943=CARTESIAN_POINT ( 'NONE',  ( 24.82523534259457421, -12.51291187729028742, 4.710542421340364605 ) ) ;
#13946=VERTEX_POINT ( 'NONE', #21700 ) ;
#13952=CARTESIAN_POINT ( 'NONE',  ( -0.5944614571882205212, -27.79380703160649446, 4.999998581000003384 ) ) ;
#13971=CARTESIAN_POINT ( 'NONE',  ( 17.16657240421717390, -9.000000000001264766, -0.6999999999999784173 ) ) ;
#13976=VERTEX_POINT ( 'NONE', #14153 ) ;
#14005=CARTESIAN_POINT ( 'NONE',  ( 28.26943722656857716, 5.193656719585778347, 0.2374258030000131470 ) ) ;
#14012=EDGE_LOOP ( 'NONE', ( #3040, #743, #3091, #26284 ) ) ;
#14015=DIRECTION ( 'NONE',  ( 0.000000000000000000, 0.000000000000000000, 1.000000000000000000 ) ) ;
#14021=VERTEX_POINT ( 'NONE', #11938 ) ;
#14027=( NAMED_UNIT ( * ) PLANE_ANGLE_UNIT ( ) SI_UNIT ( $, .RADIAN. ) );
#14028=CARTESIAN_POINT ( 'NONE',  ( -23.94466870085087606, -15.45669659436210175, 4.319305392000011068 ) ) ;
#14030=CARTESIAN_POINT ( 'NONE',  ( 20.03591075579414849, 19.99999599181853682, 0.2184197934767622973 ) ) ;
#14046=CARTESIAN_POINT ( 'NONE',  ( 1.344125205538966084, -28.46870209102001326, 5.759639119000015128 ) ) ;
#14052=CARTESIAN_POINT ( 'NONE',  ( 17.95841148948556310, 10.23646161652002817, 0.000000000000000000 ) ) ;
#14064=LINE ( 'NONE', #21143, #27716 ) ;
#14072=CARTESIAN_POINT ( 'NONE',  ( -20.14786743110572687, 20.00017459112578067, 0.3952317461953371303 ) ) ;
#14080=CARTESIAN_POINT ( 'NONE',  ( -23.81866442513186755, -14.33570206443695838, 3.899998581000013509 ) ) ;
#14083=EDGE_CURVE ( 'NONE', #29242, #15627, #14687, .T. ) ;
#14097=ORIENTED_EDGE ( 'NONE', *, *, #23384, .F. ) ;
#14103=CARTESIAN_POINT ( 'NONE',  ( -27.71261514784184499, -0.5042418799608706648, 0.5514269430000329208 ) ) ;
#14106=CARTESIAN_POINT ( 'NONE',  ( -23.62421573606080827, -14.65442406347138338, 3.957526371000025023 ) ) ;
#14119=CARTESIAN_POINT ( 'NONE',  ( -24.93720648713954446, 13.79881813474513486, 3.899998581000013509 ) ) ;
#14125=DIRECTION ( 'NONE',  ( 0.6941258031311203780, 0.7198537139083029945, 0.000000000000000000 ) ) ;
#14130=EDGE_CURVE ( 'NONE', #6068, #11650, #12063, .T. ) ;
#14137=ORIENTED_EDGE ( 'NONE', *, *, #25816, .F. ) ;
#14140=CARTESIAN_POINT ( 'NONE',  ( -28.35945636591989683, -7.983396444576476902, 1.000000000000000888 ) ) ;
#14142=CARTESIAN_POINT ( 'NONE',  ( -25.38146355688813216, 12.59839640969179975, 5.200000000000009948 ) ) ;
#14145=CARTESIAN_POINT ( 'NONE',  ( -20.26572724632349320, -21.15151735177849091, 1.000000000000000888 ) ) ;
#14152=CARTESIAN_POINT ( 'NONE',  ( 27.22264131787285990, 6.256663103294479278, 8.000000000000007105 ) ) ;
#14153=CARTESIAN_POINT ( 'NONE',  ( 16.37473331892315542, -8.236461616552139375, 0.000000000000000000 ) ) ;
#14155=CARTESIAN_POINT ( 'NONE',  ( 16.37473331892315542, -8.236461616552139375, -0.6999999999999784173 ) ) ;
#14157=CARTESIAN_POINT ( 'NONE',  ( 28.49528339128749366, 0.5184828350247226991, 1.000000000000000888 ) ) ;
#14160=CARTESIAN_POINT ( 'NONE',  ( -24.86822223968197321, -13.92223202027371975, 5.680679499000030219 ) ) ;
#14163=B_SPLINE_CURVE_WITH_KNOTS ( 'NONE', 5,
 ( #29743, #29433, #24878, #15569, #27684, #25027 ),
 .UNSPECIFIED., .F., .F.,
 ( 6, 6 ),
 ( 0.000000000000000000, 1.000000000000000000 ),
 .UNSPECIFIED. ) ;
#14165=CARTESIAN_POINT ( 'NONE',  ( -15.73094807329767519, -9.126265404193597774, -0.6999999999999784173 ) ) ;
#14178=CARTESIAN_POINT ( 'NONE',  ( 23.80092420482279891, 14.36517094565843777, 3.899998581000013509 ) ) ;
#14179=CARTESIAN_POINT ( 'NONE',  ( -24.41841039498785193, -14.69667350221323865, 3.899998581000013509 ) ) ;
#14190=CARTESIAN_POINT ( 'NONE',  ( 3.547887315624699056, -0.01749626818330200437, 0.000000000000000000 ) ) ;
#14192=CARTESIAN_POINT ( 'NONE',  ( 24.97472003062369694, 13.73006752330286595, 5.208359080000030339 ) ) ;
#14193=CARTESIAN_POINT ( 'NONE',  ( -25.33388805469397198, 13.05639290202442204, 5.735287127840217991 ) ) ;
#14203=DIRECTION ( 'NONE',  ( 0.8687154346624373913, 0.4953115116563036602, 0.000000000000000000 ) ) ;
#14229=ORIENTED_EDGE ( 'NONE', *, *, #17750, .F. ) ;
#14231=CARTESIAN_POINT ( 'NONE',  ( 1.607747500013188446, -28.45491842328731025, 4.689797669000017599 ) ) ;
#14234=FACE_OUTER_BOUND ( 'NONE', #21310, .T. ) ;
#14237=DIRECTION ( 'NONE',  ( -0.6941258031311203780, -0.7198537139083029945, 0.000000000000000000 ) ) ;
#14241=CARTESIAN_POINT ( 'NONE',  ( -16.99800965038351919, -7.902812560281212484, -0.6999999999999783062 ) ) ;
#14242=CARTESIAN_POINT ( 'NONE',  ( -26.79556473285982321, -0.4875557887250189237, 0.000000000000000000 ) ) ;
#14255=CARTESIAN_POINT ( 'NONE',  ( 1.605176535610508326, -27.75389821387976852, 4.999998581000003384 ) ) ;
#14268=CARTESIAN_POINT ( 'NONE',  ( 24.32472724076343695, -13.45989056521276872, 3.899998581000013509 ) ) ;
#14278=CARTESIAN_POINT ( 'NONE',  ( -25.44662322720032677, 12.83524168051548564, 4.689351480999998323 ) ) ;
#14281=B_SPLINE_SURFACE_WITH_KNOTS ( 'NONE', 5, 1, ( 
 ( #4828, #7339 ),
 ( #5287, #269 ),
 ( #16924, #12512 ),
 ( #29346, #581 ),
 ( #26993, #10162 ),
 ( #15042, #14425 ),
 ( #26532, #9850 ),
 ( #26681, #19606 ),
 ( #1183, #3223 ),
 ( #3373, #17842 ),
 ( #3853, #27763 ),
 ( #13443, #8558 ),
 ( #10322, #8242 ),
 ( #10475, #6207 ),
 ( #15184, #15344 ) ),
 .UNSPECIFIED., .F., .F., .F.,
 ( 6, 3, 3, 3, 6 ),
 ( 2, 2 ),
 ( 0.000000000000000000, 0.5238999881920000101, 1.047799976390000110, 1.571699964580000053, 1.746333293980000034 ),
 ( -0.7000000000009999335, 2.555864960449999711E-06 ),
 .UNSPECIFIED. ) ;
#14283=CARTESIAN_POINT ( 'NONE',  ( -16.85343921422224156, -7.900182044607009679, 0.000000000000000000 ) ) ;
#14284=CARTESIAN_POINT ( 'NONE',  ( 24.97472003062369694, 13.73006752330286595, 5.208359080000030339 ) ) ;
#14298=B_SPLINE_CURVE_WITH_KNOTS ( 'NONE', 5,
 ( #19278, #7322, #19432, #24306, #16907, #29023, #28869, #12349, #2140, #26058, #11729, #18964, #7011, #4644, #14255 ),
 .UNSPECIFIED., .F., .F.,
 ( 6, 3, 3, 3, 6 ),
 ( -1.746338520749999956, -1.571704668670000027, -1.047803112450000018, -0.5239015562239999202, 0.000000000000000000 ),
 .UNSPECIFIED. ) ;
#14300=CARTESIAN_POINT ( 'NONE',  ( -27.79539923781684507, -0.5057481689249112566, 1.000000000000000888 ) ) ;
#14316=B_SPLINE_CURVE_WITH_KNOTS ( 'NONE', 3,
 ( #13730, #10741, #22705, #25068, #25387, #11214, #6488, #25223, #10906, #1783, #20970, #20341 ),
 .UNSPECIFIED., .F., .F.,
 ( 4, 2, 2, 2, 2, 4 ),
 ( 0.000000000000000000, 0.2499999999999992784, 0.4999999999999985567, 0.6249999999999991118, 0.7499999999999995559, 1.000000000000000000 ),
 .UNSPECIFIED. ) ;
#14321=CARTESIAN_POINT ( 'NONE',  ( -18.22442895416311970, 20.00000017544967079, -0.6880553899999974909 ) ) ;
#14348=CARTESIAN_POINT ( 'NONE',  ( 17.16657240419154462, 10.99999999996915179, -0.6999999999999784173 ) ) ;
#14349=CARTESIAN_POINT ( 'NONE',  ( 17.47393819615788502, -10.06595463928881884, -4.336808689942018722E-16 ) ) ;
#14355=EDGE_CURVE ( 'NONE', #9797, #25869, #7921, .T. ) ;
#14359=CARTESIAN_POINT ( 'NONE',  ( 19.80526555972147307, 19.50877392102524155, 0.9999999989999952543 ) ) ;
#14363=CARTESIAN_POINT ( 'NONE',  ( 1.186786632855649781, -28.47586096820935353, 5.900907654000003610 ) ) ;
#14365=ORIENTED_EDGE ( 'NONE', *, *, #26192, .F. ) ;
#14367=CARTESIAN_POINT ( 'NONE',  ( 17.14656078599760392, 12.09981795542235439, -1.000005633855494125E-09 ) ) ;
#14371=ORIENTED_EDGE ( 'NONE', *, *, #21478, .F. ) ;
#14375=ORIENTED_EDGE ( 'NONE', *, *, #12099, .T. ) ;
#14382=CARTESIAN_POINT ( 'NONE',  ( 17.99591112602217891, 19.96082062028142090, 0.000000000000000000 ) ) ;
#14385=CARTESIAN_POINT ( 'NONE',  ( -19.42687617620407892, 20.00000591289990481, -0.3112909302383543575 ) ) ;
#14390=VERTEX_POINT ( 'NONE', #27805 ) ;
#14400=CARTESIAN_POINT ( 'NONE',  ( -17.13980697812163712, -7.934232311348328182, -0.6999999999999785283 ) ) ;
#14406=SURFACE_STYLE_FILL_AREA ( #9522 ) ;
#14408=CARTESIAN_POINT ( 'NONE',  ( 23.81776757408896472, 15.65134803726520296, 5.147520328545557078 ) ) ;
#14416=CARTESIAN_POINT ( 'NONE',  ( -23.98258507372315051, -15.39789217239198571, 4.239862999000004962 ) ) ;
#14425=CARTESIAN_POINT ( 'NONE',  ( -23.35655559443967988, -15.07705663931308671, 5.680691770000024121 ) ) ;
#14431=CARTESIAN_POINT ( 'NONE',  ( -24.35797963555383205, 13.39969403207715892, 3.901342130000013064 ) ) ;
#14436=CARTESIAN_POINT ( 'NONE',  ( 24.98081130624543889, 13.71897605842228529, 4.999998581000003384 ) ) ;
#14439=VERTEX_POINT ( 'NONE', #4666 ) ;
#14453=CARTESIAN_POINT ( 'NONE',  ( -27.87609112763790975, 3.928995115430390150, 3.799999999999998046 ) ) ;
#14457=FACE_BOUND ( 'NONE', #3007, .T. ) ;
#14465=CARTESIAN_POINT ( 'NONE',  ( 26.79556473285982321, 0.4875557887249620803, 0.000000000000000000 ) ) ;
#14473=CARTESIAN_POINT ( 'NONE',  ( -16.06988921231594603, 11.79183908526949054, 0.000000000000000000 ) ) ;
#14474=CARTESIAN_POINT ( 'NONE',  ( -24.66346748865669625, -14.28208995890502564, 6.002748559000014694 ) ) ;
#14481=ORIENTED_EDGE ( 'NONE', *, *, #25585, .T. ) ;
#14488=B_SPLINE_CURVE_WITH_KNOTS ( 'NONE', 3,
 ( #3662, #16665, #10, #28634, #14165, #21560 ),
 .UNSPECIFIED., .F., .F.,
 ( 4, 2, 4 ),
 ( 0.000000000000000000, 0.5000000000000000000, 1.000000000000000000 ),
 .UNSPECIFIED. ) ;
#14495=CARTESIAN_POINT ( 'NONE',  ( 21.28666574344908469, 18.00484885041732142, 1.000000000000000888 ) ) ;
#14498=CARTESIAN_POINT ( 'NONE',  ( -24.37821945910799926, 14.76389285725497125, 5.208432825000025801 ) ) ;
#14500=DIRECTION ( 'NONE',  ( 0.000000000000000000, 0.000000000000000000, -1.000000000000000000 ) ) ;
#14504=CARTESIAN_POINT ( 'NONE',  ( 1.074123786107241241, -3.361570641823106165, 0.000000000000000000 ) ) ;
#14507=CARTESIAN_POINT ( 'NONE',  ( 24.00926693399461342, 14.01467022386263395, 6.042472827000016977 ) ) ;
#14531=CARTESIAN_POINT ( 'NONE',  ( -24.98081131316241255, -13.71897606304888662, 4.999998581000003384 ) ) ;
#14541=B_SPLINE_SURFACE_WITH_KNOTS ( 'NONE', 5, 1, ( 
 ( #6243, #12694 ),
 ( #10811, #22929 ),
 ( #20560, #8117 ),
 ( #5614, #6077 ),
 ( #29991, #15674 ),
 ( #12859, #22461 ),
 ( #30155, #15846 ),
 ( #3404, #22306 ),
 ( #24820, #25450 ) ),
 .UNSPECIFIED., .F., .F., .F.,
 ( 6, 3, 6 ),
 ( 2, 2 ),
 ( 0.000000000000000000, 12.04044600379999963, 17.39568165169999858 ),
 ( -4.097259680450000872E-15, 0.7017616274569999923 ),
 .UNSPECIFIED. ) ;
#14546=CARTESIAN_POINT ( 'NONE',  ( 17.95841148948556310, 10.23646161652002817, -0.6999999999999784173 ) ) ;
#14572=B_SPLINE_SURFACE_WITH_KNOTS ( 'NONE', 5, 1, ( 
 ( #24481, #7938 ),
 ( #12511, #9849 ),
 ( #19448, #7787 ),
 ( #17539, #17389 ),
 ( #15183, #24787 ),
 ( #3220, #12831 ),
 ( #22433, #29039 ),
 ( #23059, #25422 ),
 ( #20215, #8557 ),
 ( #15811, #17841 ),
 ( #11094, #15645 ),
 ( #5887, #25098 ),
 ( #23212, #5738 ),
 ( #24941, #20071 ),
 ( #12977, #3372 ) ),
 .UNSPECIFIED., .F., .F., .F.,
 ( 6, 3, 3, 3, 6 ),
 ( 2, 2 ),
 ( 0.000000000000000000, 0.5239010160280000994, 1.047802032050000109, 1.571703048080000054, 1.746336720089999961 ),
 ( -0.7000000000009999335, 2.556023394720000151E-06 ),
 .UNSPECIFIED. ) ;
#14581=CARTESIAN_POINT ( 'NONE',  ( 22.41261198964086176, 16.47772013495439225, 7.000000000000006217 ) ) ;
#14591=CARTESIAN_POINT ( 'NONE',  ( -24.83827471527357744, 12.48687850854618198, 4.895780543000022078 ) ) ;
#14593=EDGE_CURVE ( 'NONE', #6349, #6970, #36, .T. ) ;
#14596=CARTESIAN_POINT ( 'NONE',  ( 18.13627779908860305, 10.46175468807264863, -0.6999999999999785283 ) ) ;
#14598=CARTESIAN_POINT ( 'NONE',  ( 19.80526555972147307, 19.50877392102524155, 1.400000000000012346 ) ) ;
#14600=ORIENTED_EDGE ( 'NONE', *, *, #3677, .F. ) ;
#14604=VERTEX_POINT ( 'NONE', #5743 ) ;
#14608=ORIENTED_EDGE ( 'NONE', *, *, #27578, .F. ) ;
#14617=CARTESIAN_POINT ( 'NONE',  ( 24.86822223037987456, 13.92223202030449691, 4.319317656000021266 ) ) ;
#14626=CARTESIAN_POINT ( 'NONE',  ( -15.73622915490642526, 11.16397745117368245, -4.336808689942018722E-16 ) ) ;
#14646=CYLINDRICAL_SURFACE ( 'NONE', #6516, 1.100000000000002309 ) ;
#14651=CARTESIAN_POINT ( 'NONE',  ( 18.52668879010899516, 20.00003523974170605, -0.6360013681344631742 ) ) ;
#14652=CARTESIAN_POINT ( 'NONE',  ( -24.37165444408190851, 14.77472139917419369, 5.104215870000011535 ) ) ;
#14675=CARTESIAN_POINT ( 'NONE',  ( -16.52704821190178208, 9.934232311991996411, -0.6999999999999785283 ) ) ;
#14678=ORIENTED_EDGE ( 'NONE', *, *, #6579, .F. ) ;
#14687=B_SPLINE_CURVE_WITH_KNOTS ( 'NONE', 3,
 ( #17273, #12704, #27185, #15076, #10203, #24830 ),
 .UNSPECIFIED., .F., .F.,
 ( 4, 2, 4 ),
 ( 0.000000000000000000, 0.5000000000000000000, 1.000000000000000000 ),
 .UNSPECIFIED. ) ;
#14688=CARTESIAN_POINT ( 'NONE',  ( 18.15349680648220954, 19.92137135063213549, 0.007031429000020628095 ) ) ;
#14700=EDGE_CURVE ( 'NONE', #13976, #19663, #15818, .T. ) ;
#14711=B_SPLINE_CURVE_WITH_KNOTS ( 'NONE', 5,
 ( #3760, #29411, #29875, #27210, #8002, #7847, #5649, #14140, #6736 ),
 .UNSPECIFIED., .F., .F.,
 ( 6, 3, 6 ),
 ( 0.000000000000000000, 55.31395627320000585, 94.75474476520000167 ),
 .UNSPECIFIED. ) ;
#14724=UNCERTAINTY_MEASURE_WITH_UNIT (LENGTH_MEASURE( 1.000000000000000082E-05 ), #13777, 'distance_accuracy_value', 'NONE');
#14735=CARTESIAN_POINT ( 'NONE',  ( -27.90496282365170799, -7.855453155277750454, -0.2432540810000105580 ) ) ;
#14738=CARTESIAN_POINT ( 'NONE',  ( -25.77914833267782413, -15.40383343775964065, 8.000000000000007105 ) ) ;
#14757=CARTESIAN_POINT ( 'NONE',  ( -23.77307140041805411, 14.41181874028064591, 4.895781291000017355 ) ) ;
#14758=CARTESIAN_POINT ( 'NONE',  ( -27.07233446881474137, 8.380004974202883261, 2.400000000000013234 ) ) ;
#14763=CARTESIAN_POINT ( 'NONE',  ( 23.47715715144835613, -20.00370206646645599, 8.000000000000007105 ) ) ;
#14792=VERTEX_POINT ( 'NONE', #16583 ) ;
#14802=CARTESIAN_POINT ( 'NONE',  ( -23.77307140041805411, 14.41181874028064591, 4.999998581000003384 ) ) ;
#14814=CARTESIAN_POINT ( 'NONE',  ( 24.43659368183839931, 14.66646236428692340, 6.099998581000020792 ) ) ;
#14817=ADVANCED_FACE ( 'NONE', ( #14234 ), #4627, .F. ) ;
#14820=CARTESIAN_POINT ( 'NONE',  ( -24.14840830027331364, -13.77363891130890039, 4.098702617000016701 ) ) ;
#14825=EDGE_CURVE ( 'NONE', #17991, #1011, #7157, .T. ) ;
#14826=DIRECTION ( 'NONE',  ( 0.000000000000000000, 0.000000000000000000, -1.000000000000000000 ) ) ;
#14829=B_SPLINE_SURFACE_WITH_KNOTS ( 'NONE', 5, 5, ( 
 ( #27838, #30680, #8634, #1731, #28307, #23608, #23137, #11167, #8798 ),
 ( #28157, #18708, #2044, #18230, #11634, #27997, #21233, #30832, #28465 ),
 ( #18868, #6902, #16505, #4978, #5588, #26842, #22439, #2617, #24793 ),
 ( #7945, #20076, #19767, #21978, #12209, #29352, #884, #17688, #29508 ),
 ( #22278, #24333, #275, #24487, #5745, #17544, #26998, #21821, #586 ),
 ( #15348, #26686, #9856, #12671, #7640, #19454, #15189, #29046, #5125 ),
 ( #3229, #24640, #2926, #19611, #29192, #27155, #17395, #7492, #17086 ),
 ( #10480, #5292, #12368, #3073, #14735, #15048, #2777, #434, #12836 ),
 ( #7795, #5438, #736, #10014, #14895, #29666, #10327, #17237, #8096 ) ),
 .UNSPECIFIED., .F., .F., .F.,
 ( 6, 3, 6 ),
 ( 6, 3, 6 ),
 ( 0.000000000000000000, 54.03331039209999886, 92.56095350929999199 ),
 ( 8.011061266649999624, 9.405960541640000727, 10.80085981660000094 ),
 .UNSPECIFIED. ) ;
#14845=CARTESIAN_POINT ( 'NONE',  ( -25.32653162617393861, 13.07087917251410403, 5.760266710000017554 ) ) ;
#14858=CARTESIAN_POINT ( 'NONE',  ( -24.64320960688972306, 12.86800382723239622, 4.117082646578299254 ) ) ;
#14867=CARTESIAN_POINT ( 'NONE',  ( -24.71034964618677776, 13.49086583186187660, 0.2686791940000321510 ) ) ;
#14872=( NAMED_UNIT ( * ) SI_UNIT ( $, .STERADIAN. ) SOLID_ANGLE_UNIT ( ) );
#14875=ADVANCED_FACE ( 'NONE', ( #31068 ), #24141, .F. ) ;
#14881=B_SPLINE_CURVE_WITH_KNOTS ( 'NONE', 3,
 ( #9678, #17981, #865, #15631, #3514, #27592, #13112, #20053, #20516, #24931, #5725, #10922 ),
 .UNSPECIFIED., .F., .F.,
 ( 4, 2, 2, 2, 2, 4 ),
 ( 0.000000000000000000, 0.2499999999999997224, 0.4999999999999996669, 0.6249999999999997780, 0.7499999999999997780, 1.000000000000000000 ),
 .UNSPECIFIED. ) ;
#14895=CARTESIAN_POINT ( 'NONE',  ( -28.03861306157277866, -0.5101735396242147447, -0.2432540810000105580 ) ) ;
#14914=CARTESIAN_POINT ( 'NONE',  ( -24.81746041937532965, 14.01353061208509310, 3.920132063000014710 ) ) ;
#14915=CARTESIAN_POINT ( 'NONE',  ( -19.80535357367646654, 19.50875577052770993, 2.400000000000013234 ) ) ;
#14918=FACE_OUTER_BOUND ( 'NONE', #20351, .T. ) ;
#14920=DIRECTION ( 'NONE',  ( 0.000000000000000000, 0.000000000000000000, -1.000000000000000000 ) ) ;
#14923=CARTESIAN_POINT ( 'NONE',  ( 24.61381495443087175, 14.36755986787189521, 3.957524335000017768 ) ) ;
#14939=CARTESIAN_POINT ( 'NONE',  ( 25.45799949673341800, -12.81261086040661645, 4.791562841999996714 ) ) ;
#14952=CARTESIAN_POINT ( 'NONE',  ( 27.51770821245201759, 4.728187301810311105, 8.000000000000007105 ) ) ;
#14962=CARTESIAN_POINT ( 'NONE',  ( 24.27467683999808301, -13.55001166052597128, 6.095967889000020179 ) ) ;
#14964=CARTESIAN_POINT ( 'NONE',  ( 24.31416967338466861, 13.47842985269137728, 5.506973475999988210 ) ) ;
#14980=CARTESIAN_POINT ( 'NONE',  ( 25.41371745730516807, 13.31556240574341210, 8.000000000000007105 ) ) ;
#14992=CARTESIAN_POINT ( 'NONE',  ( -24.73569401515663202, 12.68911708161206953, 5.680831397999991594 ) ) ;
#14993=CARTESIAN_POINT ( 'NONE',  ( 20.77600629922060449, 21.68409807857484140, 1.000000000000000888 ) ) ;
#15015=CARTESIAN_POINT ( 'NONE',  ( -24.95150188576461403, 13.62250486174595920, 0.8585803919999857037 ) ) ;
#15022=DIRECTION ( 'NONE',  ( 0.000000000000000000, 0.000000000000000000, -1.000000000000000000 ) ) ;
#15033=ORIENTED_EDGE ( 'NONE', *, *, #8063, .T. ) ;
#15042=CARTESIAN_POINT ( 'NONE',  ( -23.94466870085087606, -15.45669659436210175, 5.680691770000024121 ) ) ;
#15048=CARTESIAN_POINT ( 'NONE',  ( -28.21939423762516341, -7.943967920865026677, 0.2374258030000131470 ) ) ;
#15053=CARTESIAN_POINT ( 'NONE',  ( 0.4368970292312223669, -27.79681690464256150, 6.098651241000007772 ) ) ;
#15054=ORIENTED_EDGE ( 'NONE', *, *, #353, .F. ) ;
#15061=CARTESIAN_POINT ( 'NONE',  ( 27.42619050773425826, -9.513793714290953218, 0.08279779300002232389 ) ) ;
#15063=EDGE_LOOP ( 'NONE', ( #11375, #9214, #15702, #1283 ) ) ;
#15073=CARTESIAN_POINT ( 'NONE',  ( -24.66346748855670867, -14.28208995890320665, 3.997248602000014195 ) ) ;
#15076=CARTESIAN_POINT ( 'NONE',  ( -16.26205251953807007, 10.04907227120676261, -4.336808689942017243E-16 ) ) ;
#15077=ADVANCED_FACE ( 'NONE', ( #16070 ), #2225, .F. ) ;
#15087=EDGE_CURVE ( 'NONE', #15510, #1011, #26691, .T. ) ;
#15088=CARTESIAN_POINT ( 'NONE',  ( -16.81341597763548990, -10.09981795544978311, -0.6999999999999784173 ) ) ;
#15110=CARTESIAN_POINT ( 'NONE',  ( -16.06988921239048551, -8.208160914692745891, -0.6999999999999784173 ) ) ;
#15113=CARTESIAN_POINT ( 'NONE',  ( 24.74993095452947856, -14.13250376044891965, 6.042507811999997536 ) ) ;
#15114=CARTESIAN_POINT ( 'NONE',  ( 18.80717682333433061, 19.99999822827082241, -0.5856167109999921294 ) ) ;
#15115=CARTESIAN_POINT ( 'NONE',  ( 28.68577476838161644, -9.950727360109466346, 8.000000000000007105 ) ) ;
#15116=CARTESIAN_POINT ( 'NONE',  ( 28.53960566377543984, -1.916108254339756067, 8.000000000000007105 ) ) ;
#15134=CARTESIAN_POINT ( 'NONE',  ( -16.70716219638308075, 12.10247952391986281, -0.6999999999999784173 ) ) ;
#15136=CARTESIAN_POINT ( 'NONE',  ( 16.19686700681432256, -8.461754693832318708, -0.6999999999999785283 ) ) ;
#15139=CARTESIAN_POINT ( 'NONE',  ( 0.4831567132655384955, -28.49614615030703391, 6.099998581000020792 ) ) ;
#15152=CARTESIAN_POINT ( 'NONE',  ( -3.254826447623020425, 1.366018022090351280, -0.6999999999999783062 ) ) ;
#15158=CARTESIAN_POINT ( 'NONE',  ( -22.06913545123989806, 17.56725181269473524, 0.8585790010000038386 ) ) ;
#15162=ORIENTED_EDGE ( 'NONE', *, *, #24774, .T. ) ;
#15171=CARTESIAN_POINT ( 'NONE',  ( -28.35455043824866550, -0.5159221438580332553, 0.2374258030000131470 ) ) ;
#15182=CARTESIAN_POINT ( 'NONE',  ( -15.73099012567143618, 10.87604578374266673, -1.384526174263989162E-13 ) ) ;
#15183=CARTESIAN_POINT ( 'NONE',  ( -24.92639508767336309, -13.81781708088548122, 5.506973469000003618 ) ) ;
#15184=CARTESIAN_POINT ( 'NONE',  ( -24.41841039498785193, -14.69667350221323865, 6.099998581000020792 ) ) ;
#15189=CARTESIAN_POINT ( 'NONE',  ( -20.74517834863038601, -21.65192390581155379, 0.5017677510000262409 ) ) ;
#15194=ADVANCED_FACE ( 'NONE', ( #24 ), #19205, .F. ) ;
#15196=CARTESIAN_POINT ( 'NONE',  ( 0.4713258872163371693, -27.79624559782060800, 6.099998581000020792 ) ) ;
#15205=ORIENTED_EDGE ( 'NONE', *, *, #17928, .F. ) ;
#15207=CARTESIAN_POINT ( 'NONE',  ( 22.75205003212621335, -19.38592737840143343, 0.000000000000000000 ) ) ;
#15212=CARTESIAN_POINT ( 'NONE',  ( 25.05552768372066907, -13.58331698798256504, 3.920132093000017193 ) ) ;
#15216=CARTESIAN_POINT ( 'NONE',  ( 24.97129468909112404, -13.73710443560444183, 6.098655031999994591 ) ) ;
#15217=DIRECTION ( 'NONE',  ( -0.6941258031311203780, -0.7198537139083029945, 0.000000000000000000 ) ) ;
#15220=CARTESIAN_POINT ( 'NONE',  ( 16.06675444873834380, 10.97998838177521286, -0.6999999999999784173 ) ) ;
#15233=CARTESIAN_POINT ( 'NONE',  ( -17.59696597926837214, -9.791839085300418688, -0.6999999999999784173 ) ) ;
#15239=ORIENTED_EDGE ( 'NONE', *, *, #7753, .T. ) ;
#15257=CARTESIAN_POINT ( 'NONE',  ( -22.41290914069411500, 16.47772183393138690, 7.000000021000013284 ) ) ;
#15262=DIRECTION ( 'NONE',  ( 0.000000000000000000, 0.000000000000000000, -1.000000000000000000 ) ) ;
#15280=ORIENTED_EDGE ( 'NONE', *, *, #11250, .F. ) ;
#15289=CARTESIAN_POINT ( 'NONE',  ( -24.83827471527357744, 12.48687850854618198, 4.999998581000003384 ) ) ;
#15291=ORIENTED_EDGE ( 'NONE', *, *, #1666, .T. ) ;
#15292=DIRECTION ( 'NONE',  ( 0.000000000000000000, 0.000000000000000000, -1.000000000000000000 ) ) ;
#15297=ADVANCED_FACE ( 'NONE', ( #28790, #26748 ), #17159, .T. ) ;
#15299=CARTESIAN_POINT ( 'NONE',  ( -19.80535357367646654, 19.50875577052770993, 1.400000021000019634 ) ) ;
#15310=CARTESIAN_POINT ( 'NONE',  ( 2.507604248379858625, 2.484315071469196390, -0.6999999999999784173 ) ) ;
#15319=CARTESIAN_POINT ( 'NONE',  ( -26.10391306214228990, 8.822478663265938437, 0.000000000000000000 ) ) ;
#15323=EDGE_LOOP ( 'NONE', ( #26131, #25728, #3247, #28173 ) ) ;
#15329=CARTESIAN_POINT ( 'NONE',  ( 23.25311087529421172, 15.23597699658644800, 5.310552110000033466 ) ) ;
#15334=CARTESIAN_POINT ( 'NONE',  ( -24.93720648713954446, 13.79881813474513486, 3.899998581000013509 ) ) ;
#15344=CARTESIAN_POINT ( 'NONE',  ( -23.81866173682177390, -14.33570044646243247, 6.099998581000020792 ) ) ;
#15348=CARTESIAN_POINT ( 'NONE',  ( -19.53673505992006554, -20.39066108913833020, -0.6999999999999784173 ) ) ;
#15356=CARTESIAN_POINT ( 'NONE',  ( -0.4969045691271392617, -28.49594262166942116, 5.506468674000009500 ) ) ;
#15357=B_SPLINE_CURVE_WITH_KNOTS ( 'NONE', 1,
 ( #21869, #28771 ),
 .UNSPECIFIED., .F., .F.,
 ( 2, 2 ),
 ( -2.556017480449999863E-06, 0.7000000000009999335 ),
 .UNSPECIFIED. ) ;
#15365=ORIENTED_EDGE ( 'NONE', *, *, #1804, .T. ) ;
#15375=EDGE_LOOP ( 'NONE', ( #16869, #11049, #22062, #15733 ) ) ;
#15377=CARTESIAN_POINT ( 'NONE',  ( 27.79539923781684507, 0.5057481689249235801, 8.000000000000007105 ) ) ;
#15383=B_SPLINE_CURVE_WITH_KNOTS ( 'NONE', 3,
 ( #4617, #28069, #18936, #30908, #6985, #14072, #6514, #21462, #23676, #30600, #9495, #4318, #16264, #28692, #16720, #28538, #23526, #16113, #26339, #23370, #14385, #20997, #18626, #28223, #1960, #6666, #2423, #28387, #21306, #11553, #30747, #9176, #11704, #18778, #3444, #26487, #24867, #24133, #16884, #69, #12899, #20284, #9650, #9811 ),
 .UNSPECIFIED., .F., .F.,
 ( 4, 2, 2, 1, 1, 2, 2, 2, 2, 1, 1, 1, 2, 2, 2, 2, 1, 1, 1, 2, 2, 2, 2, 2, 2, 4 ),
 ( 0.000000000000000000, 0.1249999999999620304, 0.1874999999999430456, 0.2187499999999342470, 0.2343749999999298617, 0.2421874999999276412, 0.2499999999999254485, 0.3749999999998888667, 0.4374999999998705480, 0.4687499999998613887, 0.4843749999998567812, 0.4921874999998557265, 0.4960937499998562816, 0.4999999999998568923, 0.6249999999998990807, 0.6874999999999187317, 0.7187499999999298339, 0.7343749999999368283, 0.7421874999999389377, 0.7460937499999413802, 0.7499999999999437117, 0.8124999999999601430, 0.8437499999999666933, 0.8593749999999701350, 0.8749999999999734657, 1.000000000000000000 ),
 .UNSPECIFIED. ) ;
#15384=CARTESIAN_POINT ( 'NONE',  ( -3.040504020835836041, -1.733590291693717145, -0.6999999999999784173 ) ) ;
#15390=CARTESIAN_POINT ( 'NONE',  ( -17.62526668112344908, -8.236461616547455122, -0.6999999999999784173 ) ) ;
#15399=ORIENTED_EDGE ( 'NONE', *, *, #14355, .T. ) ;
#15402=CARTESIAN_POINT ( 'NONE',  ( 24.31416967338466861, 13.47842985269137728, 4.493023686000019445 ) ) ;
#15403=CARTESIAN_POINT ( 'NONE',  ( 17.47393819644387136, 9.934045360783191114, -4.336808689942018722E-16 ) ) ;
#15417=CARTESIAN_POINT ( 'NONE',  ( -4.785279987089964493, -31.71089578132167119, 1.000000000000000888 ) ) ;
#15418=CARTESIAN_POINT ( 'NONE',  ( 18.26639035967037827, -8.979988381807324060, -0.6999999999999784173 ) ) ;
#15420=CARTESIAN_POINT ( 'NONE',  ( 21.32490733757747137, 17.21310361452476201, -0.6999999999999784173 ) ) ;
#15422=CARTESIAN_POINT ( 'NONE',  ( 27.79539923781684507, 0.5057481689249130330, 1.000000000000000888 ) ) ;
#15423=EDGE_CURVE ( 'NONE', #7575, #2099, #28562, .T. ) ;
#15441=CARTESIAN_POINT ( 'NONE',  ( -16.95738181089354057, 9.897562529807188980, -0.6999999999999783062 ) ) ;
#15442=CARTESIAN_POINT ( 'NONE',  ( -17.89938223499811087, -9.307365792571914653, -0.6999999999999784173 ) ) ;
#15446=CARTESIAN_POINT ( 'NONE',  ( -24.31107512894012146, -13.48383474011653860, 5.495825983432886197 ) ) ;
#15453=CARTESIAN_POINT ( 'NONE',  ( -17.72558663041863269, -8.340546693701178071, -0.6999999999999783062 ) ) ;
#15467=EDGE_LOOP ( 'NONE', ( #4220, #4446, #20851, #2039 ) ) ;
#15469=CARTESIAN_POINT ( 'NONE',  ( -19.53673505992006554, -20.39066108913833020, -0.6999999999999784173 ) ) ;
#15472=EDGE_CURVE ( 'NONE', #18728, #3218, #15383, .T. ) ;
#15490=CARTESIAN_POINT ( 'NONE',  ( 24.88589369718092215, -13.89120818692358483, 3.904029272000009154 ) ) ;
#15496=CARTESIAN_POINT ( 'NONE',  ( 21.92393651391584086, 17.69663393520839989, 0.9999999989999952543 ) ) ;
#15499=CARTESIAN_POINT ( 'NONE',  ( -23.39354070939840824, -15.01969650306709170, 5.760134161999996394 ) ) ;
#15510=VERTEX_POINT ( 'NONE', #21619 ) ;
#15514=CARTESIAN_POINT ( 'NONE',  ( -4.663556906300703631, -30.90433882808243027, 0.7069209039999857502 ) ) ;
#15518=CARTESIAN_POINT ( 'NONE',  ( 24.98823331316959440, -13.70626928515100573, 3.904029301000005781 ) ) ;
#15519=CARTESIAN_POINT ( 'NONE',  ( 23.23277120357798964, 15.26692725135965745, 4.999998581000003384 ) ) ;
#15540=VERTEX_POINT ( 'NONE', #15110 ) ;
#15543=ADVANCED_FACE ( 'NONE', ( #26642 ), #12391, .F. ) ;
#15550=CARTESIAN_POINT ( 'NONE',  ( 23.81866173088643635, 14.33570044285385947, 3.899998581000013509 ) ) ;
#15563=CARTESIAN_POINT ( 'NONE',  ( 18.62349342026574917, 19.80369317695730302, 0.06728435000000199118 ) ) ;
#15569=CARTESIAN_POINT ( 'NONE',  ( 21.70992212615148986, 18.50697891487987334, 5.000000000000004441 ) ) ;
#15575=CARTESIAN_POINT ( 'NONE',  ( 23.98258507289250474, 15.39789216307533160, 5.760134169000008519 ) ) ;
#15583=ORIENTED_EDGE ( 'NONE', *, *, #2023, .T. ) ;
#15593=CARTESIAN_POINT ( 'NONE',  ( -24.83828730555975284, 12.48688483815296735, 5.104216618000034345 ) ) ;
#15595=B_SPLINE_CURVE_WITH_KNOTS ( 'NONE', 3,
 ( #14367, #9628, #2703, #21914, #9789, #198 ),
 .UNSPECIFIED., .F., .F.,
 ( 4, 2, 4 ),
 ( 0.000000000000000000, 0.5000000000000000000, 1.000000000000000000 ),
 .UNSPECIFIED. ) ;
#15596=CARTESIAN_POINT ( 'NONE',  ( -0.3775595308767857317, -28.49777658967402871, 4.319846982000025370 ) ) ;
#15600=CARTESIAN_POINT ( 'NONE',  ( 24.18685237987300951, -13.70673315802992676, 3.927097088518238799 ) ) ;
#15601=ORIENTED_EDGE ( 'NONE', *, *, #4892, .T. ) ;
#15627=VERTEX_POINT ( 'NONE', #8315 ) ;
#15631=CARTESIAN_POINT ( 'NONE',  ( 1.079837148504761979, -28.48011631689465517, 5.965513408196154721 ) ) ;
#15633=CARTESIAN_POINT ( 'NONE',  ( -28.03861306157277866, -0.5101735396241460219, -0.2432540810000105580 ) ) ;
#15640=CARTESIAN_POINT ( 'NONE',  ( 17.14656078602323319, -7.900182044548062166, -1.000005633855494125E-09 ) ) ;
#15645=CARTESIAN_POINT ( 'NONE',  ( -23.94167924027569327, -14.12976891190553452, 6.079852602000002548 ) ) ;
#15650=CARTESIAN_POINT ( 'NONE',  ( -23.29312071521372118, -15.17488101142239643, 5.506989586000016423 ) ) ;
#15653=CARTESIAN_POINT ( 'NONE',  ( 24.74993095443131352, -14.13250376055072266, 3.957489350000009676 ) ) ;
#15656=B_SPLINE_CURVE_WITH_KNOTS ( 'NONE', 3,
 ( #8804, #16357, #30534, #28005 ),
 .UNSPECIFIED., .F., .F.,
 ( 4, 4 ),
 ( 0.000000000000000000, 1.000000000000000000 ),
 .UNSPECIFIED. ) ;
#15660=CARTESIAN_POINT ( 'NONE',  ( -26.79556473285982321, -0.4875557887251183442, -0.6999999999999784173 ) ) ;
#15668=CARTESIAN_POINT ( 'NONE',  ( 14.20787920732396969, -27.27274267807110775, 0.5514294940000274980 ) ) ;
#15669=ORIENTED_EDGE ( 'NONE', *, *, #26420, .F. ) ;
#15672=CARTESIAN_POINT ( 'NONE',  ( 0.7509949761426776282, 3.448174246630131279, 0.000000000000000000 ) ) ;
#15674=CARTESIAN_POINT ( 'NONE',  ( -26.13752726800887771, 9.883145870918147224, 8.000000000000007105 ) ) ;
#15676=EDGE_CURVE ( 'NONE', #30352, #25224, #1725, .T. ) ;
#15678=EDGE_LOOP ( 'NONE', ( #28341, #30523, #24769, #8715 ) ) ;
#15679=CARTESIAN_POINT ( 'NONE',  ( 28.49528339128749366, 0.5184828350247233653, 1.000000000000000888 ) ) ;
#15688=DIRECTION ( 'NONE',  ( 0.7198537139083028835, -0.6941258031311204890, 0.000000000000000000 ) ) ;
#15693=ORIENTED_EDGE ( 'NONE', *, *, #5031, .F. ) ;
#15701=ORIENTED_EDGE ( 'NONE', *, *, #22817, .F. ) ;
#15702=ORIENTED_EDGE ( 'NONE', *, *, #16401, .T. ) ;
#15703=CARTESIAN_POINT ( 'NONE',  ( -17.90616261956523303, -9.270408387734455857, 0.000000000000000000 ) ) ;
#15721=CARTESIAN_POINT ( 'NONE',  ( 3.843559591276155540, -27.68757158912330496, 8.000000000000007105 ) ) ;
#15733=ORIENTED_EDGE ( 'NONE', *, *, #5042, .T. ) ;
#15766=CARTESIAN_POINT ( 'NONE',  ( 17.47295178686619010, 9.934232311478513822, -0.6999999999999785283 ) ) ;
#15769=CARTESIAN_POINT ( 'NONE',  ( -17.70100621815563713, 10.30852736142610659, 0.000000000000000000 ) ) ;
#15798=EDGE_CURVE ( 'NONE', #1647, #21140, #1124, .T. ) ;
#15811=CARTESIAN_POINT ( 'NONE',  ( -24.61381496323305740, -14.36755986783201777, 6.042472825000033687 ) ) ;
#15816=CARTESIAN_POINT ( 'NONE',  ( 26.93696268452646336, 0.4901285798019155981, 0.000000000000000000 ) ) ;
#15818=LINE ( 'NONE', #3856, #13523 ) ;
#15823=CARTESIAN_POINT ( 'NONE',  ( 24.90302311548996883, -13.86047864964742793, 3.901342110999989288 ) ) ;
#15838=CARTESIAN_POINT ( 'NONE',  ( -16.83342759582943060, -8.999999999996580513, -0.6999999999999784173 ) ) ;
#15845=CARTESIAN_POINT ( 'NONE',  ( -25.52817993772956484, 13.14824702356417241, 8.000000000000007105 ) ) ;
#15846=CARTESIAN_POINT ( 'NONE',  ( -24.12025211354654886, 13.88308537690706324, 8.000000000000007105 ) ) ;
#15851=CARTESIAN_POINT ( 'NONE',  ( 4.785280386532176244, 31.71089591181006639, 8.000000000000007105 ) ) ;
#15865=B_SPLINE_CURVE_WITH_KNOTS ( 'NONE', 1,
 ( #25920, #4194 ),
 .UNSPECIFIED., .F., .F.,
 ( 2, 2 ),
 ( -2.555864960449999711E-06, 0.7000000000009999335 ),
 .UNSPECIFIED. ) ;
#15867=ADVANCED_FACE ( 'NONE', ( #18863 ), #28926, .F. ) ;
#15891=CARTESIAN_POINT ( 'NONE',  ( 15.33917451568712842, -24.20553497015958300, 8.000000000000007105 ) ) ;
#15892=CARTESIAN_POINT ( 'NONE',  ( -19.80535357377644701, 19.50875577052588739, 0.9999999989999952543 ) ) ;
#15894=CARTESIAN_POINT ( 'NONE',  ( 22.11577621125299586, 17.85147953289403944, -0.2432540810000105580 ) ) ;
#15897=ORIENTED_EDGE ( 'NONE', *, *, #6513, .T. ) ;
#15912=CARTESIAN_POINT ( 'NONE',  ( 0.2722179827847738820, -28.49915599490020668, 3.920205022000022854 ) ) ;
#15915=CARTESIAN_POINT ( 'NONE',  ( 23.84773733367773829, -14.28804811815363962, 4.437381894575493924 ) ) ;
#15922=CARTESIAN_POINT ( 'NONE',  ( 24.70448873180906446, -12.74983733560190302, 5.760266709000011254 ) ) ;
#15940=ORIENTED_EDGE ( 'NONE', *, *, #20994, .T. ) ;
#15955=CARTESIAN_POINT ( 'NONE',  ( -17.99933668381276775, 20.17941515429619415, -0.6999999999999784173 ) ) ;
#15958=CARTESIAN_POINT ( 'NONE',  ( -24.98823330661245379, 13.70626928206978690, 3.904029301000005781 ) ) ;
#15959=PRODUCT_DEFINITION_CONTEXT ( 'detailed design', #6577, 'design' ) ;
#15962=CARTESIAN_POINT ( 'NONE',  ( -28.49528339128749366, -0.5184828350247804307, 0.7595836940000044724 ) ) ;
#15968=CARTESIAN_POINT ( 'NONE',  ( 27.00728089375858687, 4.961773542941180004, 0.02487529600000981667 ) ) ;
#15974=CARTESIAN_POINT ( 'NONE',  ( 24.00289804085882039, -14.02635914341071732, 4.098597479000015475 ) ) ;
#15978=ADVANCED_FACE ( 'NONE', ( #10970, #25130 ), #5363, .F. ) ;
#15980=DIRECTION ( 'NONE',  ( -0.6941258031311203780, -0.7198537139083029945, 0.000000000000000000 ) ) ;
#15989=CARTESIAN_POINT ( 'NONE',  ( -27.79539923781770483, -0.5057481688778047157, 1.000000000000000888 ) ) ;
#15996=CARTESIAN_POINT ( 'NONE',  ( 0.2722179827847738820, -28.49915599490020668, 3.920205022000022854 ) ) ;
#15998=ADVANCED_FACE ( 'NONE', ( #13642, #23246, #1687, #11287, #16151, #30490 ), #8912, .T. ) ;
#15999=CARTESIAN_POINT ( 'NONE',  ( -16.04158896040112126, -9.763537949678049443, 0.000000000000000000 ) ) ;
#16008=CARTESIAN_POINT ( 'NONE',  ( 23.31033037370282202, 15.14834847481879265, 4.441258569420641678 ) ) ;
#16016=ORIENTED_EDGE ( 'NONE', *, *, #284, .F. ) ;
#16032=CARTESIAN_POINT ( 'NONE',  ( -17.62526668104891314, 11.76353838341477953, 0.000000000000000000 ) ) ;
#16036=ADVANCED_FACE ( 'NONE', ( #12055 ), #24022, .F. ) ;
#16040=EDGE_CURVE ( 'NONE', #11379, #1647, #4137, .T. ) ;
#16045=CARTESIAN_POINT ( 'NONE',  ( -19.80535357387461204, 19.50875577042408793, 0.9260390330000090042 ) ) ;
#16046=CARTESIAN_POINT ( 'NONE',  ( -8.175142068926048111, -27.46593847456960091, 8.000000000000007105 ) ) ;
#16048=CARTESIAN_POINT ( 'NONE',  ( 25.95386538600433468, 9.395593539459452970, -0.6999999999999784173 ) ) ;
#16054=B_SPLINE_CURVE_WITH_KNOTS ( 'NONE', 1,
 ( #17806, #20182 ),
 .UNSPECIFIED., .F., .F.,
 ( 2, 2 ),
 ( -2.556331299420000144E-06, 0.7000000000009999335 ),
 .UNSPECIFIED. ) ;
#16061=VERTEX_POINT ( 'NONE', #14268 ) ;
#16070=FACE_OUTER_BOUND ( 'NONE', #751, .T. ) ;
#16071=CARTESIAN_POINT ( 'NONE',  ( 17.93011078765611543, -8.208160914697428368, 0.000000000000000000 ) ) ;
#16084=CARTESIAN_POINT ( 'NONE',  ( -17.59696597919420213, 10.20816091468181774, 0.000000000000000000 ) ) ;
#16085=CARTESIAN_POINT ( 'NONE',  ( 1.592882851206511186, -27.75460863273100998, 5.208113774000016960 ) ) ;
#16102=ORIENTED_EDGE ( 'NONE', *, *, #29602, .T. ) ;
#16105=CARTESIAN_POINT ( 'NONE',  ( 28.49528339128749366, 0.5184828350247753237, 8.000000000000007105 ) ) ;
#16107=ADVANCED_FACE ( 'NONE', ( #19293 ), #9880, .F. ) ;
#16109=CARTESIAN_POINT ( 'NONE',  ( -22.62479587716020291, 18.00962536120669810, 1.000000000000000888 ) ) ;
#16113=CARTESIAN_POINT ( 'NONE',  ( -19.47854282320343700, 20.00003316006251097, -0.2808666865635076060 ) ) ;
#16117=CARTESIAN_POINT ( 'NONE',  ( -27.03594125075309762, -0.4919295335571652328, -0.6999999999999784173 ) ) ;
#16126=FACE_OUTER_BOUND ( 'NONE', #4989, .T. ) ;
#16131=CARTESIAN_POINT ( 'NONE',  ( -0.4822370987978389367, -3.496762477110187284, -0.6999999999999784173 ) ) ;
#16145=CARTESIAN_POINT ( 'NONE',  ( -2.347741120694188055, 2.634769306325225102, 0.000000000000000000 ) ) ;
#16147=CARTESIAN_POINT ( 'NONE',  ( 0.03635086285233400660, -28.50041301604787947, 3.997479608999987555 ) ) ;
#16151=FACE_BOUND ( 'NONE', #967, .T. ) ;
#16165=CARTESIAN_POINT ( 'NONE',  ( 24.36724931188768650, 13.38201648792073684, 4.999998581000003384 ) ) ;
#16166=DIRECTION ( 'NONE',  ( 0.000000000000000000, 0.000000000000000000, -1.000000000000000000 ) ) ;
#16167=DIRECTION ( 'NONE',  ( 0.000000000000000000, 0.000000000000000000, -1.000000000000000000 ) ) ;
#16169=B_SPLINE_CURVE_WITH_KNOTS ( 'NONE', 5,
 ( #10445, #8213, #556, #20039, #29637, #10596 ),
 .UNSPECIFIED., .F., .F.,
 ( 6, 6 ),
 ( -17.34990440099999987, 0.000000000000000000 ),
 .UNSPECIFIED. ) ;
#16189=ORIENTED_EDGE ( 'NONE', *, *, #10606, .F. ) ;
#16190=DIRECTION ( 'NONE',  ( 0.000000000000000000, 0.000000000000000000, -1.000000000000000000 ) ) ;
#16195=CARTESIAN_POINT ( 'NONE',  ( 24.29903249413439781, 13.50560429725452849, 4.442423594862364489 ) ) ;
#16197=CARTESIAN_POINT ( 'NONE',  ( 27.84775205013805888, -6.760390605069130032, 8.000000000000007105 ) ) ;
#16203=CARTESIAN_POINT ( 'NONE',  ( 20.30396079652883756, 20.00000000004620304, 1.000000000000000888 ) ) ;
#16208=EDGE_CURVE ( 'NONE', #15627, #2709, #20628, .T. ) ;
#16233=CARTESIAN_POINT ( 'NONE',  ( -25.46368746807222649, 12.80129684246671751, 5.147587686977050048 ) ) ;
#16236=CARTESIAN_POINT ( 'NONE',  ( 1.605176535610508326, -27.75389821387976852, 4.999998581000003384 ) ) ;
#16242=ORIENTED_EDGE ( 'NONE', *, *, #20758, .F. ) ;
#16252=ORIENTED_EDGE ( 'NONE', *, *, #28848, .T. ) ;
#16264=CARTESIAN_POINT ( 'NONE',  ( -19.89484633387414902, 20.00030665124463169, 0.04277443887995936722 ) ) ;
#16268=CARTESIAN_POINT ( 'NONE',  ( -28.45300238704230367, -0.5177135156027794505, 0.5017677510000262409 ) ) ;
#16270=CARTESIAN_POINT ( 'NONE',  ( 16.06675444873834380, 10.97998838177521286, -0.6999999999999784173 ) ) ;
#16276=LINE ( 'NONE', #1976, #27800 ) ;
#16277=DIRECTION ( 'NONE',  ( 0.000000000000000000, 0.000000000000000000, -1.000000000000000000 ) ) ;
#16281=CARTESIAN_POINT ( 'NONE',  ( 16.06675444876397307, -9.020011618195203695, -0.6999999999999784173 ) ) ;
#16288=FACE_OUTER_BOUND ( 'NONE', #4450, .T. ) ;
#16292=( GEOMETRIC_REPRESENTATION_CONTEXT ( 3 ) GLOBAL_UNCERTAINTY_ASSIGNED_CONTEXT ( ( #14724 ) ) GLOBAL_UNIT_ASSIGNED_CONTEXT ( ( #13777, #9832, #12346 ) ) REPRESENTATION_CONTEXT ( 'NONE', 'WORKASPACE' ) );
#16307=CARTESIAN_POINT ( 'NONE',  ( -16.19903397984253957, -9.902734965364627939, 0.000000000000000000 ) ) ;
#16314=CARTESIAN_POINT ( 'NONE',  ( -15.99701729020289243, -9.715560209340530662, 0.000000000000000000 ) ) ;
#16315=CARTESIAN_POINT ( 'NONE',  ( 16.89818815097801519, -10.07643063672789019, -0.6999999999999785283 ) ) ;
#16318=CARTESIAN_POINT ( 'NONE',  ( 13.73773747404255552, -26.37022765825810922, 0.000000000000000000 ) ) ;
#16322=CARTESIAN_POINT ( 'NONE',  ( -27.79539923781770128, -0.5057481688779147389, 8.000000000000007105 ) ) ;
#16332=VERTEX_POINT ( 'NONE', #30127 ) ;
#16342=CARTESIAN_POINT ( 'NONE',  ( -27.66290831536099759, -7.787312998881454895, 1.000000000000000888 ) ) ;
#16350=CARTESIAN_POINT ( 'NONE',  ( 24.36724931188768650, 13.38201648792073684, 4.999998581000003384 ) ) ;
#16351=CARTESIAN_POINT ( 'NONE',  ( -18.31085446006445494, 19.88197403644849004, 0.02160863700001458554 ) ) ;
#16355=CARTESIAN_POINT ( 'NONE',  ( 27.35479945376005873, 9.902747534594007917, 0.7595836940000044724 ) ) ;
#16357=CARTESIAN_POINT ( 'NONE',  ( -20.97469196846414974, 18.32172385076221488, 4.666666738000063930 ) ) ;
#16367=EDGE_LOOP ( 'NONE', ( #8112, #21173, #25156, #27291 ) ) ;
#16376=CARTESIAN_POINT ( 'NONE',  ( 23.23277125981546476, 15.26692728828886025, 4.999998581000003384 ) ) ;
#16377=CARTESIAN_POINT ( 'NONE',  ( -24.38199545545641911, -14.75707035126829147, 3.901343066999990228 ) ) ;
#16380=CARTESIAN_POINT ( 'NONE',  ( 18.59033486452720041, 20.00000077194644277, -0.6230606123292589116 ) ) ;
#16390=PLANE ( 'NONE',  #22732 ) ;
#16400=CARTESIAN_POINT ( 'NONE',  ( -24.70074544867652122, 14.21822122508601716, 6.002806299999996043 ) ) ;
#16401=EDGE_CURVE ( 'NONE', #5736, #17991, #30776, .T. ) ;
#16414=CYLINDRICAL_SURFACE ( 'NONE', #609, 1.099999999999999867 ) ;
#16430=CARTESIAN_POINT ( 'NONE',  ( 1.632956991020356519, -28.45346066249067007, 4.791883387999989807 ) ) ;
#16431=CARTESIAN_POINT ( 'NONE',  ( 3.040504021322313122, 1.733590290792417887, 0.000000000000000000 ) ) ;
#16444=VECTOR ( 'NONE', #15292, 1000.000000000000000 ) ;
#16469=CARTESIAN_POINT ( 'NONE',  ( -24.50348397099046593, 13.13223627435659857, 3.957489296000010981 ) ) ;
#16470=CYLINDRICAL_SURFACE ( 'NONE', #8571, 1.100000000000002309 ) ;
#16484=AXIS2_PLACEMENT_3D ( 'NONE', #7248, #21891, #24398 ) ;
#16488=EDGE_CURVE ( 'NONE', #1557, #27319, #7475, .T. ) ;
#16493=CARTESIAN_POINT ( 'NONE',  ( 20.30396079662882158, 20.00000000004802203, 3.000000000000002665 ) ) ;
#16501=CARTESIAN_POINT ( 'NONE',  ( 26.33366376410667797, 9.374780377579124746, 8.000000000000007105 ) ) ;
#16505=CARTESIAN_POINT ( 'NONE',  ( 23.05336736746781767, -19.64267831869096881, -0.6577119969999878357 ) ) ;
#16508=CARTESIAN_POINT ( 'NONE',  ( -19.68703433251029722, 19.53817007346649248, 0.6302326600000074386 ) ) ;
#16529=CARTESIAN_POINT ( 'NONE',  ( 24.29089620522634263, 14.90695587088477581, 3.920145809000019632 ) ) ;
#16531=CARTESIAN_POINT ( 'NONE',  ( -23.87963657974984955, -15.55698410977798929, 4.493007575000013354 ) ) ;
#16543=CARTESIAN_POINT ( 'NONE',  ( 24.36724935763797006, 13.38201651305720574, 4.999998581000003384 ) ) ;
#16544=CARTESIAN_POINT ( 'NONE',  ( -24.93720648713954446, 13.79881813474513486, 6.099998581000020792 ) ) ;
#16548=CARTESIAN_POINT ( 'NONE',  ( 0.6243462152986178904, -28.49342029039284085, 6.095948809000023338 ) ) ;
#16551=ORIENTED_EDGE ( 'NONE', *, *, #25585, .F. ) ;
#16553=CYLINDRICAL_SURFACE ( 'NONE', #29883, 3.500000000000003109 ) ;
#16562=ORIENTED_EDGE ( 'NONE', *, *, #17928, .T. ) ;
#16583=CARTESIAN_POINT ( 'NONE',  ( 17.93011078763067090, 11.79183908526299085, -0.6999999999999784173 ) ) ;
#16589=CARTESIAN_POINT ( 'NONE',  ( 16.06937396340397939, -9.163977451780842998, -0.6999999999999784173 ) ) ;
#16596=ORIENTED_EDGE ( 'NONE', *, *, #3808, .F. ) ;
#16608=CARTESIAN_POINT ( 'NONE',  ( -24.41841039498785193, -14.69667350221323865, 3.899998581000013509 ) ) ;
#16610=UNCERTAINTY_MEASURE_WITH_UNIT (LENGTH_MEASURE( 1.000000000000000082E-05 ), #5103, 'distance_accuracy_value', 'NONE');
#16615=CARTESIAN_POINT ( 'NONE',  ( 24.93720649360215802, -13.79881813812812297, 6.099998581000020792 ) ) ;
#16619=CARTESIAN_POINT ( 'NONE',  ( 16.40303402077768169, -9.791839085275103827, -0.6999999999999784173 ) ) ;
#16622=CARTESIAN_POINT ( 'NONE',  ( -24.78870452934888746, 12.58522324287992866, 4.492873454000012146 ) ) ;
#16628=CARTESIAN_POINT ( 'NONE',  ( 24.83401022448529005, 13.98326749045440032, 5.760125282000011282 ) ) ;
#16634=VERTEX_POINT ( 'NONE', #7750 ) ;
#16645=CARTESIAN_POINT ( 'NONE',  ( -27.08859402333795430, -0.4928875713624365495, 0.02487529600000981667 ) ) ;
#16646=FACE_OUTER_BOUND ( 'NONE', #1014, .T. ) ;
#16663=EDGE_LOOP ( 'NONE', ( #20465, #14375, #22464, #23297 ) ) ;
#16665=CARTESIAN_POINT ( 'NONE',  ( -15.94126856070501930, -9.659453305974544435, -0.6999999999999783062 ) ) ;
#16680=CARTESIAN_POINT ( 'NONE',  ( -23.98258507372315051, -15.39789217239198571, 4.239862999000004962 ) ) ;
#16682=CARTESIAN_POINT ( 'NONE',  ( 20.02191110107359506, 20.00001381684630530, 0.1993976363602749657 ) ) ;
#16683=CARTESIAN_POINT ( 'NONE',  ( -24.88589369081283920, 13.89120818323882922, 6.095967889000020179 ) ) ;
#16689=CARTESIAN_POINT ( 'NONE',  ( 1.758512962375676780, -3.081546181689937658, 0.000000000000000000 ) ) ;
#16691=CARTESIAN_POINT ( 'NONE',  ( 24.54452541844319668, 14.48555669908156851, 6.079852602000002548 ) ) ;
#16709=ORIENTED_EDGE ( 'NONE', *, *, #11604, .F. ) ;
#16711=DIRECTION ( 'NONE',  ( 0.000000000000000000, 0.000000000000000000, -1.000000000000000000 ) ) ;
#16719=ORIENTED_EDGE ( 'NONE', *, *, #1764, .T. ) ;
#16720=CARTESIAN_POINT ( 'NONE',  ( -19.67781185827837831, 20.00028292424892840, -0.1456647343256203542 ) ) ;
#16726=CARTESIAN_POINT ( 'NONE',  ( -23.53065194457538567, -14.80430352413842421, 4.036042474887940656 ) ) ;
#16738=CARTESIAN_POINT ( 'NONE',  ( -27.85770179432011417, 4.285683232258365116, 0.7069222069999991920 ) ) ;
#16749=CARTESIAN_POINT ( 'NONE',  ( 23.83437493589245193, 15.62616282937172940, 5.290530241274704615 ) ) ;
#16756=ADVANCED_FACE ( 'NONE', ( #1773, #28348, #6793, #4583, #25996, #31023 ), #16390, .F. ) ;
#16766=VECTOR ( 'NONE', #16167, 1000.000000000000000 ) ;
#16775=CARTESIAN_POINT ( 'NONE',  ( -24.98823330661245379, 13.70626928206978690, 3.904029301000005781 ) ) ;
#16778=B_SPLINE_SURFACE_WITH_KNOTS ( 'NONE', 5, 5, ( 
 ( #3360, #5572, #22724, #24623, #15633, #15171, #3056, #718, #24776 ),
 ( #12967, #25086, #17982, #5876, #22577, #29650, #25244, #7927, #10152 ),
 ( #1021, #19749, #12653, #3211, #8079, #12819, #10309, #867, #3516 ),
 ( #13115, #22111, #10460, #1170, #17672, #29332, #10609, #17376, #27285 ),
 ( #5728, #26981, #29955, #20204, #5420, #10761, #29795, #27594, #16109 ),
 ( #1955, #15955, #25878, #23202, #4155, #30596, #11549, #27915, #6821 ) ),
 .UNSPECIFIED., .F., .F., .F.,
 ( 6, 6 ),
 ( 6, 3, 6 ),
 ( 0.000000000000000000, 24.33438218110000051 ),
 ( 8.011061266649999624, 9.372561696260000019, 10.73406212590000131 ),
 .UNSPECIFIED. ) ;
#16785=ORIENTED_EDGE ( 'NONE', *, *, #26769, .F. ) ;
#16798=CARTESIAN_POINT ( 'NONE',  ( 18.26639035967037827, -8.979988381807324060, -0.6999999989999727834 ) ) ;
#16801=CARTESIAN_POINT ( 'NONE',  ( -20.30403093128963476, 20.00000000003735323, 1.400000021000019634 ) ) ;
#16806=CARTESIAN_POINT ( 'NONE',  ( -19.80535357377644701, 19.50875577052588739, 3.000000106999994642 ) ) ;
#16811=CARTESIAN_POINT ( 'NONE',  ( -24.37165444408190851, 14.77472139917419369, 4.999998581000003384 ) ) ;
#16813=CARTESIAN_POINT ( 'NONE',  ( -17.83930458829795640, 19.99999999999961631, -0.6999999999999784173 ) ) ;
#16829=VERTEX_POINT ( 'NONE', #5508 ) ;
#16830=CARTESIAN_POINT ( 'NONE',  ( 24.83827472153076599, -12.48687851163286133, 4.895780544000027490 ) ) ;
#16840=CARTESIAN_POINT ( 'NONE',  ( 17.70481770901024632, 11.96970539787597509, -0.6999999999999785283 ) ) ;
#16847=CARTESIAN_POINT ( 'NONE',  ( 17.18658402241074867, -10.09981795543446736, -1.000005633855494125E-09 ) ) ;
#16851=CARTESIAN_POINT ( 'NONE',  ( 3.448453739143401808, -0.7497105383105261422, 0.000000000000000000 ) ) ;
#16854=CARTESIAN_POINT ( 'NONE',  ( 24.29138541237941240, -13.52003710528471281, 6.098655051000018368 ) ) ;
#16855=CARTESIAN_POINT ( 'NONE',  ( 19.79257030269742756, 19.51192911135138175, 0.8505974720000031297 ) ) ;
#16858=CARTESIAN_POINT ( 'NONE',  ( -24.47278419579111386, -14.60601539740217092, 3.904031772999999816 ) ) ;
#16861=B_SPLINE_CURVE_WITH_KNOTS ( 'NONE', 5,
 ( #13653, #30172, #1698, #2015, #23258, #25627, #8602, #21053, #6258 ),
 .UNSPECIFIED., .F., .F.,
 ( 6, 3, 6 ),
 ( 8.011061266649999624, 8.831591450809998634, 9.652121634960000307 ),
 .UNSPECIFIED. ) ;
#16869=ORIENTED_EDGE ( 'NONE', *, *, #20772, .F. ) ;
#16870=VERTEX_POINT ( 'NONE', #7410 ) ;
#16873=EDGE_CURVE ( 'NONE', #14390, #5681, #26761, .T. ) ;
#16874=CARTESIAN_POINT ( 'NONE',  ( 17.93011078765611543, -8.208160914697428368, 0.000000000000000000 ) ) ;
#16879=CARTESIAN_POINT ( 'NONE',  ( 19.68707593455170368, 19.53815609463533320, 0.6304112420000007599 ) ) ;
#16883=ADVANCED_FACE ( 'NONE', ( #2688 ), #7615, .F. ) ;
#16884=CARTESIAN_POINT ( 'NONE',  ( -18.31680438778779418, 19.99999316982339437, -0.6696325988070516155 ) ) ;
#16905=ORIENTED_EDGE ( 'NONE', *, *, #20250, .F. ) ;
#16907=CARTESIAN_POINT ( 'NONE',  ( 0.7459188900473354700, -27.79046661982714639, 3.920206710000012862 ) ) ;
#16908=ORIENTED_EDGE ( 'NONE', *, *, #19887, .T. ) ;
#16912=B_SPLINE_CURVE_WITH_KNOTS ( 'NONE', 1,
 ( #10136, #12339 ),
 .UNSPECIFIED., .F., .F.,
 ( 2, 2 ),
 ( -3.500000000000000000, 3.500000000000000000 ),
 .UNSPECIFIED. ) ;
#16914=CARTESIAN_POINT ( 'NONE',  ( -23.80092421045090489, -14.36517094966148633, 3.899998581000013509 ) ) ;
#16924=CARTESIAN_POINT ( 'NONE',  ( -23.82471740849593544, -15.64077206322649083, 5.208368890000008911 ) ) ;
#16960=CARTESIAN_POINT ( 'NONE',  ( -20.26572724632349320, -21.15151735177849091, 8.000000000000007105 ) ) ;
#16969=CARTESIAN_POINT ( 'NONE',  ( -18.41897712746086668, 20.00000741691685846, -0.6632653549999978360 ) ) ;
#16973=LINE ( 'NONE', #7379, #22302 ) ;
#16984=CARTESIAN_POINT ( 'NONE',  ( 24.44014313072642963, -13.24968496497942105, 3.920132093000017193 ) ) ;
#16987=ORIENTED_EDGE ( 'NONE', *, *, #2303, .T. ) ;
#16995=CARTESIAN_POINT ( 'NONE',  ( 27.07818553041514065, 6.807801137122736712, 1.000000000000000888 ) ) ;
#17001=CARTESIAN_POINT ( 'NONE',  ( -24.39135169139800041, 14.74223402946396000, 5.310643621000004977 ) ) ;
#17010=CARTESIAN_POINT ( 'NONE',  ( 23.87170004953230773, 14.24726900334573187, 6.095965388000001539 ) ) ;
#17011=CARTESIAN_POINT ( 'NONE',  ( -17.62526668104891314, 11.76353838341477953, -0.6999999999999784173 ) ) ;
#17034=CARTESIAN_POINT ( 'NONE',  ( -25.46368746804859740, 12.80129684245613575, 5.104216618000034345 ) ) ;
#17057=CARTESIAN_POINT ( 'NONE',  ( -27.52676963214367944, -0.5008603480904468830, 0.2686740700000300741 ) ) ;
#17060=EDGE_CURVE ( 'NONE', #6349, #13182, #3603, .T. ) ;
#17062=SURFACE_STYLE_USAGE ( .BOTH. , #7008 ) ;
#17077=EDGE_CURVE ( 'NONE', #2594, #27396, #27221, .T. ) ;
#17079=CARTESIAN_POINT ( 'NONE',  ( -15.73360964030186970, 11.02001161816959396, -1.000005633855494125E-09 ) ) ;
#17086=CARTESIAN_POINT ( 'NONE',  ( -25.77914833258148164, -15.40383343755785361, 1.000000000000000888 ) ) ;
#17088=CARTESIAN_POINT ( 'NONE',  ( -25.35851007062240114, 13.00862288638852959, 4.319165764000016061 ) ) ;
#17090=EDGE_CURVE ( 'NONE', #2594, #21789, #23987, .T. ) ;
#17091=B_SPLINE_CURVE_WITH_KNOTS ( 'NONE', 3,
 ( #13353, #1090, #15403, #13509, #20277, #22800 ),
 .UNSPECIFIED., .F., .F.,
 ( 4, 2, 4 ),
 ( 0.000000000000000000, 0.5000000000000000000, 1.000000000000000000 ),
 .UNSPECIFIED. ) ;
#17095=VERTEX_POINT ( 'NONE', #3773 ) ;
#17123=CARTESIAN_POINT ( 'NONE',  ( -18.03078366343508421, 19.99999999996890665, -0.6999999999999784173 ) ) ;
#17133=CARTESIAN_POINT ( 'NONE',  ( 24.98823331316959440, -13.70626928515100573, 3.904029301000005781 ) ) ;
#17153=CARTESIAN_POINT ( 'NONE',  ( -2.858922298043036214, -2.052062286655957024, 0.000000000000000000 ) ) ;
#17156=CARTESIAN_POINT ( 'NONE',  ( -17.52370713000112090, 11.86883708413922811, -0.6999999999999784173 ) ) ;
#17159=B_SPLINE_SURFACE_WITH_KNOTS ( 'NONE', 5, 1, ( 
 ( #2988, #176 ),
 ( #14495, #7849 ),
 ( #7698, #26447 ),
 ( #5185, #26910 ),
 ( #19831, #21724 ),
 ( #16995, #26600 ),
 ( #5347, #14952 ),
 ( #12578, #5039 ),
 ( #22342, #24090 ) ),
 .UNSPECIFIED., .F., .F., .F.,
 ( 6, 3, 6 ),
 ( 2, 2 ),
 ( 67.22752578339999729, 77.81866039000000512, 88.40979499649999696 ),
 ( -3.500000000000000000, 3.500000000000000000 ),
 .UNSPECIFIED. ) ;
#17182=CARTESIAN_POINT ( 'NONE',  ( 17.04261818930491401, 9.897562529765991712, -0.6999999999999783062 ) ) ;
#17195=CARTESIAN_POINT ( 'NONE',  ( 0.5057536231481193356, -27.79562098839016571, 3.899998581000013509 ) ) ;
#17212=EDGE_LOOP ( 'NONE', ( #24955, #15291, #14600, #29011 ) ) ;
#17215=ORIENTED_EDGE ( 'NONE', *, *, #10597, .T. ) ;
#17233=CARTESIAN_POINT ( 'NONE',  ( 17.18658402238548533, 9.900182044515950963, -0.6999999999999784173 ) ) ;
#17234=LINE ( 'NONE', #5742, #23720 ) ;
#17237=CARTESIAN_POINT ( 'NONE',  ( -28.49528339128749366, -0.5184828350247816520, 0.7595836940000044724 ) ) ;
#17238=CARTESIAN_POINT ( 'NONE',  ( 23.81866167241657806, 14.33570040768432996, 6.099998581000020792 ) ) ;
#17239=CARTESIAN_POINT ( 'NONE',  ( 24.37165445055180157, -14.77472140295711434, 4.999998581000003384 ) ) ;
#17240=CARTESIAN_POINT ( 'NONE',  ( 17.14656078599760392, 12.09981795542235439, -1.000005633855494125E-09 ) ) ;
#17243=CYLINDRICAL_SURFACE ( 'NONE', #7778, 1.099999999999999867 ) ;
#17246=CARTESIAN_POINT ( 'NONE',  ( 20.30396079662882158, 20.00000000004802203, 2.600000000000019185 ) ) ;
#17249=ORIENTED_EDGE ( 'NONE', *, *, #28551, .F. ) ;
#17258=CARTESIAN_POINT ( 'NONE',  ( -24.70074544867652122, 14.21822122508601716, 3.997190861000005313 ) ) ;
#17270=EDGE_CURVE ( 'NONE', #17343, #11027, #24694, .T. ) ;
#17272=CARTESIAN_POINT ( 'NONE',  ( 28.43005475791858672, 2.264356203195492689, 8.000000000000007105 ) ) ;
#17273=CARTESIAN_POINT ( 'NONE',  ( -16.81341597756113515, 9.900182044522454206, -1.000005633855494125E-09 ) ) ;
#17285=DIRECTION ( 'NONE',  ( 0.000000000000000000, 0.000000000000000000, -1.000000000000000000 ) ) ;
#17315=DIRECTION ( 'NONE',  ( 0.000000000000000000, 0.000000000000000000, -1.000000000000000000 ) ) ;
#17316=CARTESIAN_POINT ( 'NONE',  ( 20.30396079662882158, 20.00000000004802203, 1.000000000000000888 ) ) ;
#17321=CARTESIAN_POINT ( 'NONE',  ( -24.05769994060051786, -13.93129956160059102, 3.997248602000014195 ) ) ;
#17335=VECTOR ( 'NONE', #22374, 1000.000000000000000 ) ;
#17339=EDGE_LOOP ( 'NONE', ( #25153, #325, #20872, #19784 ) ) ;
#17343=VERTEX_POINT ( 'NONE', #7148 ) ;
#17345=CARTESIAN_POINT ( 'NONE',  ( 4.785280386532176244, 31.71089591181006639, 8.000000000000007105 ) ) ;
#17352=CARTESIAN_POINT ( 'NONE',  ( 24.29878022517171132, 13.50606022452295996, 5.558728318588544326 ) ) ;
#17355=CARTESIAN_POINT ( 'NONE',  ( -24.58829991325495001, 12.97289974774663790, 4.038486474265504000 ) ) ;
#17363=CARTESIAN_POINT ( 'NONE',  ( -21.50791824780870698, 17.12055895076685630, 0.02487541500001411165 ) ) ;
#17366=ORIENTED_EDGE ( 'NONE', *, *, #26679, .F. ) ;
#17374=B_SPLINE_CURVE_WITH_KNOTS ( 'NONE', 3,
 ( #25484, #18545, #13189, #20752, #30359, #13673 ),
 .UNSPECIFIED., .F., .F.,
 ( 4, 2, 4 ),
 ( 0.000000000000000000, 0.5000000000000000000, 1.000000000000000000 ),
 .UNSPECIFIED. ) ;
#17376=CARTESIAN_POINT ( 'NONE',  ( -25.57973247310144771, 13.96556750272910641, 0.7595836940000044724 ) ) ;
#17383=CARTESIAN_POINT ( 'NONE',  ( 24.81746042554890863, -14.01353061607344053, 3.920132063000014710 ) ) ;
#17389=CARTESIAN_POINT ( 'NONE',  ( -24.34942396232675321, -13.41447636113284680, 5.310538869999992251 ) ) ;
#17395=CARTESIAN_POINT ( 'NONE',  ( -25.74089749696337037, -15.38097739005167419, 0.5017677510000262409 ) ) ;
#17399=CARTESIAN_POINT ( 'NONE',  ( -0.4846640835383786983, -27.79604706135651782, 5.506468674000009500 ) ) ;
#17408=CARTESIAN_POINT ( 'NONE',  ( -4.622623965551615477, -30.63307358560974336, 0.2686722299999888541 ) ) ;
#17410=EDGE_LOOP ( 'NONE', ( #13348, #13784, #22546, #11310 ) ) ;
#17411=CARTESIAN_POINT ( 'NONE',  ( 17.14656078599760392, 12.09981795542235439, -0.6999999999999784173 ) ) ;
#17412=CARTESIAN_POINT ( 'NONE',  ( -24.93720648713954446, 13.79881813474513486, 3.899998581000013509 ) ) ;
#17417=CARTESIAN_POINT ( 'NONE',  ( 24.95427444975690889, -13.76797447160702070, 6.099998581000020792 ) ) ;
#17421=VERTEX_POINT ( 'NONE', #24452 ) ;
#17423=CARTESIAN_POINT ( 'NONE',  ( 28.49528339128749366, 0.5184828350247212558, 1.000000000000000888 ) ) ;
#17440=ORIENTED_EDGE ( 'NONE', *, *, #13819, .T. ) ;
#17441=CARTESIAN_POINT ( 'NONE',  ( 24.70448873180906446, -12.74983733560190302, 4.239730452999995514 ) ) ;
#17452=CARTESIAN_POINT ( 'NONE',  ( -17.93324555120827668, 10.97998838178171432, -0.6999999999999784173 ) ) ;
#17464=CARTESIAN_POINT ( 'NONE',  ( 23.77307140678977504, -14.41181874416537134, 4.999998581000003384 ) ) ;
#17465=CARTESIAN_POINT ( 'NONE',  ( 17.83931306984926835, 20.00000000000176570, -0.6999999999999784173 ) ) ;
#17467=CARTESIAN_POINT ( 'NONE',  ( 28.49530731802708416, 0.5184832703811660393, 8.000000000000007105 ) ) ;
#17479=CARTESIAN_POINT ( 'NONE',  ( 27.89542231038745257, 7.122393016134455301, 8.000000000000007105 ) ) ;
#17485=EDGE_LOOP ( 'NONE', ( #8692, #6029, #14481, #28286 ) ) ;
#17493=CARTESIAN_POINT ( 'NONE',  ( -24.35797963555383205, 13.39969403207715892, 6.098655031999994591 ) ) ;
#17496=AXIS2_PLACEMENT_3D ( 'NONE', #28425, #4515, #21349 ) ;
#17515=CARTESIAN_POINT ( 'NONE',  ( 21.13530760622424864, 17.06006193249097436, 0.000000000000000000 ) ) ;
#17516=CARTESIAN_POINT ( 'NONE',  ( -21.27524652179786457, 16.93536700441368126, 0.000000000000000000 ) ) ;
#17522=ORIENTED_EDGE ( 'NONE', *, *, #29847, .T. ) ;
#17523=CYLINDRICAL_SURFACE ( 'NONE', #19000, 1.100000000000002309 ) ;
#17537=ORIENTED_EDGE ( 'NONE', *, *, #4535, .F. ) ;
#17539=CARTESIAN_POINT ( 'NONE',  ( -24.96253706803760153, -13.75225324404262572, 5.310538869999992251 ) ) ;
#17544=CARTESIAN_POINT ( 'NONE',  ( -4.761646371388416732, -31.55428150781402508, 0.2374258030000131470 ) ) ;
#17550=EDGE_CURVE ( 'NONE', #18290, #23153, #27310, .T. ) ;
#17552=CARTESIAN_POINT ( 'NONE',  ( 3.040504021322313122, 1.733590290792417887, -0.6999999999999784173 ) ) ;
#17557=EDGE_CURVE ( 'NONE', #30855, #24241, #16054, .T. ) ;
#17560=EDGE_LOOP ( 'NONE', ( #13419, #12657, #7216, #23940 ) ) ;
#17563=CARTESIAN_POINT ( 'NONE',  ( 26.97469346668950152, -9.357175201752722771, 0.000000000000000000 ) ) ;
#17567=CARTESIAN_POINT ( 'NONE',  ( 24.97129468909112404, -13.73710443560444183, 3.901342130000013064 ) ) ;
#17571=CARTESIAN_POINT ( 'NONE',  ( 25.45799949673341800, -12.81261086040661645, 5.208434320000010942 ) ) ;
#17572=CARTESIAN_POINT ( 'NONE',  ( 17.16657240419154462, 10.99999999996915179, -0.6999999999999784173 ) ) ;
#17599=ORIENTED_EDGE ( 'NONE', *, *, #11896, .F. ) ;
#17602=CARTESIAN_POINT ( 'NONE',  ( -17.59696554489119080, -9.791838634853515799, 0.000000000000000000 ) ) ;
#17622=ORIENTED_EDGE ( 'NONE', *, *, #24825, .F. ) ;
#17623=CARTESIAN_POINT ( 'NONE',  ( 24.40022624086872938, 14.72688605419589614, 6.099998581000020792 ) ) ;
#17626=CARTESIAN_POINT ( 'NONE',  ( 28.49528339128749366, 0.5184828350247753237, 8.000000000000007105 ) ) ;
#17637=VERTEX_POINT ( 'NONE', #6168 ) ;
#17640=CARTESIAN_POINT ( 'NONE',  ( -24.09790742087466597, -13.86182010774420625, 5.963951780225244192 ) ) ;
#17653=CARTESIAN_POINT ( 'NONE',  ( 0.4822370985009165056, 3.496762477156720728, -0.6999999999999784173 ) ) ;
#17660=CARTESIAN_POINT ( 'NONE',  ( 13.73773747404255552, -26.37022765825810922, -0.6999999999999784173 ) ) ;
#17669=CARTESIAN_POINT ( 'NONE',  ( 23.23277120357798964, 15.26692725135965745, 4.999998581000003384 ) ) ;
#17672=CARTESIAN_POINT ( 'NONE',  ( -25.16978723329435397, 13.74175290767721691, -0.2432540810000105580 ) ) ;
#17676=EDGE_CURVE ( 'NONE', #25227, #30352, #20568, .T. ) ;
#17688=CARTESIAN_POINT ( 'NONE',  ( 14.60916111673911288, -28.04296597555454085, 0.7595836940000044724 ) ) ;
#17694=CARTESIAN_POINT ( 'NONE',  ( 0.03549436706548679543, -27.80040766162893817, 6.002517553000020101 ) ) ;
#17707=CARTESIAN_POINT ( 'NONE',  ( 27.79539923781684507, 0.5057481689249165857, 0.8585786439999909536 ) ) ;
#17714=CARTESIAN_POINT ( 'NONE',  ( 25.41286869299526074, -12.90211872965451079, 5.507123706999989210 ) ) ;
#17722=AXIS2_PLACEMENT_3D ( 'NONE', #2627, #14015, #29203 ) ;
#17726=CARTESIAN_POINT ( 'NONE',  ( -24.93720648713954446, 13.79881813474513486, 6.099998581000020792 ) ) ;
#17739=ORIENTED_EDGE ( 'NONE', *, *, #6910, .F. ) ;
#17750=EDGE_CURVE ( 'NONE', #11379, #6771, #22797, .T. ) ;
#17763=CARTESIAN_POINT ( 'NONE',  ( 24.06826093652101051, -20.50742065841456707, 1.000000000000000888 ) ) ;
#17768=AXIS2_PLACEMENT_3D ( 'NONE', #25904, #6382, #15980 ) ;
#17770=CARTESIAN_POINT ( 'NONE',  ( 17.16657240421717390, -9.000000000001264766, -0.6999999999999784173 ) ) ;
#17772=CARTESIAN_POINT ( 'NONE',  ( 27.07818553041514065, 6.807801137122736712, 1.000000000000000888 ) ) ;
#17774=DIRECTION ( 'NONE',  ( 0.000000000000000000, 0.000000000000000000, -1.000000000000000000 ) ) ;
#17777=CARTESIAN_POINT ( 'NONE',  ( -16.04158851046123502, 10.23646161653652875, -0.6999999989999727834 ) ) ;
#17781=VERTEX_POINT ( 'NONE', #18908 ) ;
#17788=CARTESIAN_POINT ( 'NONE',  ( -17.93324555128263142, -9.020011618190519442, -0.6999999999999784173 ) ) ;
#17795=CARTESIAN_POINT ( 'NONE',  ( -0.4969045691271392617, -28.49594262166942116, 5.506468674000009500 ) ) ;
#17806=CARTESIAN_POINT ( 'NONE',  ( 0.5057536231481327693, -27.79562098839016571, 3.899998581000013509 ) ) ;
#17817=CARTESIAN_POINT ( 'NONE',  ( -26.67548192793729456, 9.015773298006253711, 0.2686740810000365354 ) ) ;
#17819=EDGE_CURVE ( 'NONE', #24853, #1904, #9308, .T. ) ;
#17825=CARTESIAN_POINT ( 'NONE',  ( -24.90302310912370132, 13.86047864606265279, 3.901342110999989288 ) ) ;
#17832=CARTESIAN_POINT ( 'NONE',  ( 16.06941601963802668, 10.83371123183088436, 0.000000000000000000 ) ) ;
#17839=ORIENTED_EDGE ( 'NONE', *, *, #1764, .F. ) ;
#17841=CARTESIAN_POINT ( 'NONE',  ( -24.00926694310947695, -14.01467022312833421, 6.042472825000033687 ) ) ;
#17842=CARTESIAN_POINT ( 'NONE',  ( -23.62421573606080827, -14.65442406347138338, 6.042470790000031400 ) ) ;
#17843=CARTESIAN_POINT ( 'NONE',  ( 26.00441062110688506, 9.413902731553067227, 0.02487529700001545052 ) ) ;
#17846=CARTESIAN_POINT ( 'NONE',  ( -15.73360964098195147, -8.979988381493612337, 0.000000000000000000 ) ) ;
#17870=CARTESIAN_POINT ( 'NONE',  ( 25.25401215828319579, -13.21081861402798374, 5.901400366999986602 ) ) ;
#17878=CARTESIAN_POINT ( 'NONE',  ( 27.79539923611798358, 0.5057481688468927761, 8.000000000000007105 ) ) ;
#17889=ORIENTED_EDGE ( 'NONE', *, *, #5663, .F. ) ;
#17896=VERTEX_POINT ( 'NONE', #24716 ) ;
#17901=CARTESIAN_POINT ( 'NONE',  ( 24.61381495443087175, 14.36755986787189521, 3.957524335000017768 ) ) ;
#17915=CARTESIAN_POINT ( 'NONE',  ( -28.35945636591989683, -7.983396444576476902, 1.000000000000000888 ) ) ;
#17918=CARTESIAN_POINT ( 'NONE',  ( 18.34691755833856064, 20.56908522341882417, -0.5592437529999827461 ) ) ;
#17928=EDGE_CURVE ( 'NONE', #18728, #17781, #693, .T. ) ;
#17929=ORIENTED_EDGE ( 'NONE', *, *, #30863, .F. ) ;
#17935=ORIENTED_EDGE ( 'NONE', *, *, #22699, .F. ) ;
#17936=CARTESIAN_POINT ( 'NONE',  ( -17.36983091266188950, 10.02891580965362017, -0.6999999999999784173 ) ) ;
#17941=CARTESIAN_POINT ( 'NONE',  ( -17.62526668112344908, -8.236461616547455122, -0.6999999989999727834 ) ) ;
#17942=CARTESIAN_POINT ( 'NONE',  ( -0.6094664100040195764, -28.49364619262437870, 5.104049977999985721 ) ) ;
#17976=CARTESIAN_POINT ( 'NONE',  ( -24.52721838136531574, 14.51532614515681097, 4.239732039000021047 ) ) ;
#17977=AXIS2_PLACEMENT_3D ( 'NONE', #6676, #9038, #21471 ) ;
#17981=CARTESIAN_POINT ( 'NONE',  ( 0.6657531355379500138, -28.49283337230381008, 6.099998581000005693 ) ) ;
#17982=CARTESIAN_POINT ( 'NONE',  ( -27.37939150969657121, 4.212099059672701706, -0.6577119969999878357 ) ) ;
#17989=CARTESIAN_POINT ( 'NONE',  ( 24.37821946547973084, -14.76389286113969490, 4.791564337000009388 ) ) ;
#17991=VERTEX_POINT ( 'NONE', #1583 ) ;
#17995=CARTESIAN_POINT ( 'NONE',  ( 18.50495734115402513, 20.74627095469091742, 0.9999999989999952543 ) ) ;
#18005=ADVANCED_FACE ( 'NONE', ( #18078 ), #1268, .F. ) ;
#18019=CARTESIAN_POINT ( 'NONE',  ( 23.45614981985238146, -19.98580328777019943, 0.7069253189999902265 ) ) ;
#18023=CARTESIAN_POINT ( 'NONE',  ( -27.05781272067678600, 9.945516928293280046, 8.000000000000007105 ) ) ;
#18032=ADVANCED_FACE ( 'NONE', ( #10555 ), #24464, .F. ) ;
#18059=CARTESIAN_POINT ( 'NONE',  ( -17.93256772572758351, -9.057264202608372727, 0.000000000000000000 ) ) ;
#18073=CARTESIAN_POINT ( 'NONE',  ( 16.62864107198832642, 10.02943855701489895, -0.000000000000000000 ) ) ;
#18074=CARTESIAN_POINT ( 'NONE',  ( 18.22456968101094077, 20.00000017576654443, -0.6880465830000070948 ) ) ;
#18075=CARTESIAN_POINT ( 'NONE',  ( 14.60916111670818474, -28.04296597385482315, 8.000000000000007105 ) ) ;
#18076=CARTESIAN_POINT ( 'NONE',  ( 27.79539923781684507, 0.5057481689249125889, 8.000000000000007105 ) ) ;
#18078=FACE_OUTER_BOUND ( 'NONE', #16663, .T. ) ;
#18098=EDGE_CURVE ( 'NONE', #6771, #8375, #10370, .T. ) ;
#18100=CARTESIAN_POINT ( 'NONE',  ( -7.224034581361331309E-06, 19.99999999982847498, 0.000000000000000000 ) ) ;
#18103=CARTESIAN_POINT ( 'NONE',  ( -24.35799198229911866, 13.39970082454098232, 6.098655031999994591 ) ) ;
#18117=CARTESIAN_POINT ( 'NONE',  ( -20.30403093138962234, 20.00000000003553424, 1.000000000000000888 ) ) ;
#18124=VERTEX_POINT ( 'NONE', #8962 ) ;
#18146=CYLINDRICAL_SURFACE ( 'NONE', #5991, 1.100000000000002309 ) ;
#18148=CARTESIAN_POINT ( 'NONE',  ( -25.16696685483287155, 13.37570800105703306, 3.997190761000024573 ) ) ;
#18150=B_SPLINE_CURVE_WITH_KNOTS ( 'NONE', 3,
 ( #7003, #4337, #19113, #30924, #16589, #16281 ),
 .UNSPECIFIED., .F., .F.,
 ( 4, 2, 4 ),
 ( 0.000000000000000000, 0.5000000000000000000, 1.000000000000000000 ),
 .UNSPECIFIED. ) ;
#18158=CARTESIAN_POINT ( 'NONE',  ( -23.55444264242456498, 16.04540112444970390, 8.000000000000007105 ) ) ;
#18159=CARTESIAN_POINT ( 'NONE',  ( 18.03439872975474145, 20.21871556473540110, 0.02487532100001188518 ) ) ;
#18163=CARTESIAN_POINT ( 'NONE',  ( -23.23277126416379801, -15.26692729116844482, 5.104183903000020450 ) ) ;
#18164=CARTESIAN_POINT ( 'NONE',  ( 17.16657240419154462, 10.99999999996915179, -0.6999999999999784173 ) ) ;
#18167=CARTESIAN_POINT ( 'NONE',  ( 23.88992819277635959, -14.21747995518237317, 4.319167818000013703 ) ) ;
#18173=CARTESIAN_POINT ( 'NONE',  ( -23.77308074864635401, 14.41182440788991848, 5.146095667219259262 ) ) ;
#18180=CARTESIAN_POINT ( 'NONE',  ( -27.08859402333795430, -0.4928875713624353283, 0.02487529600000981667 ) ) ;
#18188=CARTESIAN_POINT ( 'NONE',  ( 23.81776757409229361, 15.65134803726813217, 4.999998581000003384 ) ) ;
#18192=CARTESIAN_POINT ( 'NONE',  ( -28.49528339128749366, -0.5184828350247797646, 1.000000000000000888 ) ) ;
#18196=B_SPLINE_CURVE_WITH_KNOTS ( 'NONE', 3,
 ( #948, #23126, #5806, #1251, #1565, #27665, #5650, #13039, #29876, #3761, #10536, #20133 ),
 .UNSPECIFIED., .F., .F.,
 ( 4, 2, 2, 2, 2, 4 ),
 ( 0.000000000000000000, 0.2499999999999997780, 0.4999999999999995559, 0.6250000000000000000, 0.7500000000000004441, 1.000000000000000000 ),
 .UNSPECIFIED. ) ;
#18199=CARTESIAN_POINT ( 'NONE',  ( -24.83827471527357744, 12.48687850854618198, 4.999998581000003384 ) ) ;
#18230=CARTESIAN_POINT ( 'NONE',  ( 27.74223843740156425, -9.623426708017472464, -0.5592437529999827461 ) ) ;
#18231=CARTESIAN_POINT ( 'NONE',  ( -18.92328505709462405, 19.72870074452574940, 0.1493323239999955199 ) ) ;
#18232=CARTESIAN_POINT ( 'NONE',  ( 18.81999291203268854, -20.80334143950547698, 8.000000000000007105 ) ) ;
#18234=CARTESIAN_POINT ( 'NONE',  ( 21.52822896111007367, 17.37722137477383910, -0.6577119969999878357 ) ) ;
#18236=CARTESIAN_POINT ( 'NONE',  ( 0.4368970292349217965, -27.79681690464249044, 3.901345920999998995 ) ) ;
#18241=CARTESIAN_POINT ( 'NONE',  ( 24.21906834310036771, 15.02342240524378703, 6.042470792000015578 ) ) ;
#18261=CARTESIAN_POINT ( 'NONE',  ( -0.5968465743326634154, -28.49391676915515603, 5.208100973000007627 ) ) ;
#18266=EDGE_LOOP ( 'NONE', ( #2904, #23937, #2896, #21719 ) ) ;
#18272=B_SPLINE_CURVE_WITH_KNOTS ( 'NONE', 5,
 ( #21870, #19501, #9424, #26271, #21402, #2206, #14474, #19185, #19347, #14160, #28772, #4711, #28938, #11796, #22023 ),
 .UNSPECIFIED., .F., .F.,
 ( 6, 3, 3, 3, 6 ),
 ( 0.000000000000000000, 0.1000000000005725753, 0.4000000000022904123, 0.6999999999994271915, 1.000000000000000000 ),
 .UNSPECIFIED. ) ;
#18290=VERTEX_POINT ( 'NONE', #15384 ) ;
#18304=EDGE_LOOP ( 'NONE', ( #17929, #15239, #24035, #29183 ) ) ;
#18305=CARTESIAN_POINT ( 'NONE',  ( 24.60726958095619565, -14.37955347759689317, 5.901399682999991292 ) ) ;
#18314=CARTESIAN_POINT ( 'NONE',  ( 23.47715715144835613, -20.00370206646645599, 8.000000000000007105 ) ) ;
#18320=CARTESIAN_POINT ( 'NONE',  ( -28.35455043824866550, -0.5159221438580913199, 0.2374258030000131470 ) ) ;
#18326=CARTESIAN_POINT ( 'NONE',  ( 26.65905076765696791, 9.650916058398387065, 0.7069222140000108734 ) ) ;
#18332=ORIENTED_EDGE ( 'NONE', *, *, #21982, .F. ) ;
#18338=CARTESIAN_POINT ( 'NONE',  ( -3.040504020835836041, -1.733590291693717145, -0.6999999999999784173 ) ) ;
#18350=ADVANCED_FACE ( 'NONE', ( #19955 ), #22476, .F. ) ;
#18351=CARTESIAN_POINT ( 'NONE',  ( -27.77052805885580966, -0.5052956280425512370, 0.7069222069999991920 ) ) ;
#18355=B_SPLINE_CURVE_WITH_KNOTS ( 'NONE', 3,
 ( #8227, #27138, #8385, #22261, #17832, #29488 ),
 .UNSPECIFIED., .F., .F.,
 ( 4, 2, 4 ),
 ( 0.000000000000000000, 0.5000000000000000000, 1.000000000000000000 ),
 .UNSPECIFIED. ) ;
#18365=DIRECTION ( 'NONE',  ( -1.000000000000000000, -1.771497531999344233E-11, 0.000000000000000000 ) ) ;
#18371=DIRECTION ( 'NONE',  ( 0.000000000000000000, 0.000000000000000000, -1.000000000000000000 ) ) ;
#18402=CARTESIAN_POINT ( 'NONE',  ( 8.522909508489858510, -26.72774706475087569, 8.000000000000007105 ) ) ;
#18404=CARTESIAN_POINT ( 'NONE',  ( 22.36497543530602172, 18.05262891234276168, 0.2374258030000131470 ) ) ;
#18448=EDGE_CURVE ( 'NONE', #25327, #974, #4021, .T. ) ;
#18458=CARTESIAN_POINT ( 'NONE',  ( -16.85343921402336775, -7.900182044543379689, -0.6999999999999784173 ) ) ;
#18460=CARTESIAN_POINT ( 'NONE',  ( 24.37165445055180157, -14.77472140295711434, 4.999998581000003384 ) ) ;
#18480=CARTESIAN_POINT ( 'NONE',  ( 27.16228374367956988, 4.990250640343800725, 0.08279779300002232389 ) ) ;
#18488=CARTESIAN_POINT ( 'NONE',  ( 24.60726958085803417, -14.37955347769869263, 4.098597479000015475 ) ) ;
#18494=B_SPLINE_CURVE_WITH_KNOTS ( 'NONE', 1,
 ( #28757, #16493 ),
 .UNSPECIFIED., .F., .F.,
 ( 2, 2 ),
 ( -0.7000000000189999794, 2.331468351712828735E-15 ),
 .UNSPECIFIED. ) ;
#18503=ORIENTED_EDGE ( 'NONE', *, *, #14700, .T. ) ;
#18508=CARTESIAN_POINT ( 'NONE',  ( -3.361572482953519625, -1.073845131765873484, 0.000000000000000000 ) ) ;
#18509=CARTESIAN_POINT ( 'NONE',  ( -0.3682501489830092845, -27.79783598715961901, 4.319846982000025370 ) ) ;
#18515=CARTESIAN_POINT ( 'NONE',  ( 26.11035454923439403, 9.897950727584628794, 8.000000000000007105 ) ) ;
#18521=CARTESIAN_POINT ( 'NONE',  ( 23.23277120355932723, 15.26692725134781625, 4.854156652956985951 ) ) ;
#18528=CARTESIAN_POINT ( 'NONE',  ( -16.95798644146054812, 9.897551528143511135, 0.000000000000000000 ) ) ;
#18539=EDGE_LOOP ( 'NONE', ( #9440, #29868, #16908, #2416, #24304, #19250, #23466, #27118 ) ) ;
#18545=CARTESIAN_POINT ( 'NONE',  ( -16.17397428881745469, -8.107840965152638191, -0.6999999999999783062 ) ) ;
#18548=ADVANCED_BREP_SHAPE_REPRESENTATION ( '', ( #72, #17722 ), #16292 ) ;
#18558=CARTESIAN_POINT ( 'NONE',  ( -27.77990052619939476, -1.357541420128717702, 8.000000000000007105 ) ) ;
#18561=CARTESIAN_POINT ( 'NONE',  ( 26.71513120331102797, 4.908099852724521206, -0.6999999999999784173 ) ) ;
#18563=CARTESIAN_POINT ( 'NONE',  ( -17.72521362118247623, 11.65988689034122316, -4.336808689942018722E-16 ) ) ;
#18593=CARTESIAN_POINT ( 'NONE',  ( 0.000000000000000000, 0.000000000000000000, 0.000000000000000000 ) ) ;
#18595=CARTESIAN_POINT ( 'NONE',  ( -25.20441737622035205, 13.30520055017012204, 5.965619087901981921 ) ) ;
#18598=CARTESIAN_POINT ( 'NONE',  ( 23.77307027441306531, -14.41181805765238444, 4.999998581000003384 ) ) ;
#18599=CARTESIAN_POINT ( 'NONE',  ( 0.5184513693225644149, -28.49550581263314086, 6.099998581000020792 ) ) ;
#18601=ORIENTED_EDGE ( 'NONE', *, *, #16488, .T. ) ;
#18612=VERTEX_POINT ( 'NONE', #27371 ) ;
#18623=DIRECTION ( 'NONE',  ( 0.6941258031311203780, 0.7198537139083029945, 0.000000000000000000 ) ) ;
#18626=CARTESIAN_POINT ( 'NONE',  ( -19.31846164438172053, 19.99998910362869964, -0.3730415779728155634 ) ) ;
#18658=CARTESIAN_POINT ( 'NONE',  ( -16.04158851046123502, 10.23646161653652875, -0.6999999999999784173 ) ) ;
#18667=CARTESIAN_POINT ( 'NONE',  ( -15.97608884582789734, -9.690347176502019266, 0.000000000000000000 ) ) ;
#18669=CARTESIAN_POINT ( 'NONE',  ( 20.97486217528226149, 18.32139343332559989, 4.666666666666781538 ) ) ;
#18698=CARTESIAN_POINT ( 'NONE',  ( -27.24406355354269849, -0.4957164003159654775, 0.08279779300002232389 ) ) ;
#18702=VERTEX_POINT ( 'NONE', #14465 ) ;
#18708=CARTESIAN_POINT ( 'NONE',  ( 27.21667690494597380, -9.441116152978883846, -0.6999999999999784173 ) ) ;
#18710=CARTESIAN_POINT ( 'NONE',  ( 26.38956582071493528, -11.43351142516159058, 8.000000000000007105 ) ) ;
#18712=B_SPLINE_SURFACE_WITH_KNOTS ( 'NONE', 5, 1, ( 
 ( #2228, #14802 ),
 ( #14652, #26752 ),
 ( #14498, #24094 ),
 ( #17001, #26913 ),
 ( #2834, #26604 ),
 ( #29112, #9763 ),
 ( #9610, #5043 ),
 ( #21425, #179 ),
 ( #12429, #26293 ),
 ( #19209, #24237 ),
 ( #28793, #7251 ),
 ( #16683, #28959 ),
 ( #2533, #22046 ),
 ( #2682, #21894 ),
 ( #9924, #12120 ) ),
 .UNSPECIFIED., .F., .F., .F.,
 ( 6, 3, 3, 3, 6 ),
 ( 2, 2 ),
 ( 0.000000000000000000, 0.5239055191900000574, 1.047811038380000115, 1.571716557570000061, 1.746351730630000043 ),
 ( -0.7000000000009999335, 2.557307477669999647E-06 ),
 .UNSPECIFIED. ) ;
#18713=CARTESIAN_POINT ( 'NONE',  ( 26.20132165689940962, 9.485175511428851181, -0.6577119969999878357 ) ) ;
#18728=VERTEX_POINT ( 'NONE', #21229 ) ;
#18731=CARTESIAN_POINT ( 'NONE',  ( 23.81776757409229361, 15.65134803726813217, 4.895813257000003915 ) ) ;
#18732=CARTESIAN_POINT ( 'NONE',  ( -24.40022624598054435, -14.72688605908970239, 3.899998581000013509 ) ) ;
#18734=ADVANCED_FACE ( 'NONE', ( #2649 ), #2655, .F. ) ;
#18752=CARTESIAN_POINT ( 'NONE',  ( 0.5890437901237028928, -28.49417040867362516, 6.098651075000017130 ) ) ;
#18753=CARTESIAN_POINT ( 'NONE',  ( -17.91041692047024370, 11.26717219323752062, -0.6999999999999784173 ) ) ;
#18754=EDGE_LOOP ( 'NONE', ( #8846, #30710, #29874, #16242 ) ) ;
#18763=VERTEX_POINT ( 'NONE', #2808 ) ;
#18764=EDGE_LOOP ( 'NONE', ( #7082, #28132, #15054, #9989 ) ) ;
#18775=CARTESIAN_POINT ( 'NONE',  ( 17.16657240421717390, -9.000000000001264766, -0.6999999999999784173 ) ) ;
#18778=CARTESIAN_POINT ( 'NONE',  ( -18.58704431631444010, 19.99991904899251338, -0.6240947616942604803 ) ) ;
#18808=CARTESIAN_POINT ( 'NONE',  ( -26.93696268452645981, -0.4901285798020263984, 0.000000000000000000 ) ) ;
#18832=CARTESIAN_POINT ( 'NONE',  ( -25.16696685483287155, 13.37570800105703306, 3.997190761000024573 ) ) ;
#18835=CARTESIAN_POINT ( 'NONE',  ( 24.83827260360999389, -12.48687744688666967, 4.999998581000003384 ) ) ;
#18837=CARTESIAN_POINT ( 'NONE',  ( -16.81341597756113515, 9.900182044522454206, -1.000005633855494125E-09 ) ) ;
#18846=COLOUR_RGB ( '', 0.09019608, 0.27058824, 0.51372549) ;
#18855=CARTESIAN_POINT ( 'NONE',  ( -25.38146355688813216, 12.59839640969179975, 2.400000000000013234 ) ) ;
#18858=CARTESIAN_POINT ( 'NONE',  ( -25.14597776469364732, -15.02549348228339454, 8.000000000000007105 ) ) ;
#18859=CARTESIAN_POINT ( 'NONE',  ( -16.06988921231594603, 11.79183908526949054, 0.000000000000000000 ) ) ;
#18863=FACE_OUTER_BOUND ( 'NONE', #20106, .T. ) ;
#18866=CARTESIAN_POINT ( 'NONE',  ( 24.31044119090657318, 13.69178363021313949, 8.000000000000007105 ) ) ;
#18867=CARTESIAN_POINT ( 'NONE',  ( 24.83827260360999389, -12.48687744688666967, 4.999998581000003384 ) ) ;
#18868=CARTESIAN_POINT ( 'NONE',  ( 22.63260994176697238, -19.28417101125922883, -0.6999999999999784173 ) ) ;
#18872=B_SPLINE_CURVE_WITH_KNOTS ( 'NONE', 1,
 ( #30488, #28423 ),
 .UNSPECIFIED., .F., .F.,
 ( 2, 2 ),
 ( -0.7017616274569999923, 4.107825191113079200E-15 ),
 .UNSPECIFIED. ) ;
#18878=CARTESIAN_POINT ( 'NONE',  ( -24.83827471527357744, 12.48687850854618198, 4.999998581000003384 ) ) ;
#18890=B_SPLINE_CURVE_WITH_KNOTS ( 'NONE', 3,
 ( #16544, #4125, #30568, #18595, #6949, #14193, #23796, #6635, #2243, #8676, #16233, #9779 ),
 .UNSPECIFIED., .F., .F.,
 ( 4, 2, 2, 2, 2, 4 ),
 ( 0.000000000000000000, 0.2500000000000008882, 0.5000000000000017764, 0.6250000000000016653, 0.7500000000000015543, 1.000000000000000000 ),
 .UNSPECIFIED. ) ;
#18894=CARTESIAN_POINT ( 'NONE',  ( 27.98121187870611593, -9.706323496128696604, 1.000000000000000888 ) ) ;
#18897=CARTESIAN_POINT ( 'NONE',  ( 19.98778790343742529, 20.00007856030388353, 0.1551495369530143942 ) ) ;
#18900=CARTESIAN_POINT ( 'NONE',  ( 17.85846454799866834, -9.867189877967701861, -4.336808689942017736E-16 ) ) ;
#18908=CARTESIAN_POINT ( 'NONE',  ( -20.30403093128963476, 20.00000000003735323, 3.000000106999994642 ) ) ;
#18913=CARTESIAN_POINT ( 'NONE',  ( -24.37165444408190851, 14.77472139917419369, 4.999998581000003384 ) ) ;
#18918=ORIENTED_EDGE ( 'NONE', *, *, #16401, .F. ) ;
#18936=CARTESIAN_POINT ( 'NONE',  ( -20.28349499515899268, 20.00041701855139564, 0.7434420671224396537 ) ) ;
#18942=CARTESIAN_POINT ( 'NONE',  ( -23.23277431135011994, -15.26692929364048013, 4.853020674800981205 ) ) ;
#18943=CARTESIAN_POINT ( 'NONE',  ( 0.7646642646963620615, -28.49022165133369455, 3.920206710000012862 ) ) ;
#18945=B_SPLINE_CURVE_WITH_KNOTS ( 'NONE', 3,
 ( #4554, #21866, #10054, #19181, #24212, #4706 ),
 .UNSPECIFIED., .F., .F.,
 ( 4, 2, 4 ),
 ( 0.000000000000000000, 0.5000000000000000000, 1.000000000000000000 ),
 .UNSPECIFIED. ) ;
#18964=CARTESIAN_POINT ( 'NONE',  ( 1.568292632099254291, -27.75603058367145692, 4.689797669000017599 ) ) ;
#18981=CARTESIAN_POINT ( 'NONE',  ( -15.82777162301967167, -9.463291056475755525, 0.000000000000000000 ) ) ;
#18991=CARTESIAN_POINT ( 'NONE',  ( -16.46626780658883504, -7.955406060106740895, 0.000000000000000000 ) ) ;
#18992=CARTESIAN_POINT ( 'NONE',  ( 24.45473033137484720, 14.63622297804190175, 6.098654221000004760 ) ) ;
#19000=AXIS2_PLACEMENT_3D ( 'NONE', #8541, #15022, #12811 ) ;
#19017=CARTESIAN_POINT ( 'NONE',  ( -16.83342759575507586, 10.99999999997565503, -0.6999999999999784173 ) ) ;
#19048=CARTESIAN_POINT ( 'NONE',  ( 23.94466869970572986, 15.45669658583985751, 4.319305385000027364 ) ) ;
#19051=B_SPLINE_CURVE_WITH_KNOTS ( 'NONE', 3,
 ( #9205, #11581, #4031, #23859, #13628, #21028, #30629, #1674, #7013, #13943, #4501, #23704 ),
 .UNSPECIFIED., .F., .F.,
 ( 4, 2, 2, 2, 2, 4 ),
 ( 0.000000000000000000, 0.2499999999999984457, 0.4999999999999968914, 0.6249999999999976685, 0.7499999999999984457, 1.000000000000000000 ),
 .UNSPECIFIED. ) ;
#19052=CARTESIAN_POINT ( 'NONE',  ( 19.32427370919018017, 20.00008879814301466, -0.3673419808590195901 ) ) ;
#19064=CARTESIAN_POINT ( 'NONE',  ( -17.40631048005291959, 11.95034962824490066, -0.6999999999999784173 ) ) ;
#19069=CARTESIAN_POINT ( 'NONE',  ( 1.379247882482921517, -27.76613141686462782, 5.680166690000016061 ) ) ;
#19070=CARTESIAN_POINT ( 'NONE',  ( 16.37473331889771089, 11.76353838340827984, 0.000000000000000000 ) ) ;
#19098=EDGE_CURVE ( 'NONE', #28870, #13182, #13710, .T. ) ;
#19113=CARTESIAN_POINT ( 'NONE',  ( 16.21564467616125071, -9.571375077537407350, -0.6999999999999785283 ) ) ;
#19115=CARTESIAN_POINT ( 'NONE',  ( -27.02151979721923780, 4.157043372987225816, 0.000000000000000000 ) ) ;
#19129=CARTESIAN_POINT ( 'NONE',  ( -24.16679028379773797, -15.10730798416152609, 3.997250019000003540 ) ) ;
#19134=EDGE_CURVE ( 'NONE', #17637, #7280, #4680, .T. ) ;
#19139=CARTESIAN_POINT ( 'NONE',  ( 21.81247352487541136, 17.27884107588915796, 6.000000000000005329 ) ) ;
#19146=CARTESIAN_POINT ( 'NONE',  ( -25.25401215124432852, 13.21081861195569296, 4.098596794000014754 ) ) ;
#19147=FACE_OUTER_BOUND ( 'NONE', #12755, .T. ) ;
#19171=CARTESIAN_POINT ( 'NONE',  ( -25.14597776469910428, -15.02549348198344603, 1.000000000000000888 ) ) ;
#19181=CARTESIAN_POINT ( 'NONE',  ( -15.88307796653755055, 11.57288288501910856, -0.6999999999999784173 ) ) ;
#19185=CARTESIAN_POINT ( 'NONE',  ( -24.75645986059670278, -14.12045945564184279, 5.901294544000013076 ) ) ;
#19187=EDGE_CURVE ( 'NONE', #16332, #12633, #17234, .T. ) ;
#19195=CARTESIAN_POINT ( 'NONE',  ( 24.32472894995379420, -13.45989151107506387, 3.899998581000013509 ) ) ;
#19205=CYLINDRICAL_SURFACE ( 'NONE', #16484, 1.100000000000002309 ) ;
#19207=CARTESIAN_POINT ( 'NONE',  ( 18.61284099291034266, 19.99999152564625859, -0.6181686921151241521 ) ) ;
#19209=CARTESIAN_POINT ( 'NONE',  ( -24.74993094845043018, 14.13250375615880117, 6.042507811999997536 ) ) ;
#19219=CARTESIAN_POINT ( 'NONE',  ( 19.90458219140913343, 19.99999992531521187, 0.04954396799999871703 ) ) ;
#19222=CARTESIAN_POINT ( 'NONE',  ( 23.99475407440551322, -14.04003783131165228, 5.886818977337623160 ) ) ;
#19224=CARTESIAN_POINT ( 'NONE',  ( -23.83639842770461570, -14.30623133119355828, 3.899998581000013509 ) ) ;
#19246=CARTESIAN_POINT ( 'NONE',  ( 19.06888577842656574, 19.69230313816537148, 0.2004941630000256492 ) ) ;
#19248=EDGE_CURVE ( 'NONE', #10592, #5736, #21237, .T. ) ;
#19250=ORIENTED_EDGE ( 'NONE', *, *, #5031, .T. ) ;
#19258=CARTESIAN_POINT ( 'NONE',  ( 16.06937396351131397, 10.83602254743009219, -0.6999999999999784173 ) ) ;
#19261=ADVANCED_FACE ( 'NONE', ( #3533 ), #19497, .T. ) ;
#19277=DIRECTION ( 'NONE',  ( 0.000000000000000000, 0.000000000000000000, -1.000000000000000000 ) ) ;
#19278=CARTESIAN_POINT ( 'NONE',  ( 0.5057536231481327693, -27.79562098839016571, 3.899998581000013509 ) ) ;
#19293=FACE_OUTER_BOUND ( 'NONE', #27239, .T. ) ;
#19325=VERTEX_POINT ( 'NONE', #10092 ) ;
#19327=CARTESIAN_POINT ( 'NONE',  ( -16.14314806291716664, -9.868837085557133904, -0.6999999999999784173 ) ) ;
#19332=CARTESIAN_POINT ( 'NONE',  ( 27.79539923781684507, 0.5057481689249235801, 8.000000000000007105 ) ) ;
#19347=CARTESIAN_POINT ( 'NONE',  ( -24.83401023410007724, -13.98326748972919553, 5.760125276000005456 ) ) ;
#19355=CARTESIAN_POINT ( 'NONE',  ( 25.46368747440213198, -12.80129684534102807, 4.895780544000027490 ) ) ;
#19364=DIRECTION ( 'NONE',  ( 0.000000000000000000, 0.000000000000000000, -1.000000000000000000 ) ) ;
#19368=CARTESIAN_POINT ( 'NONE',  ( 20.30396079695160694, 19.99999999996773425, 0.7422851442966436064 ) ) ;
#19379=CARTESIAN_POINT ( 'NONE',  ( 24.25742563242670613, 13.58028021435546684, 5.680679506000013923 ) ) ;
#19384=CARTESIAN_POINT ( 'NONE',  ( 1.592882851206511186, -27.75460863273100998, 5.208113774000016960 ) ) ;
#19387=VERTEX_POINT ( 'NONE', #15418 ) ;
#19390=B_SPLINE_CURVE_WITH_KNOTS ( 'NONE', 1,
 ( #15519, #18188 ),
 .UNSPECIFIED., .F., .F.,
 ( 2, 2 ),
 ( -2.555885125540000124E-06, 0.7000000000009999335 ),
 .UNSPECIFIED. ) ;
#19397=ORIENTED_EDGE ( 'NONE', *, *, #4045, .T. ) ;
#19399=EDGE_CURVE ( 'NONE', #19859, #16829, #13312, .T. ) ;
#19403=CARTESIAN_POINT ( 'NONE',  ( -25.41286868645085661, 12.90211872727317655, 5.507123707999994622 ) ) ;
#19409=CARTESIAN_POINT ( 'NONE',  ( -23.55444264242456498, 16.04540112444970390, 8.000000000000007105 ) ) ;
#19414=CARTESIAN_POINT ( 'NONE',  ( 0.5401834767574382745, -27.79499634052776358, 3.899998581000013509 ) ) ;
#19423=FACE_OUTER_BOUND ( 'NONE', #27361, .T. ) ;
#19429=FILL_AREA_STYLE_COLOUR ( '', #2732 ) ;
#19432=CARTESIAN_POINT ( 'NONE',  ( 0.5746121234323043891, -27.79431838510023667, 3.901346086000012647 ) ) ;
#19436=ADVANCED_FACE ( 'NONE', ( #3148 ), #20147, .F. ) ;
#19442=B_SPLINE_CURVE_WITH_KNOTS ( 'NONE', 3,
 ( #20009, #29607, #8038, #10571, #20166, #13222 ),
 .UNSPECIFIED., .F., .F.,
 ( 4, 2, 4 ),
 ( 0.000000000000000000, 0.5000000000000000000, 1.000000000000000000 ),
 .UNSPECIFIED. ) ;
#19447=CARTESIAN_POINT ( 'NONE',  ( -15.94164157046648533, 10.34011310946611495, -1.384526174263989415E-13 ) ) ;
#19448=CARTESIAN_POINT ( 'NONE',  ( -24.97472003774791816, -13.73006752753317450, 5.208359076000035337 ) ) ;
#19451=CARTESIAN_POINT ( 'NONE',  ( -24.25792036986074507, -13.57958751026097310, 4.317733944950783886 ) ) ;
#19454=CARTESIAN_POINT ( 'NONE',  ( -20.67339670645382199, -21.57700477944339923, 0.2374258030000131470 ) ) ;
#19456=CARTESIAN_POINT ( 'NONE',  ( 24.06826093661917554, -20.50742065831276051, 8.000000000000007105 ) ) ;
#19463=CARTESIAN_POINT ( 'NONE',  ( 24.98081130624543889, 13.71897605842228529, 5.104178997000024864 ) ) ;
#19466=CARTESIAN_POINT ( 'NONE',  ( 20.30396079662882158, 20.00000000004802203, 3.000000000000002665 ) ) ;
#19478=CARTESIAN_POINT ( 'NONE',  ( -23.88992818679365371, 14.21747995069046588, 4.319167817000008291 ) ) ;
#19484=CARTESIAN_POINT ( 'NONE',  ( -19.80535357377644701, 19.50875577052588739, 2.600000085000026218 ) ) ;
#19487=ORIENTED_EDGE ( 'NONE', *, *, #16873, .T. ) ;
#19490=ADVANCED_FACE ( 'NONE', ( #8479 ), #29030, .F. ) ;
#19492=CARTESIAN_POINT ( 'NONE',  ( 23.55411374389282386, 16.04538543799059980, 8.000000000000007105 ) ) ;
#19497=B_SPLINE_SURFACE_WITH_KNOTS ( 'NONE', 5, 5, ( 
 ( #10622, #8719, #18159, #8396, #1504, #25258, #11096, #1342, #17995 ),
 ( #8559, #20691, #1033, #20217, #3690, #27764, #13129, #23214, #15496 ),
 ( #22737, #5889, #29809, #30288, #6050, #30130, #6208, #1184, #13291 ),
 ( #8244, #25733, #17843, #25575, #13761, #22902, #18326, #10779, #27930 ),
 ( #11248, #4169, #15968, #18480, #20376, #4011, #10936, #13608, #27607 ),
 ( #1657, #15816, #30455, #8877, #28079, #25424, #27448, #25100, #29967 ) ),
 .UNSPECIFIED., .F., .F., .F.,
 ( 6, 6 ),
 ( 6, 3, 6 ),
 ( 65.40639850639999509, 88.32365686489998780 ),
 ( 8.011061266649999624, 8.811526687440000671, 9.611992108220000830 ),
 .UNSPECIFIED. ) ;
#19501=CARTESIAN_POINT ( 'NONE',  ( -24.43659368756648576, -14.66646236829179450, 6.099998581000020792 ) ) ;
#19515=ORIENTED_EDGE ( 'NONE', *, *, #9865, .F. ) ;
#19518=CYLINDRICAL_SURFACE ( 'NONE', #2013, 1.099999999999999867 ) ;
#19530=CARTESIAN_POINT ( 'NONE',  ( 2.611298560087381038, -2.373819477306434500, 0.000000000000000000 ) ) ;
#19545=CARTESIAN_POINT ( 'NONE',  ( 1.413941964909729787, -28.46527362969750996, 4.319830470999985295 ) ) ;
#19550=ORIENTED_EDGE ( 'NONE', *, *, #19593, .T. ) ;
#19578=ORIENTED_EDGE ( 'NONE', *, *, #9259, .T. ) ;
#19581=CARTESIAN_POINT ( 'NONE',  ( -24.45655680962239842, 13.35232502611413707, 0.08279996400001321533 ) ) ;
#19593=EDGE_CURVE ( 'NONE', #28672, #5339, #20445, .T. ) ;
#19606=CARTESIAN_POINT ( 'NONE',  ( -23.47637529058820860, -14.89020704899713365, 5.901296963999991263 ) ) ;
#19608=CARTESIAN_POINT ( 'NONE',  ( -24.15671119056922933, -13.75882116471486682, 4.114296042299178779 ) ) ;
#19611=CARTESIAN_POINT ( 'NONE',  ( -24.93121705008275413, -14.89716849126640952, -0.5592437529999827461 ) ) ;
#19617=CARTESIAN_POINT ( 'NONE',  ( 24.54452541844319668, 14.48555669908156851, 6.079852602000002548 ) ) ;
#19619=FACE_OUTER_BOUND ( 'NONE', #31038, .T. ) ;
#19624=EDGE_LOOP ( 'NONE', ( #28050, #15940, #13507, #13385 ) ) ;
#19629=ORIENTED_EDGE ( 'NONE', *, *, #24734, .F. ) ;
#19631=CARTESIAN_POINT ( 'NONE',  ( -24.60726957497166367, 14.37955347300500364, 4.098597478000010064 ) ) ;
#19635=CARTESIAN_POINT ( 'NONE',  ( -20.30403093128963476, 20.00000000003735323, 2.600000085000026218 ) ) ;
#19642=EDGE_CURVE ( 'NONE', #2704, #10752, #18945, .T. ) ;
#19656=CYLINDRICAL_SURFACE ( 'NONE', #5714, 1.099999999999999867 ) ;
#19661=CARTESIAN_POINT ( 'NONE',  ( 25.16696686177720821, -13.37570800343109312, 3.997190761000024573 ) ) ;
#19663=VERTEX_POINT ( 'NONE', #14155 ) ;
#19683=CARTESIAN_POINT ( 'NONE',  ( 24.81746042555073117, -14.01353061617342455, 6.079865098000015067 ) ) ;
#19688=B_SPLINE_SURFACE_WITH_KNOTS ( 'NONE', 5, 5, ( 
 ( #14300, #28755, #7208, #28452, #301, #21217 ),
 ( #4539, #4854, #14453, #9879, #26708, #30973 ),
 ( #5144, #14758, #2032, #24053, #30817, #12081 ),
 ( #21689, #18855, #26102, #14142, #11776, #21382 ),
 ( #7659, #24509, #24357, #5767, #20240, #29689 ),
 ( #10648, #14915, #22000, #756, #29838, #7968 ) ),
 .UNSPECIFIED., .F., .F., .F.,
 ( 6, 6 ),
 ( 6, 6 ),
 ( 0.000000000000000000, 22.42544452799999988 ),
 ( -3.500000000000000000, 3.500000000000000000 ),
 .UNSPECIFIED. ) ;
#19715=ORIENTED_EDGE ( 'NONE', *, *, #30240, .T. ) ;
#19716=CARTESIAN_POINT ( 'NONE',  ( -24.54884434681058991, 13.04717673392247690, 6.002806401000010617 ) ) ;
#19719=DIRECTION ( 'NONE',  ( 0.7198537139083028835, -0.6941258031311204890, 0.000000000000000000 ) ) ;
#19727=CARTESIAN_POINT ( 'NONE',  ( 0.5890437901233029905, -28.49417040867363227, 3.901346086000012647 ) ) ;
#19738=CARTESIAN_POINT ( 'NONE',  ( -18.50495978135909425, 20.74626080782525506, 0.9999999989999952543 ) ) ;
#19744=CARTESIAN_POINT ( 'NONE',  ( 23.90286779624927149, 15.52112777353848294, 5.560535498006014876 ) ) ;
#19745=CARTESIAN_POINT ( 'NONE',  ( -3.040504021322313122, -1.733590290792417887, -0.5999999999999894307 ) ) ;
#19749=CARTESIAN_POINT ( 'NONE',  ( -26.19983009839024035, 8.854867600185624354, -0.6999999999999784173 ) ) ;
#19767=CARTESIAN_POINT ( 'NONE',  ( 13.99313239240532525, -26.86047011600456713, -0.6577119969999878357 ) ) ;
#19769=VECTOR ( 'NONE', #3169, 1000.000000000000000 ) ;
#19775=CARTESIAN_POINT ( 'NONE',  ( -0.3682501489410162088, -27.79783598715885518, 5.680150179000031940 ) ) ;
#19784=ORIENTED_EDGE ( 'NONE', *, *, #25062, .T. ) ;
#19790=CARTESIAN_POINT ( 'NONE',  ( -24.74993094845043018, 14.13250375615880117, 3.957489350000009676 ) ) ;
#19791=CARTESIAN_POINT ( 'NONE',  ( -28.55928429112321609, 2.998940805198770043, 8.000000000000007105 ) ) ;
#19797=VERTEX_POINT ( 'NONE', #17726 ) ;
#19799=CARTESIAN_POINT ( 'NONE',  ( 24.98081130624543889, 13.71897605842228529, 4.895818164000031558 ) ) ;
#19815=ORIENTED_EDGE ( 'NONE', *, *, #23724, .F. ) ;
#19820=CARTESIAN_POINT ( 'NONE',  ( 25.46368747440213198, -12.80129684534102807, 4.999998581000003384 ) ) ;
#19824=EDGE_CURVE ( 'NONE', #18702, #14604, #9922, .T. ) ;
#19831=CARTESIAN_POINT ( 'NONE',  ( 25.80996960090668679, 10.85703805089278617, 1.000000000000000888 ) ) ;
#19845=CARTESIAN_POINT ( 'NONE',  ( 24.37165445055180157, -14.77472140295711434, 5.104215870000011535 ) ) ;
#19846=CARTESIAN_POINT ( 'NONE',  ( 18.31101511981528773, 19.88193408480103486, 0.02162463700000616385 ) ) ;
#19857=CARTESIAN_POINT ( 'NONE',  ( -17.93324555120827668, 10.97998838178171432, -1.000005633855494125E-09 ) ) ;
#19859=VERTEX_POINT ( 'NONE', #3734 ) ;
#19870=CARTESIAN_POINT ( 'NONE',  ( -17.78435532386814799, -9.571375077557558342, -0.6999999999999785283 ) ) ;
#19873=CARTESIAN_POINT ( 'NONE',  ( 17.93011078763067090, 11.79183908526299085, -0.6999999989999727834 ) ) ;
#19874=CARTESIAN_POINT ( 'NONE',  ( -28.49528339128749366, -0.5184828350247797646, 1.000000000000000888 ) ) ;
#19887=EDGE_CURVE ( 'NONE', #11806, #15540, #5786, .T. ) ;
#19907=CARTESIAN_POINT ( 'NONE',  ( -27.07233446881492611, 8.380004974212880597, 1.000000000000000888 ) ) ;
#19909=CARTESIAN_POINT ( 'NONE',  ( 17.00259495252183228, -7.902801559240212548, -4.336808689942018722E-16 ) ) ;
#19914=FACE_OUTER_BOUND ( 'NONE', #29565, .T. ) ;
#19925=CARTESIAN_POINT ( 'NONE',  ( 17.70297572282393617, 11.97108418938390884, 1.385610376436474414E-13 ) ) ;
#19927=CARTESIAN_POINT ( 'NONE',  ( -0.3000709590196222187, -27.79870762326714484, 5.759626916000016195 ) ) ;
#19943=CARTESIAN_POINT ( 'NONE',  ( -25.14597776469364732, -15.02549348228339454, 8.000000000000007105 ) ) ;
#19955=FACE_OUTER_BOUND ( 'NONE', #11645, .T. ) ;
#19966=ORIENTED_EDGE ( 'NONE', *, *, #11254, .T. ) ;
#19973=CARTESIAN_POINT ( 'NONE',  ( -17.78435532361610782, 10.42862492215759573, -0.6999999999999785283 ) ) ;
#19992=CARTESIAN_POINT ( 'NONE',  ( -20.30403093138962234, 20.00000000003553424, 1.000000000000000888 ) ) ;
#20009=CARTESIAN_POINT ( 'NONE',  ( 17.18658402241074867, -10.09981795543446736, -1.000005633855494125E-09 ) ) ;
#20010=ADVANCED_FACE ( 'NONE', ( #19147 ), #16470, .F. ) ;
#20023=LINE ( 'NONE', #13083, #25402 ) ;
#20030=CARTESIAN_POINT ( 'NONE',  ( -2.484315071469220815, 2.507604248379868839, -0.6999999999999783062 ) ) ;
#20039=CARTESIAN_POINT ( 'NONE',  ( -27.39085626545857721, 6.366048368229709098, 8.000000000000007105 ) ) ;
#20045=B_SPLINE_CURVE_WITH_KNOTS ( 'NONE', 5,
 ( #12739, #5658, #24240, #12122, #7403, #9926 ),
 .UNSPECIFIED., .F., .F.,
 ( 6, 6 ),
 ( 0.000000000000000000, 24.33438218110000051 ),
 .UNSPECIFIED. ) ;
#20053=CARTESIAN_POINT ( 'NONE',  ( 1.490216763352725904, -28.46131404266857601, 5.560567654947754512 ) ) ;
#20058=CARTESIAN_POINT ( 'NONE',  ( -16.83342759582943060, -8.999999999996580513, -0.6999999999999784173 ) ) ;
#20064=AXIS2_PLACEMENT_3D ( 'NONE', #18775, #28382, #19719 ) ;
#20065=CARTESIAN_POINT ( 'NONE',  ( 24.90302311548996883, -13.86047864964742793, 3.901342110999989288 ) ) ;
#20070=CARTESIAN_POINT ( 'NONE',  ( -16.04158851046123502, 10.23646161653652875, 0.000000000000000000 ) ) ;
#20071=CARTESIAN_POINT ( 'NONE',  ( -23.83639842780459972, -14.30623133119537727, 6.099998581000020792 ) ) ;
#20073=CARTESIAN_POINT ( 'NONE',  ( -24.34973987568254472, -13.41386311733433878, 4.711897478746439383 ) ) ;
#20076=CARTESIAN_POINT ( 'NONE',  ( 13.86097538755027969, -26.60678858114344436, -0.6999999999999784173 ) ) ;
#20079=CARTESIAN_POINT ( 'NONE',  ( 24.37165445055180157, -14.77472140295711434, 4.895781291000017355 ) ) ;
#20082=CARTESIAN_POINT ( 'NONE',  ( -0.1501630636364793547, -28.50011693320649542, 5.900904413000008120 ) ) ;
#20083=ORIENTED_EDGE ( 'NONE', *, *, #6910, .T. ) ;
#20091=ORIENTED_EDGE ( 'NONE', *, *, #4892, .F. ) ;
#20095=EDGE_CURVE ( 'NONE', #23829, #29063, #1285, .T. ) ;
#20096=CARTESIAN_POINT ( 'NONE',  ( 26.93696268452645626, 0.4901285798022146367, 0.000000000000000000 ) ) ;
#20097=EDGE_CURVE ( 'NONE', #23233, #16332, #2402, .T. ) ;
#20100=CARTESIAN_POINT ( 'NONE',  ( 16.47629287105559115, 11.86883708612923982, -0.6999999999999784173 ) ) ;
#20106=EDGE_LOOP ( 'NONE', ( #20585, #20746, #21993, #30505 ) ) ;
#20108=CARTESIAN_POINT ( 'NONE',  ( 24.43659368183839931, 14.66646236428692340, 3.899998581000013509 ) ) ;
#20121=CARTESIAN_POINT ( 'NONE',  ( -17.49331448452011628, -9.891786026572814805, -0.6999999999999784173 ) ) ;
#20133=CARTESIAN_POINT ( 'NONE',  ( -0.5944614571882205212, -27.79380703160649446, 4.999998581000003384 ) ) ;
#20146=CARTESIAN_POINT ( 'NONE',  ( 28.49528339128749366, 0.5184828350247822071, 1.000000000000000888 ) ) ;
#20147=CYLINDRICAL_SURFACE ( 'NONE', #11150, 1.100000000000002309 ) ;
#20149=DIRECTION ( 'NONE',  ( -0.6941258031311203780, -0.7198537139083029945, 0.000000000000000000 ) ) ;
#20154=CARTESIAN_POINT ( 'NONE',  ( 24.36375418468539067, 14.78716628296302282, 6.095965061000018892 ) ) ;
#20157=ORIENTED_EDGE ( 'NONE', *, *, #2843, .F. ) ;
#20162=EDGE_LOOP ( 'NONE', ( #24254, #6338, #17739, #22006 ) ) ;
#20166=CARTESIAN_POINT ( 'NONE',  ( 16.50835677101655108, -9.893373635889151529, 0.000000000000000000 ) ) ;
#20170=CARTESIAN_POINT ( 'NONE',  ( -0.1501630636364793547, -28.50011693320649542, 5.900904413000008120 ) ) ;
#20182=CARTESIAN_POINT ( 'NONE',  ( 0.5184513693225318853, -28.49550581263314086, 3.899998581000013509 ) ) ;
#20187=CARTESIAN_POINT ( 'NONE',  ( 25.72310959295360533, 9.312057329555777585, 0.000000000000000000 ) ) ;
#20190=CARTESIAN_POINT ( 'NONE',  ( 26.79556473285982321, 0.4875557887249851730, -0.6999999999999784173 ) ) ;
#20192=VERTEX_POINT ( 'NONE', #27937 ) ;
#20198=CARTESIAN_POINT ( 'NONE',  ( -24.60726957497166367, 14.37955347300500364, 4.098597478000010064 ) ) ;
#20200=EDGE_CURVE ( 'NONE', #22866, #3218, #21180, .T. ) ;
#20204=CARTESIAN_POINT ( 'NONE',  ( -21.88061800209681707, 17.41725036080275046, -0.5592437529999827461 ) ) ;
#20205=FACE_OUTER_BOUND ( 'NONE', #24541, .T. ) ;
#20210=CARTESIAN_POINT ( 'NONE',  ( 19.80526555962148549, 19.50877392102342256, 1.000000000000000888 ) ) ;
#20215=CARTESIAN_POINT ( 'NONE',  ( -24.66346748865669625, -14.28208995890502564, 6.002748559000014694 ) ) ;
#20217=CARTESIAN_POINT ( 'NONE',  ( 21.48906533508084138, 17.34561098343697338, 0.08279780700001793114 ) ) ;
#20222=DIRECTION ( 'NONE',  ( 0.000000000000000000, 0.000000000000000000, -1.000000000000000000 ) ) ;
#20226=FACE_OUTER_BOUND ( 'NONE', #21949, .T. ) ;
#20235=VERTEX_POINT ( 'NONE', #4804 ) ;
#20236=CARTESIAN_POINT ( 'NONE',  ( -4.653831783691562585, -30.83989042116281709, 0.5514251240000267451 ) ) ;
#20240=CARTESIAN_POINT ( 'NONE',  ( -22.90527192528401201, 16.36193184990112570, 6.600000000000022737 ) ) ;
#20242=CARTESIAN_POINT ( 'NONE',  ( 24.50348397774029152, -13.13223627703424690, 6.042507865999996675 ) ) ;
#20244=ORIENTED_EDGE ( 'NONE', *, *, #20097, .F. ) ;
#20250=EDGE_CURVE ( 'NONE', #13182, #28945, #18150, .T. ) ;
#20256=EDGE_CURVE ( 'NONE', #27013, #26158, #29414, .T. ) ;
#20276=CARTESIAN_POINT ( 'NONE',  ( -17.93062603642077946, 10.83602254735704484, -0.6999999999999784173 ) ) ;
#20277=CARTESIAN_POINT ( 'NONE',  ( 17.85846454801659533, 10.13281012205188425, -4.336808689942017736E-16 ) ) ;
#20284=CARTESIAN_POINT ( 'NONE',  ( -18.04593937785069357, 20.00000752677722815, -0.6992883787361406922 ) ) ;
#20302=CARTESIAN_POINT ( 'NONE',  ( 23.69427943123108093, 14.54081805611945910, 6.079851352999988023 ) ) ;
#20323=CARTESIAN_POINT ( 'NONE',  ( -24.25537239878455509, -13.58380780107177976, 5.677299029929432805 ) ) ;
#20341=CARTESIAN_POINT ( 'NONE',  ( -23.81776757772072983, -15.65134804123479917, 4.999998581000003384 ) ) ;
#20351=EDGE_LOOP ( 'NONE', ( #11872, #23822, #8900, #1843 ) ) ;
#20358=CARTESIAN_POINT ( 'NONE',  ( 23.35655559247464907, 15.07705663187610945, 5.680691777000007825 ) ) ;
#20362=FACE_OUTER_BOUND ( 'NONE', #12018, .T. ) ;
#20370=PRODUCT_DEFINITION_SHAPE ( 'NONE', 'NONE',  #21398 ) ;
#20376=CARTESIAN_POINT ( 'NONE',  ( 27.44414120988032124, 5.042033447402311630, 0.2686740700000300741 ) ) ;
#20384=CARTESIAN_POINT ( 'NONE',  ( 24.20792487550426841, -13.66932880343719781, 3.920132063000014710 ) ) ;
#20403=CARTESIAN_POINT ( 'NONE',  ( -0.7153897335033406746, 3.455736562763356279, 0.000000000000000000 ) ) ;
#20406=DIRECTION ( 'NONE',  ( 0.000000000000000000, 0.000000000000000000, -1.000000000000000000 ) ) ;
#20411=CARTESIAN_POINT ( 'NONE',  ( -17.93053308114354394, -8.908107087747509922, 0.000000000000000000 ) ) ;
#20413=CARTESIAN_POINT ( 'NONE',  ( 20.30396079662882158, 20.00000000004802203, 3.000000000000002665 ) ) ;
#20432=CARTESIAN_POINT ( 'NONE',  ( -17.82156395551385941, -9.499568885231910897, 0.000000000000000000 ) ) ;
#20445=B_SPLINE_CURVE_WITH_KNOTS ( 'NONE', 5,
 ( #30988, #26117, #26427, #12246, #7530, #26267, #21549, #2811, #12403 ),
 .UNSPECIFIED., .F., .F.,
 ( 6, 3, 6 ),
 ( 0.000000000000000000, 0.7281981450769999809, 1.224410041430000096 ),
 .UNSPECIFIED. ) ;
#20446=B_SPLINE_CURVE_WITH_KNOTS ( 'NONE', 3,
 ( #8293, #22948, #5940, #3579, #22784, #1237 ),
 .UNSPECIFIED., .F., .F.,
 ( 4, 2, 4 ),
 ( 0.000000000000000000, 0.5000000000000000000, 1.000000000000000000 ),
 .UNSPECIFIED. ) ;
#20447=CARTESIAN_POINT ( 'NONE',  ( 16.40303402075260308, 10.20816091466531716, 0.000000000000000000 ) ) ;
#20461=LINE ( 'NONE', #30215, #1260 ) ;
#20465=ORIENTED_EDGE ( 'NONE', *, *, #3341, .T. ) ;
#20482=VECTOR ( 'NONE', #1682, 1000.000000000000000 ) ;
#20504=EDGE_LOOP ( 'NONE', ( #24847, #7394, #16102, #7120 ) ) ;
#20516=CARTESIAN_POINT ( 'NONE',  ( 1.525061067771818824, -28.45945568257947400, 5.498290041128397476 ) ) ;
#20520=CARTESIAN_POINT ( 'NONE',  ( -25.05552767696902450, 13.58331698520493269, 3.920132093000017193 ) ) ;
#20523=CARTESIAN_POINT ( 'NONE',  ( 24.37165445055180157, -14.77472140295711434, 4.999998581000003384 ) ) ;
#20527=VECTOR ( 'NONE', #13218, 1000.000000000000000 ) ;
#20534=CARTESIAN_POINT ( 'NONE',  ( -23.78314118801539934, -14.39461388281613097, 6.098654095000016540 ) ) ;
#20535=DIRECTION ( 'NONE',  ( -0.7198537139083028835, 0.6941258031311204890, 0.000000000000000000 ) ) ;
#20544=CARTESIAN_POINT ( 'NONE',  ( 21.42460392489384091, 16.40003748012899010, -0.6999999999999784173 ) ) ;
#20545=CARTESIAN_POINT ( 'NONE',  ( -24.18581885410760179, 13.70860090230524975, 6.072235418731803946 ) ) ;
#20553=CARTESIAN_POINT ( 'NONE',  ( 14.25032083473339206, -27.35421241518758961, 0.8585795199999857186 ) ) ;
#20554=ORIENTED_EDGE ( 'NONE', *, *, #24827, .F. ) ;
#20557=CARTESIAN_POINT ( 'NONE',  ( -23.94466870085087606, -15.45669659436210175, 4.319305392000011068 ) ) ;
#20560=CARTESIAN_POINT ( 'NONE',  ( -28.32387083329934185, 4.355427724292508351, 8.000000000000007105 ) ) ;
#20563=CARTESIAN_POINT ( 'NONE',  ( -24.06826084723317649, 20.50742046750733039, 1.000000000000000888 ) ) ;
#20568=B_SPLINE_CURVE_WITH_KNOTS ( 'NONE', 3,
 ( #16084, #15769, #25382, #3820, #13406, #25696 ),
 .UNSPECIFIED., .F., .F.,
 ( 4, 2, 4 ),
 ( 0.000000000000000000, 0.5000000000000000000, 1.000000000000000000 ),
 .UNSPECIFIED. ) ;
#20571=FACE_OUTER_BOUND ( 'NONE', #29492, .T. ) ;
#20577=CARTESIAN_POINT ( 'NONE',  ( 18.11750013309444185, 11.57137507599268389, -4.336808689942017243E-16 ) ) ;
#20585=ORIENTED_EDGE ( 'NONE', *, *, #16208, .T. ) ;
#20588=ADVANCED_FACE ( 'NONE', ( #7096 ), #26605, .F. ) ;
#20596=CARTESIAN_POINT ( 'NONE',  ( -16.29702427720857472, 11.97108418944526420, -4.336808689942018722E-16 ) ) ;
#20603=CARTESIAN_POINT ( 'NONE',  ( 17.04201355855559896, 9.897551528198281545, 0.000000000000000000 ) ) ;
#20606=CARTESIAN_POINT ( 'NONE',  ( 23.39254333661255814, -15.30228500393733526, 8.000000000000007105 ) ) ;
#20608=CARTESIAN_POINT ( 'NONE',  ( 22.47598016381773789, 18.14223004230803227, 1.000000000000000888 ) ) ;
#20611=CARTESIAN_POINT ( 'NONE',  ( 0.5057536231481192246, -27.79562098839016571, 6.099998581000020792 ) ) ;
#20612=ADVANCED_FACE ( 'NONE', ( #25849 ), #23644, .F. ) ;
#20628=B_SPLINE_CURVE_WITH_KNOTS ( 'NONE', 3,
 ( #20070, #19447, #21810, #7484, #15182, #17079 ),
 .UNSPECIFIED., .F., .F.,
 ( 4, 2, 4 ),
 ( 0.000000000000000000, 0.5000000000000000000, 1.000000000000000000 ),
 .UNSPECIFIED. ) ;
#20630=B_SPLINE_CURVE_WITH_KNOTS ( 'NONE', 1,
 ( #30690, #21094 ),
 .UNSPECIFIED., .F., .F.,
 ( 2, 2 ),
 ( -0.7016521142910000508, 3.330669073875469621E-15 ),
 .UNSPECIFIED. ) ;
#20633=ORIENTED_EDGE ( 'NONE', *, *, #24170, .T. ) ;
#20636=CARTESIAN_POINT ( 'NONE',  ( -0.6094664100040195764, -28.49364619262437870, 4.895947184000021046 ) ) ;
#20639=CARTESIAN_POINT ( 'NONE',  ( 24.05454679444040167, -13.93760249370175508, 4.035491118591038706 ) ) ;
#20667=ADVANCED_FACE ( 'NONE', ( #13721 ), #4585, .F. ) ;
#20691=CARTESIAN_POINT ( 'NONE',  ( 21.24683659263830293, 17.15008680908327321, 0.000000000000000000 ) ) ;
#20694=CARTESIAN_POINT ( 'NONE',  ( -23.62421573606080827, -14.65442406347138338, 6.042470790000031400 ) ) ;
#20697=CARTESIAN_POINT ( 'NONE',  ( 24.70074545465923421, -14.21822122957792445, 3.997190862000010725 ) ) ;
#20724=CARTESIAN_POINT ( 'NONE',  ( 28.35945635836379708, 7.983396865348648674, 8.000000000000007105 ) ) ;
#20732=CARTESIAN_POINT ( 'NONE',  ( 23.46464814832361157, 14.90844422066722430, 4.118060943961503462 ) ) ;
#20737=CARTESIAN_POINT ( 'NONE',  ( -17.10083289438509979, 9.923792022609076113, -0.000000000000000000 ) ) ;
#20746=ORIENTED_EDGE ( 'NONE', *, *, #30316, .T. ) ;
#20752=CARTESIAN_POINT ( 'NONE',  ( -16.56625540545879360, -7.923010675351982002, -0.6999999999999784173 ) ) ;
#20758=EDGE_CURVE ( 'NONE', #19797, #2099, #18890, .T. ) ;
#20764=CARTESIAN_POINT ( 'NONE',  ( 28.32389467614452627, -4.355430725511089562, 8.000000000000007105 ) ) ;
#20769=CARTESIAN_POINT ( 'NONE',  ( -0.5821515579339680002, -27.79407096281863687, 4.791896188000022150 ) ) ;
#20772=EDGE_CURVE ( 'NONE', #5681, #7965, #5726, .T. ) ;
#20774=ORIENTED_EDGE ( 'NONE', *, *, #12651, .F. ) ;
#20790=CARTESIAN_POINT ( 'NONE',  ( 24.06750537026301018, 15.26514225575822081, 4.098700193000015091 ) ) ;
#20811=FACE_OUTER_BOUND ( 'NONE', #2448, .T. ) ;
#20821=CARTESIAN_POINT ( 'NONE',  ( -23.84638031100276123, 14.29033435813013853, 4.441358500814834187 ) ) ;
#20841=FACE_OUTER_BOUND ( 'NONE', #8902, .T. ) ;
#20851=ORIENTED_EDGE ( 'NONE', *, *, #19098, .T. ) ;
#20853=CARTESIAN_POINT ( 'NONE',  ( 0.8794532062878365197, -27.78659480101269708, 3.957673652000032405 ) ) ;
#20865=CARTESIAN_POINT ( 'NONE',  ( -17.83929479963776288, 19.99998902616253105, -0.6999999999999784173 ) ) ;
#20872=ORIENTED_EDGE ( 'NONE', *, *, #1482, .F. ) ;
#20882=CARTESIAN_POINT ( 'NONE',  ( -23.81776757772072983, -15.65134804123479917, 4.999998581000003384 ) ) ;
#20897=CARTESIAN_POINT ( 'NONE',  ( 23.81866167241657806, 14.33570040768432996, 3.899998581000013509 ) ) ;
#20903=LINE ( 'NONE', #11457, #16766 ) ;
#20927=CARTESIAN_POINT ( 'NONE',  ( -10.49401243977554188, -26.66603606335209875, 8.000000000000007105 ) ) ;
#20931=CARTESIAN_POINT ( 'NONE',  ( -0.4846640835643744039, -27.79604706135699033, 4.493528488000025689 ) ) ;
#20941=ADVANCED_FACE ( 'NONE', ( #1103, #5510, #22361, #22514 ), #5162, .F. ) ;
#20947=CARTESIAN_POINT ( 'NONE',  ( 23.29312071241426096, 15.17488100587054767, 4.493007569000006640 ) ) ;
#20950=CARTESIAN_POINT ( 'NONE',  ( -0.1501630637024684578, -28.50011693320769623, 4.099092748999999536 ) ) ;
#20953=CARTESIAN_POINT ( 'NONE',  ( 17.16657240419154462, 10.99999999996915179, -0.6999999999999784173 ) ) ;
#20970=CARTESIAN_POINT ( 'NONE',  ( -23.81776757771349295, -15.65134804123035828, 5.147520325772222627 ) ) ;
#20975=ORIENTED_EDGE ( 'NONE', *, *, #5405, .F. ) ;
#20982=ORIENTED_EDGE ( 'NONE', *, *, #19593, .F. ) ;
#20984=B_SPLINE_SURFACE_WITH_KNOTS ( 'NONE', 5, 1, ( 
 ( #24127, #2566 ),
 ( #17034, #12153 ),
 ( #21764, #26787 ),
 ( #9804, #214 ),
 ( #19403, #534 ),
 ( #5228, #5077 ),
 ( #14845, #24436 ),
 ( #2870, #12462 ),
 ( #10116, #19716 ),
 ( #29296, #3325 ),
 ( #27100, #3023 ),
 ( #10271, #13226 ),
 ( #10720, #17493 ),
 ( #29611, #1129 ),
 ( #12777, #8043 ) ),
 .UNSPECIFIED., .F., .F., .F.,
 ( 6, 3, 3, 3, 6 ),
 ( 2, 2 ),
 ( 0.000000000000000000, 0.5239049113010000314, 1.047809822600000107, 1.571714733900000160, 1.746349704340000031 ),
 ( -0.7000000000009999335, 2.557520719980000135E-06 ),
 .UNSPECIFIED. ) ;
#20989=CARTESIAN_POINT ( 'NONE',  ( -24.41841039498785193, -14.69667350221323865, 3.899998581000013509 ) ) ;
#20994=EDGE_CURVE ( 'NONE', #974, #22866, #7623, .T. ) ;
#20997=CARTESIAN_POINT ( 'NONE',  ( -19.42125183333303795, 20.00000466481577988, -0.3145118510766364284 ) ) ;
#21005=CARTESIAN_POINT ( 'NONE',  ( 17.93011078763067090, 11.79183908526299085, -0.6999999999999784173 ) ) ;
#21013=CARTESIAN_POINT ( 'NONE',  ( 16.27441336913832615, 11.65945330722155759, -0.6999999999999783062 ) ) ;
#21028=CARTESIAN_POINT ( 'NONE',  ( 24.71263212711717117, -12.73382341766860293, 4.267021104580390300 ) ) ;
#21031=CARTESIAN_POINT ( 'NONE',  ( -26.80856362799623582, -7.546808677664434306, 0.000000000000000000 ) ) ;
#21038=CARTESIAN_POINT ( 'NONE',  ( -0.1464386043128553250, -27.80011885101413682, 4.099092748999999536 ) ) ;
#21041=CARTESIAN_POINT ( 'NONE',  ( 16.40303402077768169, -9.791839085275103827, -0.6999999999999784173 ) ) ;
#21050=CARTESIAN_POINT ( 'NONE',  ( 26.79556473285982321, 0.4875557887249620803, 0.000000000000000000 ) ) ;
#21053=CARTESIAN_POINT ( 'NONE',  ( 27.79539923781684507, 0.5057481689249188062, 0.8585786439999909536 ) ) ;
#21063=ORIENTED_EDGE ( 'NONE', *, *, #26420, .T. ) ;
#21065=EDGE_LOOP ( 'NONE', ( #25277, #365, #17537, #21250 ) ) ;
#21076=CARTESIAN_POINT ( 'NONE',  ( -17.40480267186241292, 11.95092772882062704, -4.336808689942017243E-16 ) ) ;
#21080=CARTESIAN_POINT ( 'NONE',  ( -17.93324555120827668, 10.97998838178171432, -0.6999999989999727834 ) ) ;
#21087=CARTESIAN_POINT ( 'NONE',  ( -18.81428968775364652, -21.61535361001210731, 8.000000000000007105 ) ) ;
#21089=CARTESIAN_POINT ( 'NONE',  ( 27.31421068595970780, 9.888053941072412201, 0.5017677510000262409 ) ) ;
#21091=CARTESIAN_POINT ( 'NONE',  ( -0.3682501489830092845, -27.79783598715961901, 4.319846982000025370 ) ) ;
#21094=CARTESIAN_POINT ( 'NONE',  ( 23.55411374389282386, 16.04538543799059980, 8.000000000000007105 ) ) ;
#21114=EDGE_CURVE ( 'NONE', #30998, #19325, #28245, .T. ) ;
#21121=DIRECTION ( 'NONE',  ( -0.000000000000000000, 0.000000000000000000, 1.000000000000000000 ) ) ;
#21126=CARTESIAN_POINT ( 'NONE',  ( 1.568292632109252738, -27.75603058367127574, 5.310199493000017590 ) ) ;
#21139=ORIENTED_EDGE ( 'NONE', *, *, #22690, .T. ) ;
#21140=VERTEX_POINT ( 'NONE', #26426 ) ;
#21143=CARTESIAN_POINT ( 'NONE',  ( -16.81341597756113515, 9.900182044522454206, -0.6999999989999727834 ) ) ;
#21157=CARTESIAN_POINT ( 'NONE',  ( 1.645560275461343203, -28.45273235261698019, 4.999998581000003384 ) ) ;
#21171=CARTESIAN_POINT ( 'NONE',  ( 2.131591336857817875, -2.813577582618851380, -0.6999999999999784173 ) ) ;
#21173=ORIENTED_EDGE ( 'NONE', *, *, #29562, .F. ) ;
#21180=B_SPLINE_CURVE_WITH_KNOTS ( 'NONE', 1,
 ( #1664, #20865 ),
 .UNSPECIFIED., .F., .F.,
 ( 2, 2 ),
 ( -0.7031437918980000257, 3.133915349451399379E-11 ),
 .UNSPECIFIED. ) ;
#21186=CARTESIAN_POINT ( 'NONE',  ( 0.2655682516278248806, -27.79918151443105856, 3.920205022000022854 ) ) ;
#21194=CARTESIAN_POINT ( 'NONE',  ( -15.75156552665617937, -9.231204648498994914, 0.000000000000000000 ) ) ;
#21204=CARTESIAN_POINT ( 'NONE',  ( 18.26377084502559356, 11.16397745125027541, -4.336808689942018722E-16 ) ) ;
#21217=CARTESIAN_POINT ( 'NONE',  ( -27.79539923781684507, -0.5057481689249130330, 8.000000000000007105 ) ) ;
#21220=CARTESIAN_POINT ( 'NONE',  ( 27.79539923781684507, 0.5057481689249235801, 8.000000000000007105 ) ) ;
#21229=CARTESIAN_POINT ( 'NONE',  ( -20.30403093138962234, 20.00000000003553424, 1.000000000000000888 ) ) ;
#21233=CARTESIAN_POINT ( 'NONE',  ( 28.64321111491632976, -9.935962574576189255, 0.5017677510000262409 ) ) ;
#21235=CARTESIAN_POINT ( 'NONE',  ( 19.29387769735768998, -21.32719583073583536, 8.000000000000007105 ) ) ;
#21237=B_SPLINE_CURVE_WITH_KNOTS ( 'NONE', 3,
 ( #2773, #10476, #12365, #20073, #29348, #29662, #19451, #19608, #7637, #26838, #5289, #23061 ),
 .UNSPECIFIED., .F., .F.,
 ( 4, 2, 2, 2, 2, 4 ),
 ( 0.000000000000000000, 0.1250000000000004163, 0.2500000000000008327, 0.5000000000000005551, 0.7500000000000002220, 1.000000000000000000 ),
 .UNSPECIFIED. ) ;
#21239=CARTESIAN_POINT ( 'NONE',  ( 23.77307027441306531, -14.41181805765238444, 4.999998581000003384 ) ) ;
#21241=CARTESIAN_POINT ( 'NONE',  ( 0.5057536231481327693, -27.79562098839016571, 3.899998581000013509 ) ) ;
#21250=ORIENTED_EDGE ( 'NONE', *, *, #9442, .F. ) ;
#21254=CARTESIAN_POINT ( 'NONE',  ( -16.91615862483482857, -10.10168739744133859, 0.000000000000000000 ) ) ;
#21255=EDGE_LOOP ( 'NONE', ( #17440, #307, #29616, #12824 ) ) ;
#21258=CARTESIAN_POINT ( 'NONE',  ( 23.83861932470720291, 15.61961844235199948, 4.689445052000001724 ) ) ;
#21261=CARTESIAN_POINT ( 'NONE',  ( 18.15446590459846377, 19.99997493598501208, -0.6870078918781518107 ) ) ;
#21275=CARTESIAN_POINT ( 'NONE',  ( 1.495522319900055574, -27.76012052182101542, 5.506490228000010312 ) ) ;
#21289=ORIENTED_EDGE ( 'NONE', *, *, #11201, .F. ) ;
#21292=CARTESIAN_POINT ( 'NONE',  ( 24.49145441566124148, -14.57548795709913847, 5.680829342999987652 ) ) ;
#21294=DIRECTION ( 'NONE',  ( 0.000000000000000000, 0.000000000000000000, -1.000000000000000000 ) ) ;
#21301=B_SPLINE_CURVE_WITH_KNOTS ( 'NONE', 3,
 ( #19070, #512, #2549, #28666, #12443, #22061 ),
 .UNSPECIFIED., .F., .F.,
 ( 4, 2, 4 ),
 ( 0.000000000000000000, 0.5000000000000000000, 1.000000000000000000 ),
 .UNSPECIFIED. ) ;
#21306=CARTESIAN_POINT ( 'NONE',  ( -18.70388666750742246, 19.99992613001282038, -0.5969568546230863415 ) ) ;
#21309=CARTESIAN_POINT ( 'NONE',  ( -27.29371452669260734, -0.4966198192113801535, -0.6577119969999878357 ) ) ;
#21310=EDGE_LOOP ( 'NONE', ( #19515, #21572, #7236, #8658 ) ) ;
#21312=CARTESIAN_POINT ( 'NONE',  ( 1.344125205454980154, -28.46870209102154448, 4.240358041999986227 ) ) ;
#21326=ADVANCED_FACE ( 'NONE', ( #30797 ), #9076, .F. ) ;
#21336=CARTESIAN_POINT ( 'NONE',  ( -24.90295381356148141, -14.88027900779681723, 0.2686745300000126235 ) ) ;
#21341=CARTESIAN_POINT ( 'NONE',  ( -24.06750537087913600, -15.26514226587110379, 4.098700198000015504 ) ) ;
#21349=DIRECTION ( 'NONE',  ( -0.8687154346624373913, -0.4953115116563036602, 0.000000000000000000 ) ) ;
#21350=EDGE_CURVE ( 'NONE', #5339, #15540, #6087, .T. ) ;
#21364=FACE_OUTER_BOUND ( 'NONE', #28134, .T. ) ;
#21374=ORIENTED_EDGE ( 'NONE', *, *, #3854, .T. ) ;
#21380=EDGE_CURVE ( 'NONE', #30700, #25431, #4552, .T. ) ;
#21382=CARTESIAN_POINT ( 'NONE',  ( -25.38146355688631317, 12.59839640959181395, 8.000000000000007105 ) ) ;
#21384=FACE_BOUND ( 'NONE', #15063, .T. ) ;
#21398=PRODUCT_DEFINITION ( 'UNKNOWN', '', #26920, #15959 ) ;
#21399=CARTESIAN_POINT ( 'NONE',  ( -18.92328505709462405, 19.72870074452574940, 0.1493323239999955199 ) ) ;
#21402=CARTESIAN_POINT ( 'NONE',  ( -24.54452542612009225, -14.48555670042145138, 6.079852602000002548 ) ) ;
#21404=CARTESIAN_POINT ( 'NONE',  ( -24.32472894358752313, 13.45989150749028873, 3.899998581000013509 ) ) ;
#21408=ADVANCED_FACE ( 'NONE', ( #20571 ), #416, .F. ) ;
#21417=CARTESIAN_POINT ( 'NONE',  ( -17.01911899311089371, -10.09155933042922726, 0.000000000000000000 ) ) ;
#21419=DIRECTION ( 'NONE',  ( 0.7198537139083028835, -0.6941258031311204890, 0.000000000000000000 ) ) ;
#21420=CARTESIAN_POINT ( 'NONE',  ( 23.23277125981546476, 15.26692728828886025, 4.895813257000003915 ) ) ;
#21425=CARTESIAN_POINT ( 'NONE',  ( -24.60726957497166367, 14.37955347300500364, 5.901399683999997592 ) ) ;
#21443=CARTESIAN_POINT ( 'NONE',  ( 24.41841038956698640, 14.69667349781389376, 3.899998581000013509 ) ) ;
#21444=ADVANCED_FACE ( 'NONE', ( #9225 ), #28897, .F. ) ;
#21454=CARTESIAN_POINT ( 'NONE',  ( 27.03594125075309762, 0.4919295335571040040, -0.6999999999999784173 ) ) ;
#21462=CARTESIAN_POINT ( 'NONE',  ( -20.08956181735672430, 20.00001759534566403, 0.2963061688068184263 ) ) ;
#21469=CARTESIAN_POINT ( 'NONE',  ( 1.605176535610508326, -27.75389821387976852, 4.999998581000003384 ) ) ;
#21471=DIRECTION ( 'NONE',  ( 0.6941258031311203780, 0.7198537139083029945, 0.000000000000000000 ) ) ;
#21477=CARTESIAN_POINT ( 'NONE',  ( -17.62526668112344908, -8.236461616547455122, -0.6999999999999784173 ) ) ;
#21478=EDGE_CURVE ( 'NONE', #2398, #931, #10180, .T. ) ;
#21484=PRESENTATION_STYLE_ASSIGNMENT (( #17062 ) ) ;
#21487=CARTESIAN_POINT ( 'NONE',  ( 23.94793942833934963, 15.45149536900696674, 5.679609032776862243 ) ) ;
#21490=CARTESIAN_POINT ( 'NONE',  ( -26.03214543848244844, 7.091100912325356553, 0.000000000000000000 ) ) ;
#21493=CARTESIAN_POINT ( 'NONE',  ( -24.38199545545641911, -14.75707035126829147, 3.901343066999990228 ) ) ;
#21510=DIRECTION ( 'NONE',  ( -0.7198537139083028835, 0.6941258031311204890, 0.000000000000000000 ) ) ;
#21519=ORIENTED_EDGE ( 'NONE', *, *, #19642, .T. ) ;
#21528=CARTESIAN_POINT ( 'NONE',  ( -15.73360964030186970, 11.02001161816959396, -1.000005633855494125E-09 ) ) ;
#21549=CARTESIAN_POINT ( 'NONE',  ( -15.97294062935416115, -8.309387060397886771, 0.000000000000000000 ) ) ;
#21550=CARTESIAN_POINT ( 'NONE',  ( -19.18296382695153213, 19.99999944541083963, -0.4461354429999841997 ) ) ;
#21559=CARTESIAN_POINT ( 'NONE',  ( -17.62526623054365871, -8.236462051082252600, 0.000000000000000000 ) ) ;
#21560=CARTESIAN_POINT ( 'NONE',  ( -15.73360964037622622, -8.979988381802643360, -0.6999999999999784173 ) ) ;
#21564=CARTESIAN_POINT ( 'NONE',  ( 24.73568148353697183, -12.68911065183860920, 4.319165765000021473 ) ) ;
#21572=ORIENTED_EDGE ( 'NONE', *, *, #29562, .T. ) ;
#21573=CARTESIAN_POINT ( 'NONE',  ( -17.54655709608498881, -9.840444911176506437, 0.000000000000000000 ) ) ;
#21575=CARTESIAN_POINT ( 'NONE',  ( 16.06675444876397307, -9.020011618195203695, -1.000005633855494125E-09 ) ) ;
#21587=CARTESIAN_POINT ( 'NONE',  ( 3.063912144317538111, -1.789060389098976911, 0.000000000000000000 ) ) ;
#21590=CARTESIAN_POINT ( 'NONE',  ( 19.99486320633338465, 19.99999931165986311, 0.1511489130000265302 ) ) ;
#21594=CARTESIAN_POINT ( 'NONE',  ( -24.25742564193969031, -13.58028021372842531, 4.319317663000004970 ) ) ;
#21597=ADVANCED_FACE ( 'NONE', ( #29815 ), #9949, .T. ) ;
#21615=CARTESIAN_POINT ( 'NONE',  ( 18.92356420714367360, 19.72862907665551546, 0.1494310229999962214 ) ) ;
#21619=CARTESIAN_POINT ( 'NONE',  ( -24.41841039498785193, -14.69667350221323865, 3.899998581000013509 ) ) ;
#21629=DIRECTION ( 'NONE',  ( -0.6941258031311203780, -0.7198537139083029945, 0.000000000000000000 ) ) ;
#21669=CARTESIAN_POINT ( 'NONE',  ( -25.05552767696902450, 13.58331698520493269, 3.920132093000017193 ) ) ;
#21677=B_SPLINE_CURVE_WITH_KNOTS ( 'NONE', 5,
 ( #2100, #4309, #27744, #23514, #30588, #11693, #25717, #18305, #13905, #21292, #1948, #6188, #11542, #9017, #18460 ),
 .UNSPECIFIED., .F., .F.,
 ( 6, 3, 3, 3, 6 ),
 ( 0.000000000000000000, 0.1000000000022904789, 0.3999999999977094656, 0.7000000000005727196, 1.000000000000000000 ),
 .UNSPECIFIED. ) ;
#21688=CARTESIAN_POINT ( 'NONE',  ( -23.77307140041805411, 14.41181874028064591, 4.999998581000003384 ) ) ;
#21689=CARTESIAN_POINT ( 'NONE',  ( -25.38146355678814814, 12.59839640969361696, 1.000000000000000888 ) ) ;
#21690=AXIS2_PLACEMENT_3D ( 'NONE', #23491, #1928, #21121 ) ;
#21692=B_SPLINE_CURVE_WITH_KNOTS ( 'NONE', 3,
 ( #9115, #18563, #30379, #4254, #6448, #13849 ),
 .UNSPECIFIED., .F., .F.,
 ( 4, 2, 4 ),
 ( 0.000000000000000000, 0.5000000000000000000, 1.000000000000000000 ),
 .UNSPECIFIED. ) ;
#21695=CARTESIAN_POINT ( 'NONE',  ( -27.79539923781770128, -0.5057481688779147389, 8.000000000000007105 ) ) ;
#21696=VERTEX_POINT ( 'NONE', #28707 ) ;
#21700=CARTESIAN_POINT ( 'NONE',  ( -17.62526668104891314, 11.76353838341477953, 0.000000000000000000 ) ) ;
#21703=CARTESIAN_POINT ( 'NONE',  ( -18.15338440918069907, 19.92139857694655802, 0.007026247000024854472 ) ) ;
#21708=DIRECTION ( 'NONE',  ( 0.6941258031311203780, 0.7198537139083029945, 0.000000000000000000 ) ) ;
#21719=ORIENTED_EDGE ( 'NONE', *, *, #3307, .F. ) ;
#21722=CARTESIAN_POINT ( 'NONE',  ( -20.26572724632349320, -21.15151735177849091, 1.000000000000000888 ) ) ;
#21724=CARTESIAN_POINT ( 'NONE',  ( 25.80996960090668679, 10.85703805089278617, 8.000000000000007105 ) ) ;
#21726=CARTESIAN_POINT ( 'NONE',  ( 18.21075248917225409, 19.99999500955443921, -0.6817400023187817348 ) ) ;
#21736=CARTESIAN_POINT ( 'NONE',  ( 24.61381495442905276, 14.36755986797187923, 6.042472827000016977 ) ) ;
#21737=CARTESIAN_POINT ( 'NONE',  ( -16.99800964883880638, 12.09718744067793317, -0.6999999999999783062 ) ) ;
#21741=CARTESIAN_POINT ( 'NONE',  ( 0.8794532062938354988, -27.78659480101258694, 6.042323509000024906 ) ) ;
#21746=CARTESIAN_POINT ( 'NONE',  ( 1.632956991020356519, -28.45346066249067007, 4.791883387999989807 ) ) ;
#21749=B_SPLINE_CURVE_WITH_KNOTS ( 'NONE', 5,
 ( #5372, #14980, #24577, #17479, #3011, #17626 ),
 .UNSPECIFIED., .F., .F.,
 ( 6, 6 ),
 ( 77.28585173369999950, 94.75474465359999954 ),
 .UNSPECIFIED. ) ;
#21751=CARTESIAN_POINT ( 'NONE',  ( 23.94466869970572986, 15.45669658583985751, 4.319305385000027364 ) ) ;
#21755=B_SPLINE_SURFACE_WITH_KNOTS ( 'NONE', 5, 5, ( 
 ( #14242, #29014, #7460, #24002, #17057, #5096, #24296, #9352, #28560 ),
 ( #9518, #19115, #2746, #21947, #28709, #7155, #16738, #88, #9667 ),
 ( #1153, #15319, #13100, #26811, #17817, #26969, #24920, #3347, #5257 ),
 ( #7765, #10137, #22409, #19581, #14867, #7912, #27123, #15015, #5404 ),
 ( #17516, #24611, #17363, #5556, #27273, #3196, #2894, #15158, #7611 ),
 ( #24458, #27425, #3045, #12954, #22564, #12486, #704, #12636, #19738 ) ),
 .UNSPECIFIED., .F., .F., .F.,
 ( 6, 6 ),
 ( 6, 3, 6 ),
 ( 0.000000000000000000, 23.96001935709999842 ),
 ( 8.011061266649999624, 8.811950030160000225, 9.612838793659999936 ),
 .UNSPECIFIED. ) ;
#21762=CARTESIAN_POINT ( 'NONE',  ( 17.18658402238548533, 9.900182044515950963, -0.6999999999999784173 ) ) ;
#21763=ORIENTED_EDGE ( 'NONE', *, *, #20256, .F. ) ;
#21764=CARTESIAN_POINT ( 'NONE',  ( -25.45799949038170240, 12.81261085762170815, 5.208434320000010942 ) ) ;
#21765=DIRECTION ( 'NONE',  ( 0.000000000000000000, 0.000000000000000000, -1.000000000000000000 ) ) ;
#21767=CARTESIAN_POINT ( 'NONE',  ( 24.32472724076343695, -13.45989056521276872, 6.099998581000020792 ) ) ;
#21778=CARTESIAN_POINT ( 'NONE',  ( 28.49528339128749366, 0.5184828350247212558, 1.000000000000000888 ) ) ;
#21779=DIRECTION ( 'NONE',  ( 0.000000000000000000, 0.000000000000000000, -1.000000000000000000 ) ) ;
#21789=VERTEX_POINT ( 'NONE', #26657 ) ;
#21793=ORIENTED_EDGE ( 'NONE', *, *, #23384, .T. ) ;
#21810=CARTESIAN_POINT ( 'NONE',  ( -15.86234340635861173, 10.46359668131463216, -1.384526174263989162E-13 ) ) ;
#21821=CARTESIAN_POINT ( 'NONE',  ( -4.785279987111795030, -31.71089578012187360, 0.7595836940000044724 ) ) ;
#21826=CARTESIAN_POINT ( 'NONE',  ( 17.14656078602323319, -7.900182044548062166, -0.6999999999999784173 ) ) ;
#21827=CARTESIAN_POINT ( 'NONE',  ( 24.75645985066559263, 14.12045945726143970, 5.901294549000013490 ) ) ;
#21829=CARTESIAN_POINT ( 'NONE',  ( 19.80526555972147307, 19.50877392102524155, 2.200000000000007283 ) ) ;
#21837=ORIENTED_EDGE ( 'NONE', *, *, #17750, .T. ) ;
#21847=CARTESIAN_POINT ( 'NONE',  ( -24.37165444408190851, 14.77472139917419369, 4.999998581000003384 ) ) ;
#21849=B_SPLINE_CURVE_WITH_KNOTS ( 'NONE', 5,
 ( #17602, #29568, #1250, #10846, #22958, #20432, #27363, #15703, #1406, #30029, #18059, #8460 ),
 .UNSPECIFIED., .F., .F.,
 ( 6, 3, 3, 6 ),
 ( 1.224410003600000074, 1.456394985740000037, 2.184590823429999773, 2.448622002460000058 ),
 .UNSPECIFIED. ) ;
#21850=B_SPLINE_CURVE_WITH_KNOTS ( 'NONE', 3,
 ( #29806, #13442, #22735, #8394, #8239, #13126 ),
 .UNSPECIFIED., .F., .F.,
 ( 4, 2, 4 ),
 ( 0.000000000000000000, 0.5000000000000000000, 1.000000000000000000 ),
 .UNSPECIFIED. ) ;
#21858=CARTESIAN_POINT ( 'NONE',  ( -24.97472003774791816, -13.73006752753317450, 4.791638085000021974 ) ) ;
#21862=B_SPLINE_SURFACE_WITH_KNOTS ( 'NONE', 5, 1, ( 
 ( #26930, #12296 ),
 ( #4907, #12442 ),
 ( #2851, #10249 ),
 ( #5205, #29275 ),
 ( #5516, #7269 ),
 ( #26464, #21594 ),
 ( #43, #24108 ),
 ( #26767, #14820 ),
 ( #7718, #17321 ),
 ( #9938, #7418 ),
 ( #24417, #22060 ),
 ( #16858, #2548 ),
 ( #9623, #21909 ),
 ( #7569, #19224 ),
 ( #12135, #511 ) ),
 .UNSPECIFIED., .F., .F., .F.,
 ( 6, 3, 3, 3, 6 ),
 ( 2, 2 ),
 ( 0.000000000000000000, 0.5239010162240000934, 1.047802032450000143, 1.571703048670000102, 1.746336720750000016 ),
 ( -0.7000000000009999335, 2.556017480449999863E-06 ),
 .UNSPECIFIED. ) ;
#21866=CARTESIAN_POINT ( 'NONE',  ( -15.73624015604650772, 11.16458205270512138, -0.6999999999999783062 ) ) ;
#21869=CARTESIAN_POINT ( 'NONE',  ( -24.36725163763869162, -13.38201776504303986, 4.999998581000003384 ) ) ;
#21870=CARTESIAN_POINT ( 'NONE',  ( -24.41841039498785193, -14.69667350221323865, 6.099998581000020792 ) ) ;
#21880=ORIENTED_EDGE ( 'NONE', *, *, #28848, .F. ) ;
#21888=ORIENTED_EDGE ( 'NONE', *, *, #26679, .T. ) ;
#21891=DIRECTION ( 'NONE',  ( 0.000000000000000000, 0.000000000000000000, -1.000000000000000000 ) ) ;
#21894=CARTESIAN_POINT ( 'NONE',  ( -24.30808044443811156, 13.48997716914403533, 6.099998581000020792 ) ) ;
#21900=CARTESIAN_POINT ( 'NONE',  ( 2.347741120694188055, -2.634769306325225102, 0.000000000000000000 ) ) ;
#21903=CARTESIAN_POINT ( 'NONE',  ( 24.45473033137484720, 14.63622297804190175, 6.098654221000004760 ) ) ;
#21908=CARTESIAN_POINT ( 'NONE',  ( 1.568292632109252738, -27.75603058367127574, 5.310199493000017590 ) ) ;
#21909=CARTESIAN_POINT ( 'NONE',  ( -23.85408962131194954, -14.27673465746016213, 3.901342939999996595 ) ) ;
#21914=CARTESIAN_POINT ( 'NONE',  ( 16.59519732816799475, 11.95092772887203836, -4.336808689942017243E-16 ) ) ;
#21934=CARTESIAN_POINT ( 'NONE',  ( 18.24356172924623820, -9.267172192657799457, -0.6999999999999784173 ) ) ;
#21937=CARTESIAN_POINT ( 'NONE',  ( 0.5537481963838299936, -28.49486543565701169, 3.899998581000013509 ) ) ;
#21941=LINE ( 'NONE', #699, #8729 ) ;
#21945=CARTESIAN_POINT ( 'NONE',  ( 26.79556473285982321, 0.4875557887249620803, 0.000000000000000000 ) ) ;
#21946=EDGE_CURVE ( 'NONE', #17896, #931, #16912, .T. ) ;
#21947=CARTESIAN_POINT ( 'NONE',  ( -27.32958467830413340, 4.204436669847241070, 0.08279779300002232389 ) ) ;
#21949=EDGE_LOOP ( 'NONE', ( #28222, #9689, #9566, #3554 ) ) ;
#21955=EDGE_CURVE ( 'NONE', #26866, #18702, #30481, .T. ) ;
#21963=CARTESIAN_POINT ( 'NONE',  ( 17.85685193652881964, -9.868837085878030990, -0.6999999999999784173 ) ) ;
#21976=CARTESIAN_POINT ( 'NONE',  ( -17.46782121558967660, -8.097265036127433646, 0.000000000000000000 ) ) ;
#21977=EDGE_CURVE ( 'NONE', #21789, #1557, #5707, .T. ) ;
#21978=CARTESIAN_POINT ( 'NONE',  ( 14.12863464165936378, -27.12057300290972250, -0.5592437529999827461 ) ) ;
#21979=CARTESIAN_POINT ( 'NONE',  ( -24.83272648880584654, 12.49791454310039640, 4.791562840999991302 ) ) ;
#21982=EDGE_CURVE ( 'NONE', #16634, #1011, #14316, .T. ) ;
#21993=ORIENTED_EDGE ( 'NONE', *, *, #11254, .F. ) ;
#22000=CARTESIAN_POINT ( 'NONE',  ( -19.80535357367646654, 19.50875577052770993, 3.799999999999998046 ) ) ;
#22006=ORIENTED_EDGE ( 'NONE', *, *, #10616, .F. ) ;
#22023=CARTESIAN_POINT ( 'NONE',  ( -24.98081131316241255, -13.71897606304888662, 4.999998581000003384 ) ) ;
#22031=CARTESIAN_POINT ( 'NONE',  ( 24.63375101525831212, -12.88633855020851904, 4.098596794000014754 ) ) ;
#22046=CARTESIAN_POINT ( 'NONE',  ( -24.29138540600951046, 13.52003710149997140, 6.098655051000018368 ) ) ;
#22054=CARTESIAN_POINT ( 'NONE',  ( 24.00289804085882039, -14.02635914341071732, 5.901399682999991292 ) ) ;
#22060=CARTESIAN_POINT ( 'NONE',  ( -23.94167924027569327, -14.12976891190553452, 3.920144560000005107 ) ) ;
#22061=CARTESIAN_POINT ( 'NONE',  ( 16.06675444873834380, 10.97998838177521286, -1.000005633855494125E-09 ) ) ;
#22062=ORIENTED_EDGE ( 'NONE', *, *, #8047, .T. ) ;
#22111=CARTESIAN_POINT ( 'NONE',  ( -24.26970568828705055, 13.25034242773538118, -0.6999999999999784173 ) ) ;
#22132=EDGE_CURVE ( 'NONE', #19797, #19325, #22162, .T. ) ;
#22148=CARTESIAN_POINT ( 'NONE',  ( -24.27467683362817397, 13.55001165674122987, 3.904029272000009154 ) ) ;
#22151=CARTESIAN_POINT ( 'NONE',  ( 24.93720649360215802, -13.79881813812812297, 6.099998581000020792 ) ) ;
#22153=CARTESIAN_POINT ( 'NONE',  ( -27.66290831536081285, -7.787312998891453120, 8.000000000000007105 ) ) ;
#22156=CARTESIAN_POINT ( 'NONE',  ( 24.83401022448529005, 13.98326749045440032, 4.239871879999995485 ) ) ;
#22161=CARTESIAN_POINT ( 'NONE',  ( -0.5944614571882205212, -27.79380703160649446, 4.999998581000003384 ) ) ;
#22162=B_SPLINE_CURVE_WITH_KNOTS ( 'NONE', 5,
 ( #23340, #11373, #27421, #26007, #6958, #4448, #16400, #26582, #26728, #2659, #1935, #5022, #6642, #5166, #18913 ),
 .UNSPECIFIED., .F., .F.,
 ( 6, 3, 3, 3, 6 ),
 ( 0.000000000000000000, 0.09999999999828211583, 0.3999999999988547161, 0.6999999999994273026, 1.000000000000000000 ),
 .UNSPECIFIED. ) ;
#22192=CARTESIAN_POINT ( 'NONE',  ( 17.14656078599760392, 12.09981795542235439, -0.6999999999999784173 ) ) ;
#22200=CARTESIAN_POINT ( 'NONE',  ( -28.49528339128749366, -0.5184828350247703277, 1.000000000000000888 ) ) ;
#22227=CARTESIAN_POINT ( 'NONE',  ( -24.50349639151496106, 13.13224293120369524, 6.042507865999996675 ) ) ;
#22229=CARTESIAN_POINT ( 'NONE',  ( -28.68577477009351995, 9.950727454193893706, 8.000000000000007105 ) ) ;
#22232=CARTESIAN_POINT ( 'NONE',  ( -19.80535357377644701, 19.50875577052588739, 3.000000106999994642 ) ) ;
#22261=CARTESIAN_POINT ( 'NONE',  ( 16.10001530785001123, 10.69382497330225767, -0.000000000000000000 ) ) ;
#22278=CARTESIAN_POINT ( 'NONE',  ( -4.499842235593497719, -29.81936866046843093, -0.6999999999999784173 ) ) ;
#22287=CARTESIAN_POINT ( 'NONE',  ( 0.4478609109052260062, -28.49673184309145668, 6.098651241000007772 ) ) ;
#22299=EDGE_CURVE ( 'NONE', #29242, #25227, #29315, .T. ) ;
#22302=VECTOR ( 'NONE', #9587, 1000.000000000000000 ) ;
#22306=CARTESIAN_POINT ( 'NONE',  ( -23.56862142526452786, 14.78130733048562995, 8.000000000000007105 ) ) ;
#22307=CARTESIAN_POINT ( 'NONE',  ( 25.12046395012763256, -13.46291002078069887, 6.042507865999996675 ) ) ;
#22311=CARTESIAN_POINT ( 'NONE',  ( 24.47278418934676836, 14.60601539428441598, 3.904031772999999816 ) ) ;
#22318=B_SPLINE_CURVE_WITH_KNOTS ( 'NONE', 3,
 ( #24587, #29609, #15136, #29452, #24736, #5686 ),
 .UNSPECIFIED., .F., .F.,
 ( 4, 2, 4 ),
 ( 0.000000000000000000, 0.5000000000000000000, 1.000000000000000000 ),
 .UNSPECIFIED. ) ;
#22338=ORIENTED_EDGE ( 'NONE', *, *, #28904, .F. ) ;
#22339=ADVANCED_FACE ( 'NONE', ( #8767 ), #25933, .F. ) ;
#22342=CARTESIAN_POINT ( 'NONE',  ( 27.79539923781924315, 0.5057481687932352532, 1.000000000000000888 ) ) ;
#22361=FACE_BOUND ( 'NONE', #18266, .T. ) ;
#22371=CARTESIAN_POINT ( 'NONE',  ( 18.11692203360697562, -8.427117116353246118, -0.6999999999999784173 ) ) ;
#22374=DIRECTION ( 'NONE',  ( 0.000000000000000000, 0.000000000000000000, -1.000000000000000000 ) ) ;
#22383=CARTESIAN_POINT ( 'NONE',  ( -16.81341597756113515, 9.900182044522454206, -0.6999999999999784173 ) ) ;
#22396=CARTESIAN_POINT ( 'NONE',  ( 23.89354037824641708, 14.21129111442623660, 6.099998580999996811 ) ) ;
#22400=CARTESIAN_POINT ( 'NONE',  ( -3.040504020835836041, -1.733590291693717145, -0.6999999999999784173 ) ) ;
#22408=EDGE_CURVE ( 'NONE', #28115, #14021, #28934, .T. ) ;
#22409=CARTESIAN_POINT ( 'NONE',  ( -24.31698661571731890, 13.27613583500951755, 0.02487588100000270863 ) ) ;
#22417=B_SPLINE_CURVE_WITH_KNOTS ( 'NONE', 1,
 ( #26431, #29236 ),
 .UNSPECIFIED., .F., .F.,
 ( 2, 2 ),
 ( -2.557520719980000135E-06, 0.7000000000009999335 ),
 .UNSPECIFIED. ) ;
#22433=CARTESIAN_POINT ( 'NONE',  ( -24.83401023410007724, -13.98326748972919553, 5.760125276000005456 ) ) ;
#22434=ADVANCED_FACE ( 'NONE', ( #21364 ), #2478, .F. ) ;
#22439=CARTESIAN_POINT ( 'NONE',  ( 24.03254869350325507, -20.47699196171803848, 0.5017677510000262409 ) ) ;
#22444=B_SPLINE_CURVE_WITH_KNOTS ( 'NONE', 5,
 ( #20523, #30124, #17989, #10615, #27442, #22893, #27601, #29495, #26988, #7934, #17383, #15490, #20065, #24782, #12826 ),
 .UNSPECIFIED., .F., .F.,
 ( 6, 3, 3, 3, 6 ),
 ( 0.000000000000000000, 0.2999999999994273914, 0.5999999999977095877, 0.8999999999937011719, 1.000000000000000000 ),
 .UNSPECIFIED. ) ;
#22454=CARTESIAN_POINT ( 'NONE',  ( 27.24406355354254217, 0.4957164003247201967, 0.08279779300002232389 ) ) ;
#22459=CARTESIAN_POINT ( 'NONE',  ( 24.93720649360215802, -13.79881813812812297, 3.899998581000013509 ) ) ;
#22461=CARTESIAN_POINT ( 'NONE',  ( -24.62904075447892183, 12.95915071291530829, 8.000000000000007105 ) ) ;
#22464=ORIENTED_EDGE ( 'NONE', *, *, #25415, .F. ) ;
#22466=CARTESIAN_POINT ( 'NONE',  ( -24.86822223968379575, -13.92223202017373573, 4.319317663000004970 ) ) ;
#22476=CYLINDRICAL_SURFACE ( 'NONE', #27287, 1.100000000000002309 ) ;
#22480=CARTESIAN_POINT ( 'NONE',  ( 0.5057536231481192246, -27.79562098839016571, 6.099998581000020792 ) ) ;
#22485=EDGE_CURVE ( 'NONE', #29063, #26584, #5273, .T. ) ;
#22497=CARTESIAN_POINT ( 'NONE',  ( 23.85408961476034051, 14.27673465474052072, 3.901342939999996595 ) ) ;
#22505=CARTESIAN_POINT ( 'NONE',  ( -21.71008920740291259, 18.50699696262706695, 5.000000064000004407 ) ) ;
#22506=ORIENTED_EDGE ( 'NONE', *, *, #20200, .F. ) ;
#22512=CARTESIAN_POINT ( 'NONE',  ( 16.50835677013856184, 10.10662636436282824, 0.000000000000000000 ) ) ;
#22514=FACE_OUTER_BOUND ( 'NONE', #18764, .T. ) ;
#22524=CARTESIAN_POINT ( 'NONE',  ( 23.47637528925218575, 14.89020703997133488, 5.901296968999991677 ) ) ;
#22528=DIRECTION ( 'NONE',  ( 8.432460690569534438E-06, -1.375682488550163830E-15, -0.9999999999644468840 ) ) ;
#22529=ORIENTED_EDGE ( 'NONE', *, *, #27492, .F. ) ;
#22530=CARTESIAN_POINT ( 'NONE',  ( 24.41841038956698640, 14.69667349781389376, 3.899998581000013509 ) ) ;
#22534=ADVANCED_FACE ( 'NONE', ( #7646 ), #17243, .F. ) ;
#22541=CARTESIAN_POINT ( 'NONE',  ( 0.2722179827725955126, -28.49915599500044650, 6.079792140000011891 ) ) ;
#22543=ADVANCED_FACE ( 'NONE', ( #20226 ), #26779, .F. ) ;
#22544=CARTESIAN_POINT ( 'NONE',  ( 19.79257030269742756, 19.51192911135138175, 0.8505974720000031297 ) ) ;
#22546=ORIENTED_EDGE ( 'NONE', *, *, #11604, .T. ) ;
#22555=VECTOR ( 'NONE', #3881, 1000.000000000000000 ) ;
#22556=CARTESIAN_POINT ( 'NONE',  ( -3.267430459342683502, -1.335589246056428481, -0.6999999999999783062 ) ) ;
#22560=EDGE_LOOP ( 'NONE', ( #8181, #24542, #13627, #22529 ) ) ;
#22564=CARTESIAN_POINT ( 'NONE',  ( -18.32611560640161841, 20.54576001036038946, 0.2686742430000332860 ) ) ;
#22573=CARTESIAN_POINT ( 'NONE',  ( 1.605176535610508326, -27.75389821387976852, 4.999998581000003384 ) ) ;
#22577=CARTESIAN_POINT ( 'NONE',  ( -28.12662833602211876, 4.327055432336234020, -0.2432540810000105580 ) ) ;
#22588=VECTOR ( 'NONE', #21765, 1000.000000000000000 ) ;
#22596=CARTESIAN_POINT ( 'NONE',  ( -23.35655559443967988, -15.07705663931308671, 5.680691770000024121 ) ) ;
#22602=CARTESIAN_POINT ( 'NONE',  ( 0.5057536231481192246, -27.79562098839016571, 6.099998581000020792 ) ) ;
#22603=B_SPLINE_CURVE_WITH_KNOTS ( 'NONE', 5,
 ( #30241, #28766, #30985, #27883, #7220, #9416, #23015, #2505, #15922, #4551, #24066, #28623, #25376, #23171, #18867 ),
 .UNSPECIFIED., .F., .F.,
 ( 6, 3, 3, 3, 6 ),
 ( 0.000000000000000000, 0.09999999999599168410, 0.4000000000011452173, 0.6999999999988546495, 1.000000000000000000 ),
 .UNSPECIFIED. ) ;
#22612=CARTESIAN_POINT ( 'NONE',  ( 14.25032083441342934, -27.35421241409322946, 0.9999999950000004745 ) ) ;
#22624=CARTESIAN_POINT ( 'NONE',  ( -17.59696597919420213, 10.20816091468181774, -0.6999999989999727834 ) ) ;
#22646=CARTESIAN_POINT ( 'NONE',  ( 24.83401022448529005, 13.98326749045440032, 4.239871879999995485 ) ) ;
#22662=CARTESIAN_POINT ( 'NONE',  ( 18.17095938919667475, 20.37181511208520135, -0.6577119969999878357 ) ) ;
#22665=ORIENTED_EDGE ( 'NONE', *, *, #10171, .T. ) ;
#22667=CARTESIAN_POINT ( 'NONE',  ( 23.25311087529421172, 15.23597699658644800, 5.310552110000033466 ) ) ;
#22675=ORIENTED_EDGE ( 'NONE', *, *, #10367, .F. ) ;
#22676=ADVANCED_FACE ( 'NONE', ( #19423 ), #21755, .T. ) ;
#22685=CARTESIAN_POINT ( 'NONE',  ( -24.36725163763869162, -13.38201776504303986, 4.999998581000003384 ) ) ;
#22690=EDGE_CURVE ( 'NONE', #7951, #3809, #16169, .T. ) ;
#22695=CARTESIAN_POINT ( 'NONE',  ( 23.96498963411518446, 14.09036522719675411, 6.071979371979260520 ) ) ;
#22699=EDGE_CURVE ( 'NONE', #10529, #26737, #9039, .T. ) ;
#22705=CARTESIAN_POINT ( 'NONE',  ( -24.26927060885717680, -14.94229635206700380, 6.073751778336542451 ) ) ;
#22724=CARTESIAN_POINT ( 'NONE',  ( -27.29371452669260734, -0.4966198192112916687, -0.6577119969999878357 ) ) ;
#22732=AXIS2_PLACEMENT_3D ( 'NONE', #18593, #26151, #23956 ) ;
#22735=CARTESIAN_POINT ( 'NONE',  ( 16.86019302169865952, -7.934232311421240524, -0.6999999999999785283 ) ) ;
#22737=CARTESIAN_POINT ( 'NONE',  ( 23.82458380820737531, 13.44211522811278314, 0.000000000000000000 ) ) ;
#22739=CARTESIAN_POINT ( 'NONE',  ( 16.21708931935714304, -9.573165759297907584, -0.000000000000000000 ) ) ;
#22741=CARTESIAN_POINT ( 'NONE',  ( -23.81866442513004856, -14.33570206453694240, 6.099998581000020792 ) ) ;
#22744=CARTESIAN_POINT ( 'NONE',  ( 24.32472894995379420, -13.45989151107506387, 3.899998581000013509 ) ) ;
#22752=CARTESIAN_POINT ( 'NONE',  ( 17.93011078765611543, -8.208160914697428368, -0.6999999999999784173 ) ) ;
#22756=DIRECTION ( 'NONE',  ( -0.7198537139083028835, 0.6941258031311204890, 0.000000000000000000 ) ) ;
#22758=CARTESIAN_POINT ( 'NONE',  ( 27.79539923781684507, 0.5057481689249200274, 1.000000000000000888 ) ) ;
#22761=CARTESIAN_POINT ( 'NONE',  ( 25.45799949673341800, -12.81261086040661645, 4.791562841999996714 ) ) ;
#22770=CARTESIAN_POINT ( 'NONE',  ( -17.93324555108848628, -9.020011617866936504, 0.000000000000000000 ) ) ;
#22784=CARTESIAN_POINT ( 'NONE',  ( 18.26900987441764812, -9.123954215387964695, -4.336808689942017736E-16 ) ) ;
#22788=B_SPLINE_CURVE_WITH_KNOTS ( 'NONE', 1,
 ( #23909, #30671 ),
 .UNSPECIFIED., .F., .F.,
 ( 2, 2 ),
 ( -2.556819966299999618E-06, 0.7000000000009999335 ),
 .UNSPECIFIED. ) ;
#22797=B_SPLINE_CURVE_WITH_KNOTS ( 'NONE', 3,
 ( #30570, #23648, #9148, #4443, #19222, #30721, #11982, #2245, #6637, #28807, #4756, #18598 ),
 .UNSPECIFIED., .F., .F.,
 ( 4, 2, 2, 2, 2, 4 ),
 ( 0.000000000000000000, 0.2499999999999998335, 0.4999999999999996669, 0.6250000000000000000, 0.7500000000000003331, 1.000000000000000000 ),
 .UNSPECIFIED. ) ;
#22800=CARTESIAN_POINT ( 'NONE',  ( 17.95841148948556310, 10.23646161652002817, 0.000000000000000000 ) ) ;
#22802=CARTESIAN_POINT ( 'NONE',  ( -27.79539923781770483, -0.5057481688778011630, 1.000000000000000888 ) ) ;
#22813=CARTESIAN_POINT ( 'NONE',  ( -28.49528339128749010, -0.5184828350248836815, 8.000000000000007105 ) ) ;
#22817=EDGE_CURVE ( 'NONE', #30998, #25912, #30457, .T. ) ;
#22822=ORIENTED_EDGE ( 'NONE', *, *, #17270, .F. ) ;
#22823=CARTESIAN_POINT ( 'NONE',  ( 24.29089620522634263, 14.90695587088477581, 6.079851352999988023 ) ) ;
#22829=ORIENTED_EDGE ( 'NONE', *, *, #11315, .T. ) ;
#22859=CARTESIAN_POINT ( 'NONE',  ( -0.5944614571882205212, -27.79380703160649446, 4.999998581000003384 ) ) ;
#22866=VERTEX_POINT ( 'NONE', #1940 ) ;
#22869=EDGE_LOOP ( 'NONE', ( #10839, #23186, #2065, #21063, #9162 ) ) ;
#22888=B_SPLINE_CURVE_WITH_KNOTS ( 'NONE', 3,
 ( #14052, #7272, #31036, #28515, #4134, #2091 ),
 .UNSPECIFIED., .F., .F.,
 ( 4, 2, 4 ),
 ( 0.000000000000000000, 0.5000000000000000000, 1.000000000000000000 ),
 .UNSPECIFIED. ) ;
#22893=CARTESIAN_POINT ( 'NONE',  ( 24.49145441566124148, -14.57548795709913847, 4.319167818000013703 ) ) ;
#22902=CARTESIAN_POINT ( 'NONE',  ( 26.60345577955319030, 9.630787818574999548, 0.5514269530000337483 ) ) ;
#22924=CARTESIAN_POINT ( 'NONE',  ( -19.75038721057206104, -20.61365289012606539, 0.02487544599999447215 ) ) ;
#22926=CARTESIAN_POINT ( 'NONE',  ( -23.82471740849593544, -15.64077206322649083, 4.791628272000025390 ) ) ;
#22927=CARTESIAN_POINT ( 'NONE',  ( 25.44662323365202639, -12.83524168329857318, 4.689351482000003735 ) ) ;
#22928=CARTESIAN_POINT ( 'NONE',  ( 2.374791981039476862, 2.610414167372405281, 0.000000000000000000 ) ) ;
#22929=CARTESIAN_POINT ( 'NONE',  ( -27.83860952016654622, 1.869044697291038615, 8.000000000000007105 ) ) ;
#22941=CARTESIAN_POINT ( 'NONE',  ( -19.53673505992006554, -20.39066108913833020, 0.000000000000000000 ) ) ;
#22948=CARTESIAN_POINT ( 'NONE',  ( 18.05835842962944682, -9.659886890379860702, -4.336808689942018722E-16 ) ) ;
#22958=CARTESIAN_POINT ( 'NONE',  ( -17.75159883754878720, -9.616676199626787991, 0.000000000000000000 ) ) ;
#22964=EDGE_CURVE ( 'NONE', #8453, #17781, #1913, .T. ) ;
#22968=CARTESIAN_POINT ( 'NONE',  ( 25.39337327713160519, -12.94027895695280250, 5.560810203903397309 ) ) ;
#22976=CARTESIAN_POINT ( 'NONE',  ( -19.80535397421925481, 19.50875616500616871, 0.9999999989999952543 ) ) ;
#22979=CARTESIAN_POINT ( 'NONE',  ( 24.92980816059056082, 14.06569599973778395, -0.2432540810000105580 ) ) ;
#22983=CARTESIAN_POINT ( 'NONE',  ( 23.82471740507292068, 15.64077205896351508, 5.208368893000026034 ) ) ;
#22991=LINE ( 'NONE', #25353, #20527 ) ;
#23008=VECTOR ( 'NONE', #19277, 1000.000000000000000 ) ;
#23013=AXIS2_PLACEMENT_3D ( 'NONE', #8981, #6782, #9131 ) ;
#23015=CARTESIAN_POINT ( 'NONE',  ( 24.54884435365858053, -13.04717673649832044, 6.002806400000004317 ) ) ;
#23027=ORIENTED_EDGE ( 'NONE', *, *, #10171, .F. ) ;
#23030=ORIENTED_EDGE ( 'NONE', *, *, #22299, .T. ) ;
#23031=CARTESIAN_POINT ( 'NONE',  ( -24.32472894358752313, 13.45989150749028873, 3.899998581000013509 ) ) ;
#23049=CARTESIAN_POINT ( 'NONE',  ( 17.16657240421717390, -9.000000000001264766, -0.6999999999999784173 ) ) ;
#23056=ORIENTED_EDGE ( 'NONE', *, *, #6937, .F. ) ;
#23058=VECTOR ( 'NONE', #30219, 1000.000000000000000 ) ;
#23059=CARTESIAN_POINT ( 'NONE',  ( -24.75645986059670278, -14.12045945564184279, 5.901294544000013076 ) ) ;
#23061=CARTESIAN_POINT ( 'NONE',  ( -23.81866442513186755, -14.33570206443695838, 3.899998581000013509 ) ) ;
#23062=DIRECTION ( 'NONE',  ( 0.000000000000000000, 0.000000000000000000, -1.000000000000000000 ) ) ;
#23068=EDGE_CURVE ( 'NONE', #13449, #2398, #21749, .T. ) ;
#23083=B_SPLINE_CURVE_WITH_KNOTS ( 'NONE', 1,
 ( #22480, #27493 ),
 .UNSPECIFIED., .F., .F.,
 ( 2, 2 ),
 ( -2.556331278550000249E-06, 0.7000000000009999335 ),
 .UNSPECIFIED. ) ;
#23099=EDGE_CURVE ( 'NONE', #15627, #14439, #9944, .T. ) ;
#23113=B_SPLINE_CURVE_WITH_KNOTS ( 'NONE', 3,
 ( #4480, #28077, #11712, #28230, #4326, #21005 ),
 .UNSPECIFIED., .F., .F.,
 ( 4, 2, 4 ),
 ( 0.000000000000000000, 0.5000000000000000000, 1.000000000000000000 ),
 .UNSPECIFIED. ) ;
#23120=EDGE_LOOP ( 'NONE', ( #26901, #711, #15701, #12225 ) ) ;
#23126=CARTESIAN_POINT ( 'NONE',  ( 0.3615961171405600028, -27.79823316426096014, 6.099998580999981712 ) ) ;
#23137=CARTESIAN_POINT ( 'NONE',  ( 28.45300238704230367, 0.5177135156027735663, 0.5017677510000262409 ) ) ;
#23138=CARTESIAN_POINT ( 'NONE',  ( -18.62325121933723437, 19.80375466501974913, 0.06723541799999455115 ) ) ;
#23139=CARTESIAN_POINT ( 'NONE',  ( -14.92487790170366502, -24.58397533831729476, 8.000000000000007105 ) ) ;
#23140=CARTESIAN_POINT ( 'NONE',  ( 16.40303402077768169, -9.791839085275103827, 0.000000000000000000 ) ) ;
#23151=ORIENTED_EDGE ( 'NONE', *, *, #13098, .F. ) ;
#23153=VERTEX_POINT ( 'NONE', #24423 ) ;
#23158=EDGE_CURVE ( 'NONE', #5717, #23153, #20461, .T. ) ;
#23171=CARTESIAN_POINT ( 'NONE',  ( 24.83827472153076599, -12.48687851163286133, 5.104216618000034345 ) ) ;
#23183=CARTESIAN_POINT ( 'NONE',  ( 24.41841038956698640, 14.69667349781389376, 3.899998581000013509 ) ) ;
#23186=ORIENTED_EDGE ( 'NONE', *, *, #27578, .T. ) ;
#23202=CARTESIAN_POINT ( 'NONE',  ( -18.34690887264311243, 20.56908522426308394, -0.5592437529999827461 ) ) ;
#23209=CARTESIAN_POINT ( 'NONE',  ( -28.03861306157277866, -0.5101735396242136344, -0.2432540810000105580 ) ) ;
#23212=CARTESIAN_POINT ( 'NONE',  ( -24.45473033751197178, -14.63622298155413226, 6.098654221000004760 ) ) ;
#23214=CARTESIAN_POINT ( 'NONE',  ( 21.92393651381221886, 17.69663393540654539, 0.8585786549999974149 ) ) ;
#23220=CARTESIAN_POINT ( 'NONE',  ( 24.93720649360215802, -13.79881813812812297, 3.899998581000013509 ) ) ;
#23225=CARTESIAN_POINT ( 'NONE',  ( 3.529820002191843997, -0.01646793578303169109, -0.6999999999999783062 ) ) ;
#23233=VERTEX_POINT ( 'NONE', #11339 ) ;
#23234=CARTESIAN_POINT ( 'NONE',  ( -25.14597776469546631, -15.02549348218341230, 0.8585788009999872905 ) ) ;
#23241=CARTESIAN_POINT ( 'NONE',  ( -3.455601306038264209, -0.7156333712644181722, 0.000000000000000000 ) ) ;
#23246=FACE_BOUND ( 'NONE', #31043, .T. ) ;
#23247=LINE ( 'NONE', #22624, #8750 ) ;
#23255=CARTESIAN_POINT ( 'NONE',  ( -15.73624015665173914, -8.835417945575107623, -0.6999999999999783062 ) ) ;
#23258=CARTESIAN_POINT ( 'NONE',  ( 27.52676963214367944, 0.5008603480904615379, 0.2686740700000300741 ) ) ;
#23259=CARTESIAN_POINT ( 'NONE',  ( -17.59696597926837214, -9.791839085300418688, -0.6999999999999784173 ) ) ;
#23287=CARTESIAN_POINT ( 'NONE',  ( 24.36724931191462318, 13.38201648793565468, 4.854188467883240321 ) ) ;
#23289=CARTESIAN_POINT ( 'NONE',  ( -26.99557660706030049, -9.615007461563203961, 8.000000000000007105 ) ) ;
#23292=CARTESIAN_POINT ( 'NONE',  ( 27.47529052171122288, 5.047756207413780949, -0.5592437529999827461 ) ) ;
#23297=ORIENTED_EDGE ( 'NONE', *, *, #1625, .F. ) ;
#23313=CARTESIAN_POINT ( 'NONE',  ( 24.40022624086872938, 14.72688605419589614, 3.899998581000013509 ) ) ;
#23314=CARTESIAN_POINT ( 'NONE',  ( -23.82471740849593544, -15.64077206322649083, 4.791628272000025390 ) ) ;
#23334=EDGE_CURVE ( 'NONE', #17637, #13449, #20630, .T. ) ;
#23340=CARTESIAN_POINT ( 'NONE',  ( -24.93720648713954446, 13.79881813474513486, 6.099998581000020792 ) ) ;
#23346=ORIENTED_EDGE ( 'NONE', *, *, #21977, .F. ) ;
#23368=CARTESIAN_POINT ( 'NONE',  ( -24.39135169139981940, 14.74223402956394402, 4.689353541000001790 ) ) ;
#23370=CARTESIAN_POINT ( 'NONE',  ( -19.43556844913216608, 20.00000873967102777, -0.3062681690857439465 ) ) ;
#23384=EDGE_CURVE ( 'NONE', #11027, #24538, #12380, .T. ) ;
#23394=CARTESIAN_POINT ( 'NONE',  ( -1.366018022287268430, -3.254826447534360234, -0.6999999999999783062 ) ) ;
#23395=CARTESIAN_POINT ( 'NONE',  ( -23.88745424812704954, 14.22183756790175302, 5.677565560279540513 ) ) ;
#23401=ORIENTED_EDGE ( 'NONE', *, *, #24774, .F. ) ;
#23403=CARTESIAN_POINT ( 'NONE',  ( -25.07108469382532334, -14.98074245159186191, 0.5514273980000150566 ) ) ;
#23414=DIRECTION ( 'NONE',  ( -0.9998345049574558496, -0.01819238017630799703, 0.000000000000000000 ) ) ;
#23423=B_SPLINE_CURVE_WITH_KNOTS ( 'NONE', 3,
 ( #16071, #28181, #13392, #25836, #11045, #10887 ),
 .UNSPECIFIED., .F., .F.,
 ( 4, 2, 4 ),
 ( 0.000000000000000000, 0.5000000000000000000, 1.000000000000000000 ),
 .UNSPECIFIED. ) ;
#23445=CARTESIAN_POINT ( 'NONE',  ( -20.26572724632349320, -21.15151735177849091, 8.000000000000007105 ) ) ;
#23450=CARTESIAN_POINT ( 'NONE',  ( 24.93720649360215802, -13.79881813812812297, 6.099998581000020792 ) ) ;
#23457=CARTESIAN_POINT ( 'NONE',  ( 28.36759364733395472, 5.211690002337984851, 0.5017677510000262409 ) ) ;
#23459=CARTESIAN_POINT ( 'NONE',  ( 0.4024591535043843260, -27.79733476267318437, 3.904047916000019658 ) ) ;
#23463=CARTESIAN_POINT ( 'NONE',  ( -17.77342497899898888, -8.417133906617015882, 0.000000000000000000 ) ) ;
#23466=ORIENTED_EDGE ( 'NONE', *, *, #2303, .F. ) ;
#23475=CARTESIAN_POINT ( 'NONE',  ( 24.21906834310036771, 15.02342240524378703, 3.957526369000014199 ) ) ;
#23479=CARTESIAN_POINT ( 'NONE',  ( 0.5184513693225318853, -28.49550581263314086, 3.899998581000013509 ) ) ;
#23491=CARTESIAN_POINT ( 'NONE',  ( -1.030301836990161535, 20.00000000003602452, -0.6999999999999784173 ) ) ;
#23494=EDGE_CURVE ( 'NONE', #29062, #28672, #27717, .T. ) ;
#23503=CARTESIAN_POINT ( 'NONE',  ( 1.000415564564199444, -28.48292217093161938, 3.997481721999984750 ) ) ;
#23506=CARTESIAN_POINT ( 'NONE',  ( -23.88764392071930587, 14.22151635026485117, 4.322084506810967675 ) ) ;
#23510=ORIENTED_EDGE ( 'NONE', *, *, #24825, .T. ) ;
#23514=CARTESIAN_POINT ( 'NONE',  ( 24.88589369718092215, -13.89120818692358483, 6.095967889000020179 ) ) ;
#23523=FACE_OUTER_BOUND ( 'NONE', #15467, .T. ) ;
#23526=CARTESIAN_POINT ( 'NONE',  ( -19.53717638892995723, 20.00009241111888159, -0.2444329966749828886 ) ) ;
#23538=CARTESIAN_POINT ( 'NONE',  ( 16.08958307952436328, 11.26717219148106786, -0.6999999999999784173 ) ) ;
#23541=CARTESIAN_POINT ( 'NONE',  ( -16.85343921402336775, -7.900182044543379689, -0.6999999999999784173 ) ) ;
#23546=CARTESIAN_POINT ( 'NONE',  ( 3.415131431000496764, 0.8926240808846060970, -0.6999999999999785283 ) ) ;
#23554=CARTESIAN_POINT ( 'NONE',  ( -22.06837820954319440, 15.41983382789281620, 0.000000000000000000 ) ) ;
#23565=CARTESIAN_POINT ( 'NONE',  ( -0.5944614571882205212, -27.79380703160649446, 4.895947184000021046 ) ) ;
#23575=CARTESIAN_POINT ( 'NONE',  ( 17.04261818891856350, -10.10243747014645521, -0.6999999999999783062 ) ) ;
#23590=ORIENTED_EDGE ( 'NONE', *, *, #5663, .T. ) ;
#23608=CARTESIAN_POINT ( 'NONE',  ( 28.35455043824866550, 0.5159221438580675612, 0.2374258030000131470 ) ) ;
#23609=CARTESIAN_POINT ( 'NONE',  ( -17.99585043762395742, 19.96083428726235809, 0.000000000000000000 ) ) ;
#23610=CARTESIAN_POINT ( 'NONE',  ( 23.98155922632636816, -15.68763507556827541, 8.000000000000007105 ) ) ;
#23611=CARTESIAN_POINT ( 'NONE',  ( -17.99585043762395742, 19.96083428726235809, 0.000000000000000000 ) ) ;
#23612=CARTESIAN_POINT ( 'NONE',  ( 27.29371452669260734, 0.4966198192112817322, -0.6577119969999878357 ) ) ;
#23614=CARTESIAN_POINT ( 'NONE',  ( 24.93720649360215802, -13.79881813812812297, 3.899998581000013509 ) ) ;
#23629=CARTESIAN_POINT ( 'NONE',  ( -16.81341597784800967, -10.09981795476353739, 0.000000000000000000 ) ) ;
#23634=CARTESIAN_POINT ( 'NONE',  ( 19.28276787503908452, 20.00015277968180882, -0.3880171390712462420 ) ) ;
#23644=CYLINDRICAL_SURFACE ( 'NONE', #92, 1.100000000000002309 ) ;
#23648=CARTESIAN_POINT ( 'NONE',  ( 24.25496636523650551, -13.58595625263505013, 6.099998581000014575 ) ) ;
#23650=CARTESIAN_POINT ( 'NONE',  ( 0.7459188900473354700, -27.79046661982714639, 6.079790450999988494 ) ) ;
#23655=EDGE_CURVE ( 'NONE', #27389, #2398, #13090, .T. ) ;
#23663=ORIENTED_EDGE ( 'NONE', *, *, #1962, .F. ) ;
#23676=CARTESIAN_POINT ( 'NONE',  ( -20.07475214973380773, 19.99999824547289862, 0.2739201808243049152 ) ) ;
#23704=CARTESIAN_POINT ( 'NONE',  ( 24.83827260360999389, -12.48687744688666967, 4.999998581000003384 ) ) ;
#23710=CARTESIAN_POINT ( 'NONE',  ( -23.39354070940022723, -15.01969650296710768, 4.239862999000004962 ) ) ;
#23720=VECTOR ( 'NONE', #2921, 1000.000000000000000 ) ;
#23724=EDGE_CURVE ( 'NONE', #17896, #18728, #9361, .T. ) ;
#23726=CARTESIAN_POINT ( 'NONE',  ( -28.49530731802708416, -0.5184832703812605192, 8.000000000000007105 ) ) ;
#23730=EDGE_CURVE ( 'NONE', #27396, #28115, #8177, .T. ) ;
#23734=ORIENTED_EDGE ( 'NONE', *, *, #6449, .F. ) ;
#23762=CARTESIAN_POINT ( 'NONE',  ( -19.90432701819680972, 19.99999991336795802, 0.04921632800000685926 ) ) ;
#23769=ORIENTED_EDGE ( 'NONE', *, *, #17676, .T. ) ;
#23783=CARTESIAN_POINT ( 'NONE',  ( 23.81776757409229361, 15.65134803726813217, 4.999998581000003384 ) ) ;
#23785=CARTESIAN_POINT ( 'NONE',  ( 17.95841148951064525, -9.763538383420391042, -0.6999999999999784173 ) ) ;
#23795=CARTESIAN_POINT ( 'NONE',  ( 24.36130769279719033, 13.39283555502935208, 5.208359080000030339 ) ) ;
#23796=CARTESIAN_POINT ( 'NONE',  ( -25.35557883284624481, 13.01417685709828831, 5.679894689235580607 ) ) ;
#23807=CARTESIAN_POINT ( 'NONE',  ( -1.776062861149290062E-14, -3.231615895114969171E-16, -0.5999999999999894307 ) ) ;
#23808=EDGE_LOOP ( 'NONE', ( #28996, #19629, #28174, #25936 ) ) ;
#23809=B_SPLINE_CURVE_WITH_KNOTS ( 'NONE', 5,
 ( #1984, #9197, #20544, #13621, #3702, #1355, #8569, #10949, #25589 ),
 .UNSPECIFIED., .F., .F.,
 ( 6, 3, 6 ),
 ( 0.000000000000000000, 18.06409709749999948, 31.46353197719999883 ),
 .UNSPECIFIED. ) ;
#23820=CARTESIAN_POINT ( 'NONE',  ( 18.26639035967037827, -8.979988381807324060, -1.000005633855494125E-09 ) ) ;
#23822=ORIENTED_EDGE ( 'NONE', *, *, #13915, .T. ) ;
#23829=VERTEX_POINT ( 'NONE', #17238 ) ;
#23836=CARTESIAN_POINT ( 'NONE',  ( 1.645560275461343203, -28.45273235261698019, 4.895940783000013674 ) ) ;
#23840=CARTESIAN_POINT ( 'NONE',  ( 24.36724931188768650, 13.38201648792073684, 4.999998581000003384 ) ) ;
#23841=CARTESIAN_POINT ( 'NONE',  ( 16.06675444873834380, 10.97998838177521286, -0.6999999999999784173 ) ) ;
#23843=ORIENTED_EDGE ( 'NONE', *, *, #3854, .F. ) ;
#23847=VECTOR ( 'NONE', #18371, 1000.000000000000000 ) ;
#23859=CARTESIAN_POINT ( 'NONE',  ( 24.58642410257749233, -12.97641166413832714, 4.035859796549723377 ) ) ;
#23861=ORIENTED_EDGE ( 'NONE', *, *, #5405, .T. ) ;
#23884=CARTESIAN_POINT ( 'NONE',  ( -24.63375100851393640, 12.88633854783081922, 4.098596794000014754 ) ) ;
#23893=CARTESIAN_POINT ( 'NONE',  ( 20.30396079662882158, 20.00000000004802203, 1.000000000000000888 ) ) ;
#23909=CARTESIAN_POINT ( 'NONE',  ( 1.605176535610508326, -27.75389821387976852, 4.999998581000003384 ) ) ;
#23910=CARTESIAN_POINT ( 'NONE',  ( -27.79539923781770128, -0.5057481688779184026, 8.000000000000007105 ) ) ;
#23916=ADVANCED_FACE ( 'NONE', ( #8401 ), #3537, .F. ) ;
#23922=CARTESIAN_POINT ( 'NONE',  ( -19.65670002335123812, 20.00000013293643875, -0.1824558819999988479 ) ) ;
#23937=ORIENTED_EDGE ( 'NONE', *, *, #30240, .F. ) ;
#23940=ORIENTED_EDGE ( 'NONE', *, *, #23099, .T. ) ;
#23947=CARTESIAN_POINT ( 'NONE',  ( 18.02647417827482812, 19.99991602546214153, -0.6955594401470849286 ) ) ;
#23950=DIRECTION ( 'NONE',  ( 0.6941258031311203780, 0.7198537139083029945, 0.000000000000000000 ) ) ;
#23956=DIRECTION ( 'NONE',  ( -0.9998345049574558496, -0.01819238017630799703, 0.000000000000000000 ) ) ;
#23974=CARTESIAN_POINT ( 'NONE',  ( 27.29371452669260734, 0.4966198192113223664, -0.6577119969999878357 ) ) ;
#23980=CARTESIAN_POINT ( 'NONE',  ( 18.31101511981528773, 19.88193408480103486, 0.02162463700000616385 ) ) ;
#23987=B_SPLINE_CURVE_WITH_KNOTS ( 'NONE', 3,
 ( #13198, #20603, #12904, #18073, #22512, #20447 ),
 .UNSPECIFIED., .F., .F.,
 ( 4, 2, 4 ),
 ( 0.000000000000000000, 0.5000000000000000000, 1.000000000000000000 ),
 .UNSPECIFIED. ) ;
#24002=CARTESIAN_POINT ( 'NONE',  ( -27.24406355354254217, -0.4957164003246626316, 0.08279779300002232389 ) ) ;
#24009=CARTESIAN_POINT ( 'NONE',  ( -24.32472894358752313, 13.45989150749028873, 3.899998581000013509 ) ) ;
#24016=CARTESIAN_POINT ( 'NONE',  ( -20.30403093138962234, 20.00000000003553424, 1.000000000000000888 ) ) ;
#24017=CARTESIAN_POINT ( 'NONE',  ( -19.80535397421925481, 19.50875616500616871, 0.9999999989999952543 ) ) ;
#24022=CYLINDRICAL_SURFACE ( 'NONE', #17496, 3.500000000000003109 ) ;
#24026=CARTESIAN_POINT ( 'NONE',  ( 22.97559295455008765, 15.65128684778802715, 8.000000000000007105 ) ) ;
#24030=CARTESIAN_POINT ( 'NONE',  ( -25.45799949038170240, 12.81261085762170815, 4.791562840999991302 ) ) ;
#24031=CARTESIAN_POINT ( 'NONE',  ( 17.16657240419154462, 10.99999999996915179, -0.6999999999999784173 ) ) ;
#24035=ORIENTED_EDGE ( 'NONE', *, *, #11785, .T. ) ;
#24053=CARTESIAN_POINT ( 'NONE',  ( -27.07233438391262226, 8.380005029826659069, 5.200000000000009948 ) ) ;
#24056=CARTESIAN_POINT ( 'NONE',  ( -4.667733413567799694, -30.93201666733562405, 8.000000000000007105 ) ) ;
#24057=CARTESIAN_POINT ( 'NONE',  ( -19.80535357377644701, 19.50875577052588739, 2.200000064000007249 ) ) ;
#24062=AXIS2_PLACEMENT_3D ( 'NONE', #20953, #14500, #13875 ) ;
#24066=CARTESIAN_POINT ( 'NONE',  ( 24.78870453580057998, -12.58522324566301620, 5.507123706999989210 ) ) ;
#24069=CARTESIAN_POINT ( 'NONE',  ( -19.36598219300702794, 19.99999980947656297, -0.3593759589999856452 ) ) ;
#24075=FACE_OUTER_BOUND ( 'NONE', #22560, .T. ) ;
#24084=ORIENTED_EDGE ( 'NONE', *, *, #5934, .T. ) ;
#24089=CARTESIAN_POINT ( 'NONE',  ( 14.25032083441342934, -27.35421241409322946, 1.000000000000000888 ) ) ;
#24090=CARTESIAN_POINT ( 'NONE',  ( 27.79539923781924315, 0.5057481687932959824, 8.000000000000007105 ) ) ;
#24093=CARTESIAN_POINT ( 'NONE',  ( 18.56971040771836101, 20.00001258923172998, -0.6273519244159778685 ) ) ;
#24094=CARTESIAN_POINT ( 'NONE',  ( -23.77947513073445407, 14.40125622634048774, 5.208432825000025801 ) ) ;
#24097=CARTESIAN_POINT ( 'NONE',  ( 17.33054985591605757, -10.09719844076225215, -4.336808689942018722E-16 ) ) ;
#24101=CARTESIAN_POINT ( 'NONE',  ( 0.7153897335033406746, -3.455736562763356279, 0.000000000000000000 ) ) ;
#24103=CARTESIAN_POINT ( 'NONE',  ( 24.41841038956698640, 14.69667349781389376, 6.099998581000020792 ) ) ;
#24108=CARTESIAN_POINT ( 'NONE',  ( -24.22405393111852234, -13.63981656674930854, 4.239871886000001311 ) ) ;
#24113=LINE ( 'NONE', #12601, #4221 ) ;
#24118=CARTESIAN_POINT ( 'NONE',  ( 23.81776757409229361, 15.65134803726813217, 4.999998581000003384 ) ) ;
#24127=CARTESIAN_POINT ( 'NONE',  ( -25.46368746804859740, 12.80129684245613575, 4.999998581000003384 ) ) ;
#24133=CARTESIAN_POINT ( 'NONE',  ( -18.33647963386089685, 19.99999869789418128, -0.6670195793833753051 ) ) ;
#24141=CYLINDRICAL_SURFACE ( 'NONE', #29534, 1.099999999999999867 ) ;
#24150=ADVANCED_FACE ( 'NONE', ( #16126 ), #4632, .F. ) ;
#24151=ORIENTED_EDGE ( 'NONE', *, *, #9169, .F. ) ;
#24153=( NAMED_UNIT ( * ) PLANE_ANGLE_UNIT ( ) SI_UNIT ( $, .RADIAN. ) );
#24162=CARTESIAN_POINT ( 'NONE',  ( -23.81866173682177390, -14.33570044646243247, 3.899998581000013509 ) ) ;
#24170=EDGE_CURVE ( 'NONE', #11464, #27319, #25085, .T. ) ;
#24177=CARTESIAN_POINT ( 'NONE',  ( 23.89355638714178198, 14.21126451599432272, 3.899998580999974873 ) ) ;
#24179=CARTESIAN_POINT ( 'NONE',  ( -24.73568147689076469, 12.68911064935910815, 4.319165764000016061 ) ) ;
#24183=CARTESIAN_POINT ( 'NONE',  ( -16.14308042027219869, -8.142661250102314341, 0.000000000000000000 ) ) ;
#24187=CARTESIAN_POINT ( 'NONE',  ( 19.80526555972147307, 19.50877392102524155, 3.000000000000002665 ) ) ;
#24197=CARTESIAN_POINT ( 'NONE',  ( -16.52704821365513510, -10.06576768835640046, -0.6999999999999785283 ) ) ;
#24203=FACE_OUTER_BOUND ( 'NONE', #25359, .T. ) ;
#24212=CARTESIAN_POINT ( 'NONE',  ( -15.96459051030187126, 11.69027953513920437, -0.6999999999999784173 ) ) ;
#24213=CARTESIAN_POINT ( 'NONE',  ( -18.62325121933723437, 19.80375466501974913, 0.06723541799999455115 ) ) ;
#24215=CARTESIAN_POINT ( 'NONE',  ( -15.76747295634271495, 11.30736579152925003, -4.336808689942018722E-16 ) ) ;
#24233=CARTESIAN_POINT ( 'NONE',  ( 17.93011078763067090, 11.79183908526299085, -0.6999999999999784173 ) ) ;
#24236=CARTESIAN_POINT ( 'NONE',  ( 19.13554320545159371, 20.00034038933170422, -0.4554370248835840629 ) ) ;
#24237=CARTESIAN_POINT ( 'NONE',  ( -24.14205448738587023, 13.78537896750705194, 6.042507811999997536 ) ) ;
#24240=CARTESIAN_POINT ( 'NONE',  ( -25.96688743241739061, 8.776138983998601262, -0.6999999999999784173 ) ) ;
#24241=VERTEX_POINT ( 'NONE', #12025 ) ;
#24247=CARTESIAN_POINT ( 'NONE',  ( 20.28766220345061910, 20.00000013976770674, 0.7460156100000114865 ) ) ;
#24254=ORIENTED_EDGE ( 'NONE', *, *, #20097, .T. ) ;
#24261=CARTESIAN_POINT ( 'NONE',  ( -16.26054471415775993, 10.04965037057037236, -0.6999999999999784173 ) ) ;
#24271=CARTESIAN_POINT ( 'NONE',  ( 18.23252704342300845, -8.692634207812194092, -4.336808689942018722E-16 ) ) ;
#24276=CARTESIAN_POINT ( 'NONE',  ( 19.29866511436280874, 19.63492491799039996, 0.3046098590000212436 ) ) ;
#24278=ORIENTED_EDGE ( 'NONE', *, *, #17060, .T. ) ;
#24281=VECTOR ( 'NONE', #10259, 1000.000000000000000 ) ;
#24287=CARTESIAN_POINT ( 'NONE',  ( -24.77402022478258914, 12.61404137177703433, 4.439986940269814220 ) ) ;
#24296=CARTESIAN_POINT ( 'NONE',  ( -27.77052805885498898, -0.5052956280874019157, 0.7069222069999991920 ) ) ;
#24299=ORIENTED_EDGE ( 'NONE', *, *, #14130, .T. ) ;
#24304=ORIENTED_EDGE ( 'NONE', *, *, #20256, .T. ) ;
#24306=CARTESIAN_POINT ( 'NONE',  ( 0.6090474298383116158, -27.79358669172298946, 3.904048352000033528 ) ) ;
#24333=CARTESIAN_POINT ( 'NONE',  ( -4.540209229552565340, -30.08687099007853405, -0.6999999999999784173 ) ) ;
#24339=DIRECTION ( 'NONE',  ( 0.000000000000000000, 0.000000000000000000, -1.000000000000000000 ) ) ;
#24341=STYLED_ITEM ( 'NONE', ( #21484 ), #18548 ) ;
#24357=CARTESIAN_POINT ( 'NONE',  ( -22.90527192528401201, 16.36193184990112570, 3.799999999999998046 ) ) ;
#24365=CARTESIAN_POINT ( 'NONE',  ( -24.75645986059852177, -14.12045945554185522, 4.098702617000016701 ) ) ;
#24367=CARTESIAN_POINT ( 'NONE',  ( 28.47939442936984733, 1.391723841383464277, 8.000000000000007105 ) ) ;
#24369=B_SPLINE_SURFACE_WITH_KNOTS ( 'NONE', 5, 1, ( 
 ( #17316, #14359 ),
 ( #9778, #26923 ),
 ( #24247, #16855 ),
 ( #5359, #3000 ),
 ( #12592, #11978 ),
 ( #21590, #38 ),
 ( #19219, #28801 ),
 ( #7264, #26460 ),
 ( #28968, #7411 ),
 ( #13365, #961 ),
 ( #15114, #15563 ),
 ( #8018, #19846 ),
 ( #18074, #3774 ),
 ( #7862, #8319 ),
 ( #17465, #10551 ) ),
 .UNSPECIFIED., .F., .F., .F.,
 ( 6, 3, 3, 3, 6 ),
 ( 2, 2 ),
 ( 0.000000000000000000, 0.5777945772229999832, 1.155589154450000100, 2.022281020279999897, 2.888972886109999916 ),
 ( 6.550315845290000521E-15, 0.7031438909409999383 ),
 .UNSPECIFIED. ) ;
#24396=FACE_OUTER_BOUND ( 'NONE', #16367, .T. ) ;
#24397=CARTESIAN_POINT ( 'NONE',  ( -16.81341597756113515, 9.900182044522454206, -0.6999999999999784173 ) ) ;
#24398=DIRECTION ( 'NONE',  ( -0.7198537139083028835, 0.6941258031311204890, 0.000000000000000000 ) ) ;
#24401=CARTESIAN_POINT ( 'NONE',  ( -22.97593529893700648, 15.65128280014837081, 8.000000000000007105 ) ) ;
#24403=CARTESIAN_POINT ( 'NONE',  ( -17.59696597919420213, 10.20816091468181774, -0.6999999999999784173 ) ) ;
#24404=ORIENTED_EDGE ( 'NONE', *, *, #27456, .T. ) ;
#24415=B_SPLINE_CURVE_WITH_KNOTS ( 'NONE', 3,
 ( #18859, #6433, #20596, #25800, #25648, #4078 ),
 .UNSPECIFIED., .F., .F.,
 ( 4, 2, 4 ),
 ( 0.000000000000000000, 0.5000000000000000000, 1.000000000000000000 ),
 .UNSPECIFIED. ) ;
#24416=CARTESIAN_POINT ( 'NONE',  ( 1.605176535610508326, -27.75389821387976852, 5.104056378000016103 ) ) ;
#24417=CARTESIAN_POINT ( 'NONE',  ( -24.54452542612009225, -14.48555670042145138, 3.920144560000005107 ) ) ;
#24420=CARTESIAN_POINT ( 'NONE',  ( 18.23234009198083072, -8.693620616447864435, -0.6999999999999785283 ) ) ;
#24423=CARTESIAN_POINT ( 'NONE',  ( 3.040504021322313122, 1.733590290792417887, -0.6999999999999784173 ) ) ;
#24434=CARTESIAN_POINT ( 'NONE',  ( 16.89818815126293217, 9.923569363153179168, -0.6999999999999785283 ) ) ;
#24436=CARTESIAN_POINT ( 'NONE',  ( -24.70448872506469229, 12.74983733322420321, 5.760266710000017554 ) ) ;
#24437=CARTESIAN_POINT ( 'NONE',  ( 28.35945635826399780, 7.983396865336832349, 1.000000000000000888 ) ) ;
#24445=CARTESIAN_POINT ( 'NONE',  ( 18.26639035967037827, -8.979988381807324060, -0.6999999999999784173 ) ) ;
#24449=CARTESIAN_POINT ( 'NONE',  ( -24.83828966697487317, 12.48688602537153791, 4.853901705271463030 ) ) ;
#24452=CARTESIAN_POINT ( 'NONE',  ( 1.645560275461343203, -28.45273235261698019, 4.999998581000003384 ) ) ;
#24458=CARTESIAN_POINT ( 'NONE',  ( -17.83930458829795640, 19.99999999999961631, 0.000000000000000000 ) ) ;
#24464=B_SPLINE_SURFACE_WITH_KNOTS ( 'NONE', 5, 5, ( 
 ( #13204, #1108, #22662, #17918, #25177, #27528, #5974, #10868, #13371 ),
 ( #29741, #15420, #18234, #3610, #15894, #18404, #27682, #6130, #20608 ),
 ( #3780, #25025, #5668, #5822, #22979, #30206, #6294, #25497, #27383 ),
 ( #11171, #16048, #18713, #25964, #11486, #30532, #21089, #16355, #28161 ),
 ( #18561, #30836, #28003, #23292, #4400, #14005, #23457, #4252, #13847 ),
 ( #1889, #25813, #23612, #4556, #11638, #11332, #2048, #25660, #14157 ) ),
 .UNSPECIFIED., .F., .F., .F.,
 ( 6, 6 ),
 ( 6, 3, 6 ),
 ( 65.40639850639999509, 88.68172752359998867 ),
 ( 8.011061266649999624, 9.371850724429998891, 10.73264018220000082 ),
 .UNSPECIFIED. ) ;
#24469=ORIENTED_EDGE ( 'NONE', *, *, #6937, .T. ) ;
#24471=EDGE_CURVE ( 'NONE', #7965, #25224, #25483, .T. ) ;
#24481=CARTESIAN_POINT ( 'NONE',  ( -24.98081131316241255, -13.71897606304888662, 4.999998581000003384 ) ) ;
#24483=CARTESIAN_POINT ( 'NONE',  ( -27.75400871128895375, 8.590834169133980680, 1.000000000000000888 ) ) ;
#24487=CARTESIAN_POINT ( 'NONE',  ( -4.627881920500872326, -30.66785676076818490, -0.5592437529999827461 ) ) ;
#24489=CARTESIAN_POINT ( 'NONE',  ( 23.77307140678977504, -14.41181874416537134, 4.895781291000017355 ) ) ;
#24508=CARTESIAN_POINT ( 'NONE',  ( -16.81341597763548990, -10.09981795544978311, -0.6999999999999784173 ) ) ;
#24509=CARTESIAN_POINT ( 'NONE',  ( -22.90527192528401201, 16.36193184990112570, 2.400000000000013234 ) ) ;
#24514=CARTESIAN_POINT ( 'NONE',  ( 24.54884435365858053, -13.04717673649832044, 6.002806400000004317 ) ) ;
#24516=CARTESIAN_POINT ( 'NONE',  ( 27.98121187870611593, -9.706323496128696604, 8.000000000000007105 ) ) ;
#24519=CARTESIAN_POINT ( 'NONE',  ( 24.54452541844319668, 14.48555669908156851, 3.920144559000027229 ) ) ;
#24538=VERTEX_POINT ( 'NONE', #2087 ) ;
#24539=CARTESIAN_POINT ( 'NONE',  ( 24.82162974202869421, -12.51998933900577349, 4.689351482000003735 ) ) ;
#24541=EDGE_LOOP ( 'NONE', ( #21793, #7692, #15693, #5116 ) ) ;
#24542=ORIENTED_EDGE ( 'NONE', *, *, #2234, .T. ) ;
#24544=EDGE_LOOP ( 'NONE', ( #19815, #8974, #818, #17889, #15205 ) ) ;
#24566=CARTESIAN_POINT ( 'NONE',  ( -17.93324555128263142, -9.020011618190519442, -0.6999999999999784173 ) ) ;
#24574=CARTESIAN_POINT ( 'NONE',  ( 1.533144572060379796, -28.45911136072525238, 4.493506933999996455 ) ) ;
#24577=CARTESIAN_POINT ( 'NONE',  ( 26.87806031854113087, 10.31605756234181115, 8.000000000000007105 ) ) ;
#24587=CARTESIAN_POINT ( 'NONE',  ( 16.37473331892315542, -8.236461616552139375, -0.6999999999999784173 ) ) ;
#24589=CARTESIAN_POINT ( 'NONE',  ( -24.78871709450119809, 12.58522962245461585, 5.507123707999994622 ) ) ;
#24591=CARTESIAN_POINT ( 'NONE',  ( -23.96314403019941608, -14.09350462245096125, 6.073177660868579686 ) ) ;
#24611=CARTESIAN_POINT ( 'NONE',  ( -21.38751961657293066, 17.02472927140214054, 0.000000000000000000 ) ) ;
#24623=CARTESIAN_POINT ( 'NONE',  ( -27.55801272791059731, -0.5014288284349446290, -0.5592437529999827461 ) ) ;
#24640=CARTESIAN_POINT ( 'NONE',  ( -24.45890872495081680, -14.61494978185785421, -0.6999999999999784173 ) ) ;
#24647=CARTESIAN_POINT ( 'NONE',  ( 0.5184513693225726305, -28.49550581263314086, 6.099998581000020792 ) ) ;
#24656=CARTESIAN_POINT ( 'NONE',  ( -4.499842235593497719, -29.81936866046843093, 0.000000000000000000 ) ) ;
#24665=CARTESIAN_POINT ( 'NONE',  ( 24.83827472153076599, -12.48687851163286133, 4.999998581000003384 ) ) ;
#24678=EDGE_CURVE ( 'NONE', #13797, #11577, #21301, .T. ) ;
#24689=ORIENTED_EDGE ( 'NONE', *, *, #4045, .F. ) ;
#24694=B_SPLINE_CURVE_WITH_KNOTS ( 'NONE', 5,
 ( #3377, #12982, #29190, #2776, #12367, #21976, #6527, #3857, #27932 ),
 .UNSPECIFIED., .F., .F.,
 ( 6, 3, 6 ),
 ( 0.000000000000000000, 0.7281981308589999813, 1.224410036190000106 ),
 .UNSPECIFIED. ) ;
#24696=CARTESIAN_POINT ( 'NONE',  ( 16.37473331892315542, -8.236461616552139375, 0.000000000000000000 ) ) ;
#24697=CARTESIAN_POINT ( 'NONE',  ( -17.89938223473397017, 10.69263420681399346, -0.6999999999999784173 ) ) ;
#24704=CARTESIAN_POINT ( 'NONE',  ( -22.36193249936582816, 17.71394520520996707, 6.000000042999998229 ) ) ;
#24710=CARTESIAN_POINT ( 'NONE',  ( 24.90302311548996883, -13.86047864964742793, 6.098655051000018368 ) ) ;
#24716=CARTESIAN_POINT ( 'NONE',  ( -28.49528339128749366, -0.5184828350247674411, 1.000000000000000888 ) ) ;
#24723=ORIENTED_EDGE ( 'NONE', *, *, #2240, .T. ) ;
#24734=EDGE_CURVE ( 'NONE', #4633, #19859, #25024, .T. ) ;
#24735=CARTESIAN_POINT ( 'NONE',  ( -16.17397428794474479, 11.89215903497504456, -0.6999999999999783062 ) ) ;
#24736=CARTESIAN_POINT ( 'NONE',  ( 16.06409288148108416, -8.873734595567666972, -0.6999999999999784173 ) ) ;
#24742=CARTESIAN_POINT ( 'NONE',  ( -24.15628151204887786, -13.75958218676210087, 5.886532584766007936 ) ) ;
#24769=ORIENTED_EDGE ( 'NONE', *, *, #22408, .F. ) ;
#24771=CARTESIAN_POINT ( 'NONE',  ( 23.23277125981546476, 15.26692728828886025, 5.104183903999998329 ) ) ;
#24774=EDGE_CURVE ( 'NONE', #13449, #9797, #14163, .T. ) ;
#24776=CARTESIAN_POINT ( 'NONE',  ( -28.49528339128749366, -0.5184828350247461248, 1.000000000000000888 ) ) ;
#24782=CARTESIAN_POINT ( 'NONE',  ( 24.92013865993870425, -13.82966158318416738, 3.899998581000013509 ) ) ;
#24787=CARTESIAN_POINT ( 'NONE',  ( -24.31416968206321627, -13.47842985394946780, 5.506973469000003618 ) ) ;
#24793=CARTESIAN_POINT ( 'NONE',  ( 24.06826093652101051, -20.50742065841456707, 1.000000000000000888 ) ) ;
#24802=CARTESIAN_POINT ( 'NONE',  ( 3.267430459712248325, 1.335589245137589254, -0.6999999999999783062 ) ) ;
#24810=CARTESIAN_POINT ( 'NONE',  ( 23.47715715125384861, -20.00370206677004958, 0.8585801419999927742 ) ) ;
#24818=UNCERTAINTY_MEASURE_WITH_UNIT (LENGTH_MEASURE( 1.000000000000000082E-05 ), #13550, 'distance_accuracy_value', 'NONE');
#24820=CARTESIAN_POINT ( 'NONE',  ( -23.55444264242456498, 16.04540112444970390, 8.000000000000007105 ) ) ;
#24821=CARTESIAN_POINT ( 'NONE',  ( 24.35797964201644561, -13.39969403546014703, 6.098655031999994591 ) ) ;
#24825=EDGE_CURVE ( 'NONE', #8453, #7951, #15656, .T. ) ;
#24826=CARTESIAN_POINT ( 'NONE',  ( -24.43659368756648576, -14.66646236829179450, 3.899998581000013509 ) ) ;
#24827=EDGE_CURVE ( 'NONE', #6068, #30855, #8512, .T. ) ;
#24830=CARTESIAN_POINT ( 'NONE',  ( -16.04158851046123502, 10.23646161653652875, 0.000000000000000000 ) ) ;
#24843=ORIENTED_EDGE ( 'NONE', *, *, #27337, .F. ) ;
#24847=ORIENTED_EDGE ( 'NONE', *, *, #19642, .F. ) ;
#24853=VERTEX_POINT ( 'NONE', #20611 ) ;
#24855=MECHANICAL_DESIGN_GEOMETRIC_PRESENTATION_REPRESENTATION('',(#24341),#9787);
#24857=CARTESIAN_POINT ( 'NONE',  ( 24.36130769279719033, 13.39283555502935208, 4.791638082000004850 ) ) ;
#24858=EDGE_CURVE ( 'NONE', #13946, #30352, #21692, .T. ) ;
#24867=CARTESIAN_POINT ( 'NONE',  ( -18.39373989079361138, 20.00001178696177462, -0.6589525304462929833 ) ) ;
#24878=CARTESIAN_POINT ( 'NONE',  ( 22.36170820408901960, 17.71391973664089292, 6.000000000000005329 ) ) ;
#24881=CARTESIAN_POINT ( 'NONE',  ( 23.81776757409229361, 15.65134803726813217, 4.999998581000003384 ) ) ;
#24885=CARTESIAN_POINT ( 'NONE',  ( 16.06675444876397307, -9.020011618195203695, -0.6999999989999727834 ) ) ;
#24893=VERTEX_POINT ( 'NONE', #23614 ) ;
#24901=CARTESIAN_POINT ( 'NONE',  ( 19.80526555962148549, 19.50877392102342256, 1.000000000000000888 ) ) ;
#24913=CARTESIAN_POINT ( 'NONE',  ( 2.813577582285908818, 2.131591337306447453, -0.6999999999999784173 ) ) ;
#24920=CARTESIAN_POINT ( 'NONE',  ( -26.91170281299162426, 9.095659093862945355, 0.7069222149999887517 ) ) ;
#24927=CARTESIAN_POINT ( 'NONE',  ( -24.74993094845043018, 14.13250375615880117, 3.957489350000009676 ) ) ;
#24931=CARTESIAN_POINT ( 'NONE',  ( 1.615442258875288362, -28.45452079205452733, 5.290483759618271442 ) ) ;
#24941=CARTESIAN_POINT ( 'NONE',  ( -24.43659368756648576, -14.66646236829179450, 6.099998581000020792 ) ) ;
#24950=CARTESIAN_POINT ( 'NONE',  ( 17.29052662034098020, 12.10243747006436799, 1.385610376436474667E-13 ) ) ;
#24954=CARTESIAN_POINT ( 'NONE',  ( -0.3076636919214117971, -28.49867017228250177, 5.759626916000016195 ) ) ;
#24955=ORIENTED_EDGE ( 'NONE', *, *, #25435, .T. ) ;
#24963=CARTESIAN_POINT ( 'NONE',  ( 22.63260994176697238, -19.28417101125922883, 0.000000000000000000 ) ) ;
#24970=CARTESIAN_POINT ( 'NONE',  ( 25.46368747440213198, -12.80129684534102807, 4.999998581000003384 ) ) ;
#25002=CARTESIAN_POINT ( 'NONE',  ( 24.47278418934676836, 14.60601539428441598, 3.904031772999999816 ) ) ;
#25011=EDGE_LOOP ( 'NONE', ( #26323, #25712, #12678, #23346 ) ) ;
#25016=EDGE_CURVE ( 'NONE', #16634, #6458, #18272, .T. ) ;
#25019=CARTESIAN_POINT ( 'NONE',  ( 28.68577476828162531, -9.950727360111285336, 1.000000000000000888 ) ) ;
#25024=B_SPLINE_CURVE_WITH_KNOTS ( 'NONE', 5,
 ( #8170, #13206, #10701, #3153, #966, #17772, #5670, #5823, #15422 ),
 .UNSPECIFIED., .F., .F.,
 ( 6, 3, 6 ),
 ( 67.22752578339999729, 77.81866039000000512, 88.40979499649999696 ),
 .UNSPECIFIED. ) ;
#25025=CARTESIAN_POINT ( 'NONE',  ( 24.03830838765967925, 13.56270118689358206, -0.6999999999999784173 ) ) ;
#25027=CARTESIAN_POINT ( 'NONE',  ( 20.30396079662882158, 20.00000000004802203, 3.000000000000002665 ) ) ;
#25029=ORIENTED_EDGE ( 'NONE', *, *, #27492, .T. ) ;
#25031=CARTESIAN_POINT ( 'NONE',  ( 18.26639035967037827, -8.979988381807324060, -1.000005633855494125E-09 ) ) ;
#25035=LINE ( 'NONE', #29749, #30819 ) ;
#25041=ORIENTED_EDGE ( 'NONE', *, *, #3341, .F. ) ;
#25051=CARTESIAN_POINT ( 'NONE',  ( 24.25493619443923876, -13.58601077461538509, 3.899998581000038378 ) ) ;
#25062=EDGE_CURVE ( 'NONE', #3709, #19797, #22417, .T. ) ;
#25068=CARTESIAN_POINT ( 'NONE',  ( -24.12437076912601341, -15.17512416476963111, 5.965434395632247977 ) ) ;
#25079=CARTESIAN_POINT ( 'NONE',  ( -24.93720648713954446, 13.79881813474513486, 3.899998581000013509 ) ) ;
#25085=B_SPLINE_CURVE_WITH_KNOTS ( 'NONE', 3,
 ( #1821, #21013, #30617, #23538, #25896, #23841 ),
 .UNSPECIFIED., .F., .F.,
 ( 4, 2, 4 ),
 ( 0.000000000000000000, 0.5000000000000000000, 1.000000000000000000 ),
 .UNSPECIFIED. ) ;
#25086=CARTESIAN_POINT ( 'NONE',  ( -27.12080906453036278, 4.172318231302202030, -0.6999999999999784173 ) ) ;
#25089=CARTESIAN_POINT ( 'NONE',  ( -25.35851007062240114, 13.00862288638852959, 4.319165764000016061 ) ) ;
#25098=CARTESIAN_POINT ( 'NONE',  ( -23.87170005649112525, -14.24726900567271493, 6.095965388000001539 ) ) ;
#25100=CARTESIAN_POINT ( 'NONE',  ( 27.79539923781770483, 0.5057481688777786255, 0.8585786439999909536 ) ) ;
#25107=CARTESIAN_POINT ( 'NONE',  ( 23.79228474585360686, -14.38012950158411662, 4.689353541000001790 ) ) ;
#25111=B_SPLINE_CURVE_WITH_KNOTS ( 'NONE', 1,
 ( #18835, #28128 ),
 .UNSPECIFIED., .F., .F.,
 ( 2, 2 ),
 ( -2.557514682700000071E-06, 0.7000000000009999335 ),
 .UNSPECIFIED. ) ;
#25120=CARTESIAN_POINT ( 'NONE',  ( -19.53673505992006554, -20.39066108913833020, 0.000000000000000000 ) ) ;
#25121=ORIENTED_EDGE ( 'NONE', *, *, #22699, .T. ) ;
#25130=FACE_OUTER_BOUND ( 'NONE', #24544, .T. ) ;
#25131=DIRECTION ( 'NONE',  ( 0.000000000000000000, 0.000000000000000000, -1.000000000000000000 ) ) ;
#25153=ORIENTED_EDGE ( 'NONE', *, *, #22132, .T. ) ;
#25156=ORIENTED_EDGE ( 'NONE', *, *, #8459, .T. ) ;
#25177=CARTESIAN_POINT ( 'NONE',  ( 18.66688021548718979, 20.92780155529449715, -0.2432540810000105580 ) ) ;
#25182=CARTESIAN_POINT ( 'NONE',  ( 23.83861932470720291, 15.61961844235199948, 5.310552110000033466 ) ) ;
#25199=CARTESIAN_POINT ( 'NONE',  ( -24.54885679033566248, 13.04718334763902199, 6.002806401000010617 ) ) ;
#25209=CARTESIAN_POINT ( 'NONE',  ( 24.36724931191508858, 13.38201648793566889, 5.145839562916747489 ) ) ;
#25214=CARTESIAN_POINT ( 'NONE',  ( -28.49528339128749366, -0.5184828350247674411, 1.000000000000000888 ) ) ;
#25223=CARTESIAN_POINT ( 'NONE',  ( -23.90286779622075741, -15.52112778363645340, 5.560535487288766454 ) ) ;
#25224=VERTEX_POINT ( 'NONE', #25628 ) ;
#25227=VERTEX_POINT ( 'NONE', #1549 ) ;
#25229=CARTESIAN_POINT ( 'NONE',  ( -24.05205707537934856, 13.94194077903211593, 4.038530408134264782 ) ) ;
#25230=CARTESIAN_POINT ( 'NONE',  ( 23.81866167241657806, 14.33570040768432996, 3.899998581000013509 ) ) ;
#25231=VERTEX_POINT ( 'NONE', #23259 ) ;
#25244=CARTESIAN_POINT ( 'NONE',  ( -28.54231846005005835, 4.391006012848424511, 0.5017677510000262409 ) ) ;
#25251=CARTESIAN_POINT ( 'NONE',  ( 16.59519732805809156, -8.049072271192613925, -4.336808689942017243E-16 ) ) ;
#25258=CARTESIAN_POINT ( 'NONE',  ( 18.44984352795534832, 20.68448143878967826, 0.5514271650000068803 ) ) ;
#25267=CARTESIAN_POINT ( 'NONE',  ( 0.8926240813841433974, -3.415131430869944307, -0.6999999999999784173 ) ) ;
#25272=EDGE_CURVE ( 'NONE', #29062, #17095, #30656, .T. ) ;
#25277=ORIENTED_EDGE ( 'NONE', *, *, #15798, .T. ) ;
#25278=EDGE_CURVE ( 'NONE', #20192, #23233, #27252, .T. ) ;
#25279=CARTESIAN_POINT ( 'NONE',  ( -4.549046388969006038, -30.14545866191155810, 0.02487508500001456291 ) ) ;
#25281=VERTEX_POINT ( 'NONE', #16165 ) ;
#25284=CARTESIAN_POINT ( 'NONE',  ( -3.063912144317538111, 1.789060389098976911, 0.000000000000000000 ) ) ;
#25289=CARTESIAN_POINT ( 'NONE',  ( 28.49528339128749366, 0.5184828350247835393, 8.000000000000007105 ) ) ;
#25318=CARTESIAN_POINT ( 'NONE',  ( 24.34942395458080000, 13.41447635809142724, 4.689458287000014991 ) ) ;
#25323=CARTESIAN_POINT ( 'NONE',  ( -17.14079338756361892, 12.06595463930550238, -4.336808689942018722E-16 ) ) ;
#25327=VERTEX_POINT ( 'NONE', #27811 ) ;
#25335=CARTESIAN_POINT ( 'NONE',  ( -27.90784132687080898, -6.416341681828127363, 8.000000000000007105 ) ) ;
#25353=CARTESIAN_POINT ( 'NONE',  ( -16.85343921402336775, -7.900182044543379689, -0.6999999989999727834 ) ) ;
#25359=EDGE_LOOP ( 'NONE', ( #11430, #7046, #10306, #25029 ) ) ;
#25370=CARTESIAN_POINT ( 'NONE',  ( 23.99428763615714644, -14.04082805276427592, 4.114052333822514562 ) ) ;
#25376=CARTESIAN_POINT ( 'NONE',  ( 24.83272649506304219, -12.49791454618707398, 5.208434320000010942 ) ) ;
#25380=CARTESIAN_POINT ( 'NONE',  ( 17.73945528731000110, 10.04965037119602655, -0.6999999999999784173 ) ) ;
#25382=CARTESIAN_POINT ( 'NONE',  ( -17.78291068004000053, 10.42683423967575251, -0.000000000000000000 ) ) ;
#25387=CARTESIAN_POINT ( 'NONE',  ( -24.06001628199535247, -15.27670956567710192, 5.888744255995201904 ) ) ;
#25402=VECTOR ( 'NONE', #1137, 1000.000000000000000 ) ;
#25415=EDGE_CURVE ( 'NONE', #8936, #21696, #27632, .T. ) ;
#25418=PRODUCT ( 'Rear Frame Plate', 'Rear Frame Plate', '', ( #27981 ) ) ;
#25420=ORIENTED_EDGE ( 'NONE', *, *, #3808, .T. ) ;
#25422=CARTESIAN_POINT ( 'NONE',  ( -24.14840830027149465, -13.77363891140888619, 5.901294544000013076 ) ) ;
#25424=CARTESIAN_POINT ( 'NONE',  ( 27.71261514784184499, 0.5042418799608394675, 0.5514269430000329208 ) ) ;
#25431=VERTEX_POINT ( 'NONE', #28901 ) ;
#25432=CARTESIAN_POINT ( 'NONE',  ( 23.83006841374216833, -14.31758446293960141, 4.492876031999992748 ) ) ;
#25435=EDGE_CURVE ( 'NONE', #5339, #17343, #2841, .T. ) ;
#25436=CARTESIAN_POINT ( 'NONE',  ( 3.496762477039628614, -0.4822370993093180735, -0.6999999999999784173 ) ) ;
#25447=CARTESIAN_POINT ( 'NONE',  ( -23.87963657974984955, -15.55698410977798929, 4.493007575000013354 ) ) ;
#25450=CARTESIAN_POINT ( 'NONE',  ( -22.97593508925929129, 15.65128309461163703, 8.000000000000007105 ) ) ;
#25454=CARTESIAN_POINT ( 'NONE',  ( -28.49528339128749366, -0.5184828350247786544, 8.000000000000007105 ) ) ;
#25455=CARTESIAN_POINT ( 'NONE',  ( 24.18069373756728524, 13.78367726165553009, 8.000000000000007105 ) ) ;
#25464=EDGE_CURVE ( 'NONE', #28983, #10752, #26693, .T. ) ;
#25483=B_SPLINE_CURVE_WITH_KNOTS ( 'NONE', 3,
 ( #11837, #1619, #27890, #18753, #11370, #6334 ),
 .UNSPECIFIED., .F., .F.,
 ( 4, 2, 4 ),
 ( 0.000000000000000000, 0.5000000000000000000, 1.000000000000000000 ),
 .UNSPECIFIED. ) ;
#25484=CARTESIAN_POINT ( 'NONE',  ( -16.06988921239048551, -8.208160914692745891, -0.6999999999999784173 ) ) ;
#25495=CARTESIAN_POINT ( 'NONE',  ( -20.30403093158959038, 20.00000000003189626, 0.8742661550000252468 ) ) ;
#25497=CARTESIAN_POINT ( 'NONE',  ( 25.33584480268451600, 14.29478671887457608, 0.7595836940000044724 ) ) ;
#25510=B_SPLINE_CURVE_WITH_KNOTS ( 'NONE', 3,
 ( #12406, #14626, #24215, #2657, #10057, #14473 ),
 .UNSPECIFIED., .F., .F.,
 ( 4, 2, 4 ),
 ( 0.000000000000000000, 0.5000000000000000000, 1.000000000000000000 ),
 .UNSPECIFIED. ) ;
#25521=CARTESIAN_POINT ( 'NONE',  ( 0.4831567132674381426, -28.49614615030699838, 3.899998581000013509 ) ) ;
#25526=ADVANCED_FACE ( 'NONE', ( #9316 ), #16553, .F. ) ;
#25538=CARTESIAN_POINT ( 'NONE',  ( 16.06675444876397307, -9.020011618195203695, -0.6999999999999784173 ) ) ;
#25574=CARTESIAN_POINT ( 'NONE',  ( 24.32472724076343695, -13.45989056521276872, 3.899998581000013509 ) ) ;
#25575=CARTESIAN_POINT ( 'NONE',  ( 26.15365760668691308, 9.467937797150383972, 0.08279779700001710374 ) ) ;
#25585=EDGE_CURVE ( 'NONE', #16332, #13797, #15595, .T. ) ;
#25586=B_SPLINE_CURVE_WITH_KNOTS ( 'NONE', 1,
 ( #30940, #24016 ),
 .UNSPECIFIED., .F., .F.,
 ( 2, 2 ),
 ( -0.6999999999459999289, 1.998401444325281773E-15 ),
 .UNSPECIFIED. ) ;
#25589=CARTESIAN_POINT ( 'NONE',  ( 26.79556473285982321, 0.4875557887249851730, -0.6999999999999784173 ) ) ;
#25590=CARTESIAN_POINT ( 'NONE',  ( -24.32472894358752313, 13.45989150749028873, 6.099998581000020792 ) ) ;
#25600=CARTESIAN_POINT ( 'NONE',  ( -24.24144457387483698, -14.48500828217274439, 0.000000000000000000 ) ) ;
#25621=CARTESIAN_POINT ( 'NONE',  ( 23.24837000782807905, 15.24326850565740443, 4.713240265032504261 ) ) ;
#25627=CARTESIAN_POINT ( 'NONE',  ( 27.71261514784112379, 0.5042418800004117019, 0.5514269430000329208 ) ) ;
#25628=CARTESIAN_POINT ( 'NONE',  ( -17.93324555120827668, 10.97998838178171432, -0.6999999999999784173 ) ) ;
#25643=CARTESIAN_POINT ( 'NONE',  ( 20.30396079652883756, 20.00000000004620304, 1.000000000000000888 ) ) ;
#25648=CARTESIAN_POINT ( 'NONE',  ( -16.70947337985631975, 12.10243747010558657, -4.336808689942017736E-16 ) ) ;
#25657=CARTESIAN_POINT ( 'NONE',  ( -18.15338440918069907, 19.92139857694655802, 0.007026247000024854472 ) ) ;
#25658=CARTESIAN_POINT ( 'NONE',  ( -23.17877535335809824, -15.80276672810151517, 8.000000000000007105 ) ) ;
#25660=CARTESIAN_POINT ( 'NONE',  ( 28.49528339128749366, 0.5184828350247432383, 0.7595836940000044724 ) ) ;
#25673=ORIENTED_EDGE ( 'NONE', *, *, #17557, .F. ) ;
#25678=CARTESIAN_POINT ( 'NONE',  ( 24.36375418468539067, 14.78716628296302282, 3.904032100999987875 ) ) ;
#25682=CARTESIAN_POINT ( 'NONE',  ( -0.4969045691571343237, -28.49594262166996828, 4.493528488000025689 ) ) ;
#25696=CARTESIAN_POINT ( 'NONE',  ( -17.93324555120827668, 10.97998838178171432, -1.000005633855494125E-09 ) ) ;
#25697=CARTESIAN_POINT ( 'NONE',  ( 1.157672466183025994, -27.77645868488734138, 5.900907654000003610 ) ) ;
#25710=EDGE_LOOP ( 'NONE', ( #2141, #15280, #27146, #10618 ) ) ;
#25712=ORIENTED_EDGE ( 'NONE', *, *, #17077, .T. ) ;
#25714=VERTEX_POINT ( 'NONE', #11025 ) ;
#25717=CARTESIAN_POINT ( 'NONE',  ( 24.70074545475921823, -14.21822122957610368, 6.002806299999996043 ) ) ;
#25724=ORIENTED_EDGE ( 'NONE', *, *, #14355, .F. ) ;
#25728=ORIENTED_EDGE ( 'NONE', *, *, #11241, .T. ) ;
#25733=CARTESIAN_POINT ( 'NONE',  ( 25.85884820509708604, 9.361201669947201154, 0.000000000000000000 ) ) ;
#25746=CARTESIAN_POINT ( 'NONE',  ( -0.01646793526671820954, -3.529820002194270945, -0.6999999999999783062 ) ) ;
#25753=CARTESIAN_POINT ( 'NONE',  ( -26.58668732968209980, 4.592113237615420118, 0.000000000000000000 ) ) ;
#25759=CARTESIAN_POINT ( 'NONE',  ( -15.73094807277625584, 10.87373459869253445, -0.6999999999999784173 ) ) ;
#25760=B_SPLINE_SURFACE_WITH_KNOTS ( 'NONE', 5, 1, ( 
 ( #12236, #16806 ),
 ( #19635, #19484 ),
 ( #2346, #24057 ),
 ( #5004, #2190 ),
 ( #16801, #29071 ),
 ( #28616, #11780 ) ),
 .UNSPECIFIED., .F., .F., .F.,
 ( 6, 6 ),
 ( 2, 2 ),
 ( 4.999999893150000041, 7.000000000150000012 ),
 ( -1.998401444329999950E-15, 0.6999999999459999289 ),
 .UNSPECIFIED. ) ;
#25762=CARTESIAN_POINT ( 'NONE',  ( -0.1501630637024684578, -28.50011693320769623, 4.099092748999999536 ) ) ;
#25778=CARTESIAN_POINT ( 'NONE',  ( -16.04158851053540857, -9.763538383445707680, -0.6999999989999727834 ) ) ;
#25789=EDGE_LOOP ( 'NONE', ( #23590, #27353, #17622, #8489 ) ) ;
#25800=CARTESIAN_POINT ( 'NONE',  ( -16.56504334151864910, 12.07643063650710857, -4.336808689942017243E-16 ) ) ;
#25809=CARTESIAN_POINT ( 'NONE',  ( 24.10046253615778511, 13.85738024105139488, 4.039349569685102281 ) ) ;
#25810=CARTESIAN_POINT ( 'NONE',  ( -19.49296039895628851, 19.58649212980878929, 0.4407160300000101394 ) ) ;
#25811=CARTESIAN_POINT ( 'NONE',  ( 1.461759203915476313, -27.91510208544341509, 8.000000000000007105 ) ) ;
#25813=CARTESIAN_POINT ( 'NONE',  ( 27.03594125075309762, 0.4919295335570642025, -0.6999999999999784173 ) ) ;
#25816=EDGE_CURVE ( 'NONE', #6569, #2099, #6244, .T. ) ;
#25836=CARTESIAN_POINT ( 'NONE',  ( 17.43495665832235630, -7.923569363432783952, -4.336808689942017243E-16 ) ) ;
#25849=FACE_OUTER_BOUND ( 'NONE', #17560, .T. ) ;
#25852=CARTESIAN_POINT ( 'NONE',  ( 0.5746121234326042604, -27.79431838510023312, 6.098651075000017130 ) ) ;
#25860=CARTESIAN_POINT ( 'NONE',  ( 0.7646642646963620615, -28.49022165133369455, 3.920206710000012862 ) ) ;
#25862=ORIENTED_EDGE ( 'NONE', *, *, #11896, .T. ) ;
#25869=VERTEX_POINT ( 'NONE', #16203 ) ;
#25872=B_SPLINE_CURVE_WITH_KNOTS ( 'NONE', 1,
 ( #24009, #10453 ),
 .UNSPECIFIED., .F., .F.,
 ( 2, 2 ),
 ( -2.557518061549999935E-06, 0.7000000000009999335 ),
 .UNSPECIFIED. ) ;
#25878=CARTESIAN_POINT ( 'NONE',  ( -18.17095077428239236, 20.37181511265805156, -0.6577119969999878357 ) ) ;
#25885=VECTOR ( 'NONE', #24339, 1000.000000000000000 ) ;
#25896=CARTESIAN_POINT ( 'NONE',  ( 16.06409288198120677, 11.12626540299224942, -0.6999999999999784173 ) ) ;
#25904=CARTESIAN_POINT ( 'NONE',  ( 17.16657240421717390, -9.000000000001264766, -0.6999999999999784173 ) ) ;
#25911=CARTESIAN_POINT ( 'NONE',  ( -27.24406355354269849, -0.4957164003159642007, 0.08279779300002232389 ) ) ;
#25912=VERTEX_POINT ( 'NONE', #21404 ) ;
#25914=CARTESIAN_POINT ( 'NONE',  ( -23.23277126416379801, -15.26692729116844482, 4.895813258999987205 ) ) ;
#25917=FACE_OUTER_BOUND ( 'NONE', #1946, .T. ) ;
#25920=CARTESIAN_POINT ( 'NONE',  ( -23.81866442513004856, -14.33570206453694240, 6.099998581000020792 ) ) ;
#25929=CARTESIAN_POINT ( 'NONE',  ( -4.499842235593497719, -29.81936866046843093, 0.000000000000000000 ) ) ;
#25933=CYLINDRICAL_SURFACE ( 'NONE', #3242, 1.099999999999999867 ) ;
#25936=ORIENTED_EDGE ( 'NONE', *, *, #21955, .T. ) ;
#25950=FACE_BOUND ( 'NONE', #1334, .T. ) ;
#25960=CARTESIAN_POINT ( 'NONE',  ( 24.26024164798999649, 13.57543367310533000, 4.323353004038539282 ) ) ;
#25962=CARTESIAN_POINT ( 'NONE',  ( -28.43007859798022707, -2.264358681363081605, 8.000000000000007105 ) ) ;
#25964=CARTESIAN_POINT ( 'NONE',  ( 26.45504170235313879, 9.577025040725851923, -0.5592437529999827461 ) ) ;
#25987=CARTESIAN_POINT ( 'NONE',  ( 18.94011831790433931, 20.00034691316145086, -0.5314523398227246620 ) ) ;
#25990=DIRECTION ( 'NONE',  ( 0.000000000000000000, 0.000000000000000000, -1.000000000000000000 ) ) ;
#25996=FACE_BOUND ( 'NONE', #5072, .T. ) ;
#26001=VECTOR ( 'NONE', #10422, 1000.000000000000000 ) ;
#26005=ORIENTED_EDGE ( 'NONE', *, *, #10616, .T. ) ;
#26007=CARTESIAN_POINT ( 'NONE',  ( -24.88589369081283920, 13.89120818323882922, 6.095967889000020179 ) ) ;
#26039=CARTESIAN_POINT ( 'NONE',  ( 1.186786632755666426, -28.47586096821117252, 4.099089508000003157 ) ) ;
#26040=CARTESIAN_POINT ( 'NONE',  ( -23.81866442513186755, -14.33570206443695838, 3.899998581000013509 ) ) ;
#26058=CARTESIAN_POINT ( 'NONE',  ( 1.379247882464924579, -27.76613141686495823, 4.319830470999985295 ) ) ;
#26062=CARTESIAN_POINT ( 'NONE',  ( -27.58051882800086574, -7.764119750527245678, 0.5514269430000329208 ) ) ;
#26068=CARTESIAN_POINT ( 'NONE',  ( 17.14656078602323319, -7.900182044548062166, -0.6999999989999727834 ) ) ;
#26082=CARTESIAN_POINT ( 'NONE',  ( -24.70448872506469229, 12.74983733322420321, 4.239730451999990102 ) ) ;
#26087=CARTESIAN_POINT ( 'NONE',  ( 17.43374459427612067, -7.923010675184074536, -0.6999999999999784173 ) ) ;
#26102=CARTESIAN_POINT ( 'NONE',  ( -25.38146355610767912, 12.59839636679889807, 3.799999999999998046 ) ) ;
#26105=CARTESIAN_POINT ( 'NONE',  ( -27.79539923781770128, -0.5057481688779147389, 8.000000000000007105 ) ) ;
#26109=ORIENTED_EDGE ( 'NONE', *, *, #5724, .T. ) ;
#26112=CARTESIAN_POINT ( 'NONE',  ( 25.43650006538670638, 11.58982781969230125, 8.000000000000007105 ) ) ;
#26115=CARTESIAN_POINT ( 'NONE',  ( 24.35342033856957045, 13.40728427522152444, 4.712140172059656962 ) ) ;
#26116=CARTESIAN_POINT ( 'NONE',  ( -17.83930458849792089, 19.99999999999597478, -1.000005633855494125E-09 ) ) ;
#26117=CARTESIAN_POINT ( 'NONE',  ( -15.73547908372051296, -8.877245731167342058, 0.000000000000000000 ) ) ;
#26118=CARTESIAN_POINT ( 'NONE',  ( -19.49296039895628851, 19.58649212980878929, 0.4407160300000101394 ) ) ;
#26119=B_SPLINE_CURVE_WITH_KNOTS ( 'NONE', 3,
 ( #2735, #29006, #7752, #17355, #14858, #7452, #24287, #10129, #24449, #26347 ),
 .UNSPECIFIED., .F., .F.,
 ( 4, 2, 2, 2, 4 ),
 ( 0.000000000000000000, 0.2500000000000000000, 0.5000000000000000000, 0.7500000000000000000, 1.000000000000000000 ),
 .UNSPECIFIED. ) ;
#26124=ADVANCED_FACE ( 'NONE', ( #24075 ), #19656, .F. ) ;
#26131=ORIENTED_EDGE ( 'NONE', *, *, #23494, .T. ) ;
#26134=B_SPLINE_CURVE_WITH_KNOTS ( 'NONE', 1,
 ( #9093, #25643 ),
 .UNSPECIFIED., .F., .F.,
 ( 2, 2 ),
 ( -0.7000000000189999794, 2.331468351712828735E-15 ),
 .UNSPECIFIED. ) ;
#26140=CARTESIAN_POINT ( 'NONE',  ( 23.76534794177020871, 14.42397062701149935, 3.904032100999987875 ) ) ;
#26143=CARTESIAN_POINT ( 'NONE',  ( 18.31933453193921579, 19.99999486414201755, -0.6702687248541838727 ) ) ;
#26151=DIRECTION ( 'NONE',  ( -0.000000000000000000, 0.000000000000000000, -1.000000000000000000 ) ) ;
#26152=CARTESIAN_POINT ( 'NONE',  ( 24.98081130624543889, 13.71897605842228529, 5.104178997000024864 ) ) ;
#26156=CARTESIAN_POINT ( 'NONE',  ( 0.6090474298383116158, -27.79358669172298946, 6.095948809000023338 ) ) ;
#26158=VERTEX_POINT ( 'NONE', #15390 ) ;
#26165=CARTESIAN_POINT ( 'NONE',  ( 23.98258507289250474, 15.39789216307533160, 4.239862992999999136 ) ) ;
#26168=EDGE_CURVE ( 'NONE', #20235, #25231, #28702, .T. ) ;
#26180=ORIENTED_EDGE ( 'NONE', *, *, #12872, .T. ) ;
#26182=EDGE_CURVE ( 'NONE', #24853, #18124, #23083, .T. ) ;
#26192=EDGE_CURVE ( 'NONE', #18763, #30472, #20446, .T. ) ;
#26212=CARTESIAN_POINT ( 'NONE',  ( -26.79556473285982321, -0.4875557887250224209, 0.000000000000000000 ) ) ;
#26216=CARTESIAN_POINT ( 'NONE',  ( -24.36375418918093061, -14.78716628874576244, 3.904032100999987875 ) ) ;
#26225=CARTESIAN_POINT ( 'NONE',  ( -15.73293181562159404, -9.017240966205054775, 0.000000000000000000 ) ) ;
#26235=CARTESIAN_POINT ( 'NONE',  ( -16.77890539070889275, -7.900403655799213887, 0.000000000000000000 ) ) ;
#26236=CARTESIAN_POINT ( 'NONE',  ( 24.96253706050071131, 13.75225324050492581, 5.310538874999992665 ) ) ;
#26240=EDGE_CURVE ( 'NONE', #28488, #25231, #20903, .T. ) ;
#26255=CARTESIAN_POINT ( 'NONE',  ( -27.52676963214412353, -0.5008603480660359653, 0.2686740700000300741 ) ) ;
#26267=CARTESIAN_POINT ( 'NONE',  ( -15.93069263124182555, -8.365606382343615977, 0.000000000000000000 ) ) ;
#26271=CARTESIAN_POINT ( 'NONE',  ( -24.47278419579111386, -14.60601539740217092, 6.095965388000001539 ) ) ;
#26278=ORIENTED_EDGE ( 'NONE', *, *, #3349, .T. ) ;
#26282=ORIENTED_EDGE ( 'NONE', *, *, #12379, .T. ) ;
#26284=ORIENTED_EDGE ( 'NONE', *, *, #9259, .F. ) ;
#26292=CARTESIAN_POINT ( 'NONE',  ( 18.62215279828695458, 19.99998923236033832, -0.6161023301325340151 ) ) ;
#26293=CARTESIAN_POINT ( 'NONE',  ( -24.09407738750993033, 13.86899051154378881, 6.002806299999996043 ) ) ;
#26309=B_SPLINE_CURVE_WITH_KNOTS ( 'NONE', 5,
 ( #65, #14382, #14688, #23980, #12008, #21615, #19246, #24276, #28833, #7290, #16879, #834, #22544, #5845, #24901 ),
 .UNSPECIFIED., .F., .F.,
 ( 6, 3, 3, 3, 6 ),
 ( 0.000000000000000000, 0.2999999999989615973, 0.5999999999979230836, 0.7999999999996538769, 1.000000000000000000 ),
 .UNSPECIFIED. ) ;
#26312=CARTESIAN_POINT ( 'NONE',  ( 24.41841038956698640, 14.69667349781389376, 6.099998581000020792 ) ) ;
#26318=ORIENTED_EDGE ( 'NONE', *, *, #5246, .T. ) ;
#26320=CARTESIAN_POINT ( 'NONE',  ( 23.81776757409229361, 15.65134803726813217, 4.895813257000003915 ) ) ;
#26323=ORIENTED_EDGE ( 'NONE', *, *, #17090, .F. ) ;
#26339=CARTESIAN_POINT ( 'NONE',  ( -19.44855986669129777, 20.00001404973996699, -0.2987059375404466643 ) ) ;
#26340=B_SPLINE_SURFACE_WITH_KNOTS ( 'NONE', 5, 1, ( 
 ( #19874, #3480 ),
 ( #26788, #22229 ),
 ( #26950, #29455 ),
 ( #8045, #10117 ),
 ( #987, #17345 ),
 ( #14993, #12932 ),
 ( #3173, #10721 ),
 ( #24437, #27253 ),
 ( #2872, #7741 ) ),
 .UNSPECIFIED., .F., .F., .F.,
 ( 6, 3, 6 ),
 ( 2, 2 ),
 ( 0.000000000000000000, 55.31395511720000258, 94.75474465359999954 ),
 ( -3.500000000000000000, 3.500000000000000000 ),
 .UNSPECIFIED. ) ;
#26346=CARTESIAN_POINT ( 'NONE',  ( 0.7459188900473354700, -27.79046661982714639, 3.920206710000012862 ) ) ;
#26347=CARTESIAN_POINT ( 'NONE',  ( -24.83827471527357744, 12.48687850854618198, 4.999998581000003384 ) ) ;
#26357=AXIS2_PLACEMENT_3D ( 'NONE', #5672, #17774, #27232 ) ;
#26367=CARTESIAN_POINT ( 'NONE',  ( 24.41841038956698640, 14.69667349781389376, 6.099998581000020792 ) ) ;
#26385=CARTESIAN_POINT ( 'NONE',  ( 22.36170820408901960, 17.71391973664089292, 6.000000000000005329 ) ) ;
#26387=FACE_OUTER_BOUND ( 'NONE', #3365, .T. ) ;
#26392=CARTESIAN_POINT ( 'NONE',  ( -24.44014312407112399, 13.24968496200000523, 3.920132093000017193 ) ) ;
#26410=CARTESIAN_POINT ( 'NONE',  ( -23.83006840756495137, 14.31758445875128594, 4.492876031000014869 ) ) ;
#26413=CARTESIAN_POINT ( 'NONE',  ( 14.25032083441342934, -27.35421241409322946, 8.000000000000007105 ) ) ;
#26420=EDGE_CURVE ( 'NONE', #7280, #4633, #7307, .T. ) ;
#26424=CARTESIAN_POINT ( 'NONE',  ( -3.040504021322313122, -1.733590290792417887, 0.000000000000000000 ) ) ;
#26426=CARTESIAN_POINT ( 'NONE',  ( 25.46368747440213198, -12.80129684534102807, 4.999998581000003384 ) ) ;
#26427=CARTESIAN_POINT ( 'NONE',  ( -15.74934601578848614, -8.774721957951193474, 0.000000000000000000 ) ) ;
#26431=CARTESIAN_POINT ( 'NONE',  ( -24.32472894358752313, 13.45989150749028873, 6.099998581000020792 ) ) ;
#26445=CARTESIAN_POINT ( 'NONE',  ( 17.43374459646987873, 12.07698932438915840, -0.6999999999999784173 ) ) ;
#26447=CARTESIAN_POINT ( 'NONE',  ( 22.62517538432032183, 16.36045799713948057, 8.000000000000007105 ) ) ;
#26449=CARTESIAN_POINT ( 'NONE',  ( 18.22359483181848105, 19.99999695154517809, -0.6804351800466643674 ) ) ;
#26450=CARTESIAN_POINT ( 'NONE',  ( -17.62526668104891314, 11.76353838341477953, -0.6999999999999784173 ) ) ;
#26457=CARTESIAN_POINT ( 'NONE',  ( -0.7509949761406778945, -3.448174246630094864, 0.000000000000000000 ) ) ;
#26460=CARTESIAN_POINT ( 'NONE',  ( 19.29866511436280874, 19.63492491799039996, 0.3046098590000212436 ) ) ;
#26464=CARTESIAN_POINT ( 'NONE',  ( -24.86822223968379575, -13.92223202017373573, 4.319317663000004970 ) ) ;
#26479=CARTESIAN_POINT ( 'NONE',  ( 16.50668551558484509, 10.10821397331193339, -0.6999999999999784173 ) ) ;
#26480=ADVANCED_FACE ( 'NONE', ( #19619 ), #12193, .F. ) ;
#26487=CARTESIAN_POINT ( 'NONE',  ( -18.42955812989342945, 20.00001476357908814, -0.6532716553696857886 ) ) ;
#26519=B_SPLINE_CURVE_WITH_KNOTS ( 'NONE', 5,
 ( #10190, #19791, #11280, #18023, #15845, #30154 ),
 .UNSPECIFIED., .F., .F.,
 ( 6, 6 ),
 ( 0.000000000000000000, 18.58426834389999982 ),
 .UNSPECIFIED. ) ;
#26522=CARTESIAN_POINT ( 'NONE',  ( -23.76534794678204321, -14.42397063190348483, 3.904032100999987875 ) ) ;
#26524=CARTESIAN_POINT ( 'NONE',  ( -22.90527192528401201, 16.36193184990112570, 1.000000000000000888 ) ) ;
#26529=CARTESIAN_POINT ( 'NONE',  ( 20.50699588867001211, 18.79637368904402095, 4.000000000000003553 ) ) ;
#26532=CARTESIAN_POINT ( 'NONE',  ( -23.98258507372315051, -15.39789217239198571, 5.760134161999996394 ) ) ;
#26544=DIRECTION ( 'NONE',  ( 0.7198537139083028835, -0.6941258031311204890, 0.000000000000000000 ) ) ;
#26566=ORIENTED_EDGE ( 'NONE', *, *, #14593, .T. ) ;
#26576=CARTESIAN_POINT ( 'NONE',  ( -19.06860189597471944, 19.69237645765742073, 0.2003674019999956979 ) ) ;
#26582=CARTESIAN_POINT ( 'NONE',  ( -24.60726957497166367, 14.37955347300500364, 5.901399683999997592 ) ) ;
#26584=VERTEX_POINT ( 'NONE', #5753 ) ;
#26600=CARTESIAN_POINT ( 'NONE',  ( 27.07818553041514065, 6.807801137122736712, 8.000000000000007105 ) ) ;
#26603=CARTESIAN_POINT ( 'NONE',  ( 17.92796488783011455, 19.99992859427167957, -0.6995494494441671929 ) ) ;
#26604=CARTESIAN_POINT ( 'NONE',  ( -23.83006840756313238, 14.31758445865130369, 5.507121130000014020 ) ) ;
#26605=CYLINDRICAL_SURFACE ( 'NONE', #5063, 1.099999999999999867 ) ;
#26610=CARTESIAN_POINT ( 'NONE',  ( 24.37165445055180157, -14.77472140295711434, 4.999998581000003384 ) ) ;
#26622=B_SPLINE_SURFACE_WITH_KNOTS ( 'NONE', 5, 1, ( 
 ( #30879, #16236 ),
 ( #1931, #9149 ),
 ( #28196, #16085 ),
 ( #4590, #21126 ),
 ( #13724, #21275 ),
 ( #11676, #19069 ),
 ( #14046, #6955 ),
 ( #14363, #25697 ),
 ( #4128, #30418 ),
 ( #8837, #1779 ),
 ( #4444, #23650 ),
 ( #16548, #26156 ),
 ( #18752, #25852 ),
 ( #2086, #9310 ),
 ( #18599, #11369 ) ),
 .UNSPECIFIED., .F., .F., .F.,
 ( 6, 3, 3, 3, 6 ),
 ( 2, 2 ),
 ( 0.000000000000000000, 0.5239015560140000138, 1.047803112029999983, 1.571704668039999975, 1.746338520049999898 ),
 ( -0.7000000000009999335, 2.556813327499999719E-06 ),
 .UNSPECIFIED. ) ;
#26624=CARTESIAN_POINT ( 'NONE',  ( -16.66884554159437926, 9.902812559993083852, -0.6999999999999783062 ) ) ;
#26636=ORIENTED_EDGE ( 'NONE', *, *, #8459, .F. ) ;
#26637=FACE_OUTER_BOUND ( 'NONE', #18754, .T. ) ;
#26642=FACE_OUTER_BOUND ( 'NONE', #25789, .T. ) ;
#26657=CARTESIAN_POINT ( 'NONE',  ( 16.40303402075260308, 10.20816091466531716, 0.000000000000000000 ) ) ;
#26663=CARTESIAN_POINT ( 'NONE',  ( -17.93324555128263142, -9.020011618190519442, -0.6999999989999727834 ) ) ;
#26679=EDGE_CURVE ( 'NONE', #23153, #18290, #6570, .T. ) ;
#26681=CARTESIAN_POINT ( 'NONE',  ( -24.06750537087731701, -15.26514226597108781, 5.901296963999991263 ) ) ;
#26686=CARTESIAN_POINT ( 'NONE',  ( -19.71199437610940919, -20.57358076904808897, -0.6999999999999784173 ) ) ;
#26688=CARTESIAN_POINT ( 'NONE',  ( 14.60916111670818474, -28.04296597385482315, 8.000000000000007105 ) ) ;
#26691=B_SPLINE_CURVE_WITH_KNOTS ( 'NONE', 5,
 ( #14179, #18732, #16377, #28179, #1761, #1910, #11505, #13709, #16680, #14028, #16531, #4110, #23314, #28333, #11659 ),
 .UNSPECIFIED., .F., .F.,
 ( 6, 3, 3, 3, 6 ),
 ( 0.000000000000000000, 0.1000000000011452422, 0.3999999999988547161, 0.7000000000005726086, 1.000000000000000000 ),
 .UNSPECIFIED. ) ;
#26693=LINE ( 'NONE', #5130, #25885 ) ;
#26699=ORIENTED_EDGE ( 'NONE', *, *, #20250, .T. ) ;
#26707=CARTESIAN_POINT ( 'NONE',  ( -24.43008698341936835, 14.67811372381255630, 4.492876031000014869 ) ) ;
#26708=CARTESIAN_POINT ( 'NONE',  ( -27.87609112763809449, 3.928995115440388375, 6.600000000000022737 ) ) ;
#26717=CARTESIAN_POINT ( 'NONE',  ( -24.47278419579111386, -14.60601539740217092, 3.904031772999999816 ) ) ;
#26719=CARTESIAN_POINT ( 'NONE',  ( 22.97559295454826511, 15.65128684788800939, 8.000000000000007105 ) ) ;
#26723=CARTESIAN_POINT ( 'NONE',  ( -19.80535357387461204, 19.50875577042408793, 0.9260390330000090042 ) ) ;
#26728=CARTESIAN_POINT ( 'NONE',  ( -24.52721838146529620, 14.51532614515499020, 5.760265123000013254 ) ) ;
#26735=CARTESIAN_POINT ( 'NONE',  ( 24.50348397774211051, -13.13223627713423092, 3.957489296000010981 ) ) ;
#26737=VERTEX_POINT ( 'NONE', #15660 ) ;
#26740=B_SPLINE_CURVE_WITH_KNOTS ( 'NONE', 5,
 ( #11778, #30672, #16645, #18698, #26255, #10683, #29878, #27668, #22802 ),
 .UNSPECIFIED., .F., .F.,
 ( 6, 3, 6 ),
 ( 8.011061266649999624, 8.831591450809998634, 9.652121634960000307 ),
 .UNSPECIFIED. ) ;
#26748=FACE_OUTER_BOUND ( 'NONE', #22869, .T. ) ;
#26752=CARTESIAN_POINT ( 'NONE',  ( -23.77307140041805411, 14.41181874028064591, 5.104215870000011535 ) ) ;
#26754=VECTOR ( 'NONE', #17315, 1000.000000000000000 ) ;
#26760=ADVANCED_FACE ( 'NONE', ( #16288 ), #8733, .F. ) ;
#26761=LINE ( 'NONE', #9776, #26754 ) ;
#26762=CARTESIAN_POINT ( 'NONE',  ( 24.86822223037987456, 13.92223202030449691, 5.680679506000013923 ) ) ;
#26767=CARTESIAN_POINT ( 'NONE',  ( -24.75645986059852177, -14.12045945554185522, 4.098702617000016701 ) ) ;
#26769=EDGE_CURVE ( 'NONE', #4259, #10529, #23809, .T. ) ;
#26779=B_SPLINE_SURFACE_WITH_KNOTS ( 'NONE', 5, 1, ( 
 ( #29357, #10174 ),
 ( #12844, #29820 ),
 ( #12677, #29515 ),
 ( #8408, #7802 ),
 ( #15356, #17399 ),
 ( #27005, #19775 ),
 ( #24954, #19927 ),
 ( #20082, #5443 ),
 ( #13139, #17694 ),
 ( #27312, #10789 ),
 ( #7950, #3386 ),
 ( #5751, #12990 ),
 ( #22287, #15053 ),
 ( #8257, #15196 ),
 ( #24647, #22602 ) ),
 .UNSPECIFIED., .F., .F., .F.,
 ( 6, 3, 3, 3, 6 ),
 ( 2, 2 ),
 ( 0.000000000000000000, 0.5239017170190000128, 1.047803434039999981, 1.571705151059999972, 1.746339056730000117 ),
 ( -0.7000000000009999335, 2.556331278550000249E-06 ),
 .UNSPECIFIED. ) ;
#26780=ORIENTED_EDGE ( 'NONE', *, *, #26192, .T. ) ;
#26782=ORIENTED_EDGE ( 'NONE', *, *, #13819, .F. ) ;
#26787=CARTESIAN_POINT ( 'NONE',  ( -24.83272648880584654, 12.49791454310039640, 5.208434320000010942 ) ) ;
#26788=CARTESIAN_POINT ( 'NONE',  ( -28.68577476999353237, 9.950727454195712696, 1.000000000000000888 ) ) ;
#26800=CARTESIAN_POINT ( 'NONE',  ( 0.5184513693225187847, -28.49550581263314086, 3.899998581000013509 ) ) ;
#26811=CARTESIAN_POINT ( 'NONE',  ( -26.40151772468378510, 8.923123374263472130, 0.08279779700001710374 ) ) ;
#26838=CARTESIAN_POINT ( 'NONE',  ( -23.96357375497718678, -14.09276578719063266, 3.927141029190090560 ) ) ;
#26842=CARTESIAN_POINT ( 'NONE',  ( 23.94939220324485518, -20.40613828787117967, 0.2374258030000131470 ) ) ;
#26847=B_SPLINE_CURVE_WITH_KNOTS ( 'NONE', 5,
 ( #22459, #909, #17567, #15518, #15212, #27174, #12692, #13154, #29688, #10647, #30153, #22927, #22761, #6238, #8114 ),
 .UNSPECIFIED., .F., .F.,
 ( 6, 3, 3, 3, 6 ),
 ( 0.000000000000000000, 0.1000000000000000472, 0.3999999999942737139, 0.6999999999994274136, 1.000000000000000000 ),
 .UNSPECIFIED. ) ;
#26853=CARTESIAN_POINT ( 'NONE',  ( 19.80526555972147307, 19.50877392102524155, 2.600000000000019185 ) ) ;
#26866=VERTEX_POINT ( 'NONE', #2592 ) ;
#26868=CARTESIAN_POINT ( 'NONE',  ( -24.09407738750993033, 13.86899051154378881, 3.997190861000005313 ) ) ;
#26878=CARTESIAN_POINT ( 'NONE',  ( 24.97472003062369694, 13.73006752330286595, 4.791638082000004850 ) ) ;
#26901=ORIENTED_EDGE ( 'NONE', *, *, #9395, .T. ) ;
#26910=CARTESIAN_POINT ( 'NONE',  ( 23.80322556508107112, 14.59355840047072661, 8.000000000000007105 ) ) ;
#26913=CARTESIAN_POINT ( 'NONE',  ( -23.79228473957821777, 14.38012949749760416, 5.310643621000004977 ) ) ;
#26920=PRODUCT_DEFINITION_FORMATION_WITH_SPECIFIED_SOURCE ( 'ANY', '', #25418, .NOT_KNOWN. ) ;
#26921=CARTESIAN_POINT ( 'NONE',  ( 24.14205449336675713, -13.78537897189897343, 6.042507811999997536 ) ) ;
#26923=CARTESIAN_POINT ( 'NONE',  ( 19.80526555982327608, 19.50877392092707296, 0.9260799790000162623 ) ) ;
#26930=CARTESIAN_POINT ( 'NONE',  ( -24.98081131316241255, -13.71897606304888662, 4.999998581000003384 ) ) ;
#26950=CARTESIAN_POINT ( 'NONE',  ( -24.06826084723317649, 20.50742046750733039, 1.000000000000000888 ) ) ;
#26955=CARTESIAN_POINT ( 'NONE',  ( -17.91041691994261242, -8.732827808381141921, -0.6999999999999784173 ) ) ;
#26965=ORIENTED_EDGE ( 'NONE', *, *, #19134, .F. ) ;
#26968=B_SPLINE_CURVE_WITH_KNOTS ( 'NONE', 3,
 ( #22383, #15441, #3321, #17936, #980, #27094 ),
 .UNSPECIFIED., .F., .F.,
 ( 4, 2, 4 ),
 ( 0.000000000000000000, 0.5000000000000000000, 1.000000000000000000 ),
 .UNSPECIFIED. ) ;
#26969=CARTESIAN_POINT ( 'NONE',  ( -26.85558069653561120, 9.076679569434611849, 0.5514269540000116265 ) ) ;
#26976=CARTESIAN_POINT ( 'NONE',  ( 23.47637528925218575, 14.89020703997133488, 5.901296968999991677 ) ) ;
#26981=CARTESIAN_POINT ( 'NONE',  ( -21.46610162199371885, 17.08729007858795157, -0.6999999999999784173 ) ) ;
#26988=CARTESIAN_POINT ( 'NONE',  ( 24.70074545465923421, -14.21822122957792445, 3.997190862000010725 ) ) ;
#26993=CARTESIAN_POINT ( 'NONE',  ( -23.87963657974803056, -15.55698410987797331, 5.506989586000016423 ) ) ;
#26998=CARTESIAN_POINT ( 'NONE',  ( -4.778179638654715511, -31.66384348256136150, 0.5017677510000262409 ) ) ;
#27001=CARTESIAN_POINT ( 'NONE',  ( 24.41841038956698640, 14.69667349781389376, 6.099998581000020792 ) ) ;
#27005=CARTESIAN_POINT ( 'NONE',  ( -0.3775595308337927891, -28.49777658967324356, 5.680150179000031940 ) ) ;
#27012=ORIENTED_EDGE ( 'NONE', *, *, #24678, .F. ) ;
#27013=VERTEX_POINT ( 'NONE', #18458 ) ;
#27015=CARTESIAN_POINT ( 'NONE',  ( 13.81022701813574116, -26.50938575128768804, 0.000000000000000000 ) ) ;
#27020=CARTESIAN_POINT ( 'NONE',  ( -24.32472894358752313, 13.45989150749028873, 3.899998581000013509 ) ) ;
#27030=CARTESIAN_POINT ( 'NONE',  ( -24.54452542612009225, -14.48555670042145138, 3.920144560000005107 ) ) ;
#27043=AXIS2_PLACEMENT_3D ( 'NONE', #15838, #3874, #22756 ) ;
#27044=CARTESIAN_POINT ( 'NONE',  ( -17.10181184920913822, -10.07643063668447958, -0.6999999999999785283 ) ) ;
#27057=CARTESIAN_POINT ( 'NONE',  ( 24.00926693399461342, 14.01467022386263395, 3.957524335000017768 ) ) ;
#27070=CARTESIAN_POINT ( 'NONE',  ( 24.60726958095619565, -14.37955347759689317, 5.901399682999991292 ) ) ;
#27074=CARTESIAN_POINT ( 'NONE',  ( 17.16657240421717390, -9.000000000001264766, -0.6999999999999784173 ) ) ;
#27090=EDGE_LOOP ( 'NONE', ( #18601, #21880, #20157, #12229 ) ) ;
#27094=CARTESIAN_POINT ( 'NONE',  ( -17.59696597919420213, 10.20816091468181774, -0.6999999999999784173 ) ) ;
#27100=CARTESIAN_POINT ( 'NONE',  ( -25.05552767696902450, 13.58331698520493269, 6.079865069000017996 ) ) ;
#27104=CARTESIAN_POINT ( 'NONE',  ( -19.80535357367646654, 19.50875577052770993, 2.200000064000007249 ) ) ;
#27109=CARTESIAN_POINT ( 'NONE',  ( 23.81866167241657806, 14.33570040768432996, 6.099998581000020792 ) ) ;
#27118=ORIENTED_EDGE ( 'NONE', *, *, #26168, .F. ) ;
#27123=CARTESIAN_POINT ( 'NONE',  ( -24.92917479049725316, 13.61031708633488613, 0.7069258409999890080 ) ) ;
#27131=LINE ( 'NONE', #862, #1915 ) ;
#27136=ADVANCED_FACE ( 'NONE', ( #164 ), #2760, .F. ) ;
#27138=CARTESIAN_POINT ( 'NONE',  ( 16.29899378188139281, 10.30852736161794958, 0.000000000000000000 ) ) ;
#27146=ORIENTED_EDGE ( 'NONE', *, *, #21380, .F. ) ;
#27155=CARTESIAN_POINT ( 'NONE',  ( -25.65182985565638418, -15.32775674290634704, 0.2374258030000131470 ) ) ;
#27170=CARTESIAN_POINT ( 'NONE',  ( 27.26968166180262898, -9.459502808761374837, 0.02487529600000981667 ) ) ;
#27174=CARTESIAN_POINT ( 'NONE',  ( 25.12046395012945155, -13.46291002088068289, 3.957489296000010981 ) ) ;
#27177=CARTESIAN_POINT ( 'NONE',  ( 24.70448873180906446, -12.74983733560190302, 5.760266709000011254 ) ) ;
#27185=CARTESIAN_POINT ( 'NONE',  ( -16.52606180369280864, 9.934045360728056551, -4.336808689942018722E-16 ) ) ;
#27210=CARTESIAN_POINT ( 'NONE',  ( 14.60916111670818474, -28.04296597385482315, 1.000000000000000888 ) ) ;
#27221=LINE ( 'NONE', #5664, #3116 ) ;
#27224=DIRECTION ( 'NONE',  ( 0.000000000000000000, 0.000000000000000000, -1.000000000000000000 ) ) ;
#27227=CARTESIAN_POINT ( 'NONE',  ( 0.5401834767575381946, -27.79499634052776358, 6.099998581000020792 ) ) ;
#27228=CARTESIAN_POINT ( 'NONE',  ( -16.81341597756113515, 9.900182044522454206, -1.000005633855494125E-09 ) ) ;
#27232=DIRECTION ( 'NONE',  ( -0.7198537139083028835, 0.6941258031311204890, 0.000000000000000000 ) ) ;
#27238=CARTESIAN_POINT ( 'NONE',  ( 24.93720649360215802, -13.79881813812812297, 6.099998581000020792 ) ) ;
#27239=EDGE_LOOP ( 'NONE', ( #15162, #16596, #26965, #9669 ) ) ;
#27250=CARTESIAN_POINT ( 'NONE',  ( -24.83273907627866706, 12.49792087830325471, 5.208434320000010942 ) ) ;
#27252=B_SPLINE_CURVE_WITH_KNOTS ( 'NONE', 3,
 ( #11140, #21204, #6092, #20577, #4058, #13654 ),
 .UNSPECIFIED., .F., .F.,
 ( 4, 2, 4 ),
 ( 0.000000000000000000, 0.5000000000000000000, 1.000000000000000000 ),
 .UNSPECIFIED. ) ;
#27253=CARTESIAN_POINT ( 'NONE',  ( 28.35945635836379708, 7.983396865348648674, 8.000000000000007105 ) ) ;
#27265=CARTESIAN_POINT ( 'NONE',  ( 1.366018022090341510, 3.254826447622997776, -0.6999999999999783062 ) ) ;
#27273=CARTESIAN_POINT ( 'NONE',  ( -21.85583880085616570, 17.39748151240578267, 0.2686751170000167832 ) ) ;
#27281=CARTESIAN_POINT ( 'NONE',  ( -24.39135169139981940, 14.74223402956394402, 4.689353541000001790 ) ) ;
#27282=DIRECTION ( 'NONE',  ( 0.000000000000000000, 0.000000000000000000, -1.000000000000000000 ) ) ;
#27285=CARTESIAN_POINT ( 'NONE',  ( -25.57973247309962872, 13.96556750262912416, 1.000000000000000888 ) ) ;
#27287=AXIS2_PLACEMENT_3D ( 'NONE', #27488, #5936, #15688 ) ;
#27291=ORIENTED_EDGE ( 'NONE', *, *, #25272, .T. ) ;
#27300=CARTESIAN_POINT ( 'NONE',  ( 16.06675444876397307, -9.020011618195203695, -1.000005633855494125E-09 ) ) ;
#27302=B_SPLINE_CURVE_WITH_KNOTS ( 'NONE', 5,
 ( #29105, #18894, #174, #24089, #2528, #21722, #6929, #9918, #9757 ),
 .UNSPECIFIED., .F., .F.,
 ( 6, 3, 6 ),
 ( 0.000000000000000000, 53.95537973340000093, 92.42745556099998794 ),
 .UNSPECIFIED. ) ;
#27310=B_SPLINE_CURVE_WITH_KNOTS ( 'NONE', 3,
 ( #22400, #22556, #698, #7904, #7605, #15152, #847, #20030, #12947, #10438, #29628, #8057, #17653, #27265, #5702, #15310, #24913, #9820 ),
 .UNSPECIFIED., .F., .F.,
 ( 4, 2, 2, 2, 2, 2, 2, 2, 4 ),
 ( 0.000000000000000000, 0.1250000000000000000, 0.2500000000000000000, 0.3750000000000000000, 0.5000000000000000000, 0.6250000000000000000, 0.7500000000000000000, 0.8750000000000000000, 1.000000000000000000 ),
 .UNSPECIFIED. ) ;
#27312=CARTESIAN_POINT ( 'NONE',  ( 0.1352650258152492124, -28.50015511220863118, 6.042326290000010758 ) ) ;
#27319=VERTEX_POINT ( 'NONE', #15220 ) ;
#27321=CARTESIAN_POINT ( 'NONE',  ( 27.95617443546494130, -9.697638328662621987, 0.7069222069999991920 ) ) ;
#27332=CARTESIAN_POINT ( 'NONE',  ( 24.32472894995379420, -13.45989151107506387, 6.099998581000020792 ) ) ;
#27336=CARTESIAN_POINT ( 'NONE',  ( 24.66346747934186112, 14.28208995963568739, 3.997248600000002927 ) ) ;
#27337=EDGE_CURVE ( 'NONE', #6458, #15510, #5397, .T. ) ;
#27353=ORIENTED_EDGE ( 'NONE', *, *, #13149, .F. ) ;
#27357=ORIENTED_EDGE ( 'NONE', *, *, #291, .F. ) ;
#27361=EDGE_LOOP ( 'NONE', ( #9876, #887, #12101, #23843 ) ) ;
#27363=CARTESIAN_POINT ( 'NONE',  ( -17.86397328150795971, -9.404917770633179686, 0.000000000000000000 ) ) ;
#27371=CARTESIAN_POINT ( 'NONE',  ( 23.81776757409229361, 15.65134803726813217, 4.999998581000003384 ) ) ;
#27383=CARTESIAN_POINT ( 'NONE',  ( 25.33584480268815042, 14.29478671867460982, 1.000000000000000888 ) ) ;
#27387=CARTESIAN_POINT ( 'NONE',  ( 23.23277125981546476, 15.26692728828886025, 4.999998581000003384 ) ) ;
#27389=VERTEX_POINT ( 'NONE', #17423 ) ;
#27396=VERTEX_POINT ( 'NONE', #12550 ) ;
#27400=CARTESIAN_POINT ( 'NONE',  ( -17.59696597926837214, -9.791839085300418688, -0.6999999999999784173 ) ) ;
#27404=CARTESIAN_POINT ( 'NONE',  ( -17.83929479963776288, 19.99998902616253105, -0.6999999999999784173 ) ) ;
#27417=CARTESIAN_POINT ( 'NONE',  ( -16.06988921231594603, 11.79183908526949054, 0.000000000000000000 ) ) ;
#27421=CARTESIAN_POINT ( 'NONE',  ( -24.90302310912370132, 13.86047864606265279, 6.098655051000018368 ) ) ;
#27425=CARTESIAN_POINT ( 'NONE',  ( -17.93344248771828475, 20.10553726043776734, 0.000000000000000000 ) ) ;
#27442=CARTESIAN_POINT ( 'NONE',  ( 24.43008698959658176, -14.67811372800087000, 4.492876031999992748 ) ) ;
#27448=CARTESIAN_POINT ( 'NONE',  ( 27.77052805885580966, 0.5052956280425284774, 0.7069222069999991920 ) ) ;
#27454=CARTESIAN_POINT ( 'NONE',  ( 23.77307140678977504, -14.41181874416537134, 4.999998581000003384 ) ) ;
#27456=EDGE_CURVE ( 'NONE', #26584, #30026, #519, .T. ) ;
#27466=ORIENTED_EDGE ( 'NONE', *, *, #30961, .T. ) ;
#27468=EDGE_LOOP ( 'NONE', ( #23030, #23769, #295, #6343, #7845, #12311, #3427, #3940 ) ) ;
#27469=CARTESIAN_POINT ( 'NONE',  ( 27.98121187870611593, -9.706323496128696604, 0.8585786439999909536 ) ) ;
#27470=ORIENTED_EDGE ( 'NONE', *, *, #5836, .F. ) ;
#27474=CARTESIAN_POINT ( 'NONE',  ( 17.83931306984926835, 20.00000000000176570, -0.6999999999999784173 ) ) ;
#27475=CARTESIAN_POINT ( 'NONE',  ( 24.63375101535647360, -12.88633855010671247, 5.901400366999986602 ) ) ;
#27488=CARTESIAN_POINT ( 'NONE',  ( 17.16657240421717390, -9.000000000001264766, -0.6999999999999784173 ) ) ;
#27492=EDGE_CURVE ( 'NONE', #25227, #12548, #23247, .T. ) ;
#27493=CARTESIAN_POINT ( 'NONE',  ( 0.5184513693225726305, -28.49550581263314086, 6.099998581000020792 ) ) ;
#27498=EDGE_LOOP ( 'NONE', ( #29721, #11224, #31, #7879 ) ) ;
#27506=CARTESIAN_POINT ( 'NONE',  ( 24.05769993097482029, 13.93129956292569638, 3.997248600000002927 ) ) ;
#27510=B_SPLINE_CURVE_WITH_KNOTS ( 'NONE', 3,
 ( #2227, #28335, #26603, #23947, #6784, #12118, #21261, #26, #21726, #26449, #26143, #9609, #7094, #14651, #24093, #16380, #19207, #26292, #2070, #31013, #2681, #25987, #24236, #2383, #23634, #19052, #178, #30862, #28650, #28494, #4893, #11661, #9294, #28792, #5041, #4427, #18897, #16682, #14030, #4736, #4576, #9762, #19368, #28958 ),
 .UNSPECIFIED., .F., .F.,
 ( 4, 2, 2, 1, 2, 2, 2, 2, 1, 1, 2, 2, 2, 2, 1, 1, 1, 2, 2, 2, 2, 1, 1, 2, 2, 4 ),
 ( 0.000000000000000000, 0.06250000000003701206, 0.09375000000005716261, 0.1093750000000685701, 0.1171875000000742878, 0.1250000000000799916, 0.1875000000001231792, 0.2187500000001463274, 0.2343750000001579292, 0.2421875000001617317, 0.2460937500001615930, 0.2500000000001614264, 0.3750000000001613154, 0.4375000000001627587, 0.4687500000001635359, 0.4843750000001654787, 0.4921875000001664779, 0.4960937500001669220, 0.5000000000001674216, 0.6250000000001194600, 0.6875000000000943690, 0.7187500000000829337, 0.7343750000000781597, 0.7421875000000758282, 0.7500000000000733857, 1.000000000000000000 ),
 .UNSPECIFIED. ) ;
#27517=CARTESIAN_POINT ( 'NONE',  ( -20.30403093128963476, 20.00000000003735323, 3.000000106999994642 ) ) ;
#27524=CARTESIAN_POINT ( 'NONE',  ( -28.35945636601969611, -7.983396444588293228, 8.000000000000007105 ) ) ;
#27528=CARTESIAN_POINT ( 'NONE',  ( 18.87721748640135644, 21.16361474300574841, 0.2374258030000131470 ) ) ;
#27546=EDGE_LOOP ( 'NONE', ( #12104, #15601, #27694, #2591, #4107, #7686, #16905, #6039 ) ) ;
#27553=SURFACE_STYLE_FILL_AREA ( #10574 ) ;
#27554=CARTESIAN_POINT ( 'NONE',  ( -24.37451445311242892, 13.36962324138351299, 6.095967861000000987 ) ) ;
#27555=CARTESIAN_POINT ( 'NONE',  ( -0.6094664100040195764, -28.49364619262437870, 4.999998581000003384 ) ) ;
#27560=CARTESIAN_POINT ( 'NONE',  ( -17.62526668112344908, -8.236461616547455122, -0.6999999999999784173 ) ) ;
#27575=EDGE_CURVE ( 'NONE', #4259, #3218, #1376, .T. ) ;
#27578=EDGE_CURVE ( 'NONE', #16829, #17637, #5727, .T. ) ;
#27589=CARTESIAN_POINT ( 'NONE',  ( -24.88589369081283920, 13.89120818323882922, 3.904029272000009154 ) ) ;
#27592=CARTESIAN_POINT ( 'NONE',  ( 1.360000222151617422, -28.46784699774883975, 5.735069644430439872 ) ) ;
#27594=CARTESIAN_POINT ( 'NONE',  ( -22.62479587716747886, 18.00962536160662708, 0.7595836940000044724 ) ) ;
#27601=CARTESIAN_POINT ( 'NONE',  ( 24.52721838744982463, -14.51532614974687796, 4.239732040000027347 ) ) ;
#27607=CARTESIAN_POINT ( 'NONE',  ( 27.71196445724500990, 5.091237891590008502, 1.000000000000000888 ) ) ;
#27625=CARTESIAN_POINT ( 'NONE',  ( 14.11260095516644242, -27.08984601216539190, 0.2686766510000271335 ) ) ;
#27632=B_SPLINE_CURVE_WITH_KNOTS ( 'NONE', 3,
 ( #123, #2477, #2327, #26087, #11909, #21826 ),
 .UNSPECIFIED., .F., .F.,
 ( 4, 2, 4 ),
 ( 0.000000000000000000, 0.5000000000000000000, 1.000000000000000000 ),
 .UNSPECIFIED. ) ;
#27636=CARTESIAN_POINT ( 'NONE',  ( 20.77600629932058851, 21.68409807857665683, 8.000000000000007105 ) ) ;
#27655=ORIENTED_EDGE ( 'NONE', *, *, #15676, .T. ) ;
#27665=CARTESIAN_POINT ( 'NONE',  ( -0.3176897050407275214, -27.79840873693312631, 5.732747703400294270 ) ) ;
#27668=CARTESIAN_POINT ( 'NONE',  ( -27.79539923781770483, -0.5057481688778130424, 0.8585786439999909536 ) ) ;
#27682=CARTESIAN_POINT ( 'NONE',  ( 22.44263053747149783, 18.11531079112418752, 0.5017677510000262409 ) ) ;
#27684=CARTESIAN_POINT ( 'NONE',  ( 21.02336020643863179, 19.26966202639587067, 4.000000000000003553 ) ) ;
#27688=FACE_OUTER_BOUND ( 'NONE', #2863, .T. ) ;
#27694=ORIENTED_EDGE ( 'NONE', *, *, #30349, .T. ) ;
#27704=CARTESIAN_POINT ( 'NONE',  ( -24.34138990045594042, 13.42981243766085164, 6.099998581000020792 ) ) ;
#27716=VECTOR ( 'NONE', #16711, 1000.000000000000000 ) ;
#27717=B_SPLINE_CURVE_WITH_KNOTS ( 'NONE', 5,
 ( #30328, #1847, #16314, #18667, #9222, #18981, #2159, #21194, #4663, #9693, #26225, #28731 ),
 .UNSPECIFIED., .F., .F.,
 ( 6, 3, 3, 6 ),
 ( 1.224410044450000123, 1.456395030499999965, 2.184590855310000190, 2.448622034100000011 ),
 .UNSPECIFIED. ) ;
#27744=CARTESIAN_POINT ( 'NONE',  ( 24.90302311548996883, -13.86047864964742793, 6.098655051000018368 ) ) ;
#27752=CARTESIAN_POINT ( 'NONE',  ( -25.44662322720032677, 12.83524168051548564, 4.689351480999998323 ) ) ;
#27763=CARTESIAN_POINT ( 'NONE',  ( -23.69427943501400691, -14.54081806258934861, 6.079851352000009257 ) ) ;
#27764=CARTESIAN_POINT ( 'NONE',  ( 21.85863980187338740, 17.64392717939186284, 0.5514269750000189152 ) ) ;
#27770=CARTESIAN_POINT ( 'NONE',  ( 24.81746042554890863, -14.01353061607344053, 3.920132063000014710 ) ) ;
#27774=CARTESIAN_POINT ( 'NONE',  ( -23.77307140041805411, 14.41181874028064591, 4.999998581000003384 ) ) ;
#27795=DIRECTION ( 'NONE',  ( 0.000000000000000000, 0.000000000000000000, -1.000000000000000000 ) ) ;
#27799=CARTESIAN_POINT ( 'NONE',  ( 27.07818553041514065, 6.807801137122736712, 8.000000000000007105 ) ) ;
#27800=VECTOR ( 'NONE', #4631, 1000.000000000000000 ) ;
#27805=CARTESIAN_POINT ( 'NONE',  ( -16.85343921394901301, 12.09981795542885585, -1.000005633855494125E-09 ) ) ;
#27811=CARTESIAN_POINT ( 'NONE',  ( -27.79539923781770483, -0.5057481688778011630, 1.000000000000000888 ) ) ;
#27838=CARTESIAN_POINT ( 'NONE',  ( 26.79556473285982321, 0.4875557887250580036, -0.6999999999999784173 ) ) ;
#27841=CARTESIAN_POINT ( 'NONE',  ( 13.21383179760920967, -25.42848403399915469, 8.000000000000007105 ) ) ;
#27842=FACE_OUTER_BOUND ( 'NONE', #19624, .T. ) ;
#27846=DIRECTION ( 'NONE',  ( 0.000000000000000000, 0.000000000000000000, -1.000000000000000000 ) ) ;
#27848=CARTESIAN_POINT ( 'NONE',  ( -0.1464386043128553250, -27.80011885101413682, 4.099092748999999536 ) ) ;
#27851=B_SPLINE_CURVE_WITH_KNOTS ( 'NONE', 3,
 ( #10382, #3591, #19973, #24697, #20276, #17452 ),
 .UNSPECIFIED., .F., .F.,
 ( 4, 2, 4 ),
 ( 0.000000000000000000, 0.5000000000000000000, 1.000000000000000000 ),
 .UNSPECIFIED. ) ;
#27852=CARTESIAN_POINT ( 'NONE',  ( 23.62421573330318836, 14.65442405561991634, 6.042470792000015578 ) ) ;
#27875=CARTESIAN_POINT ( 'NONE',  ( 23.88966196158443367, -14.21810147650477596, 4.317391451927520940 ) ) ;
#27876=ADVANCED_FACE ( 'NONE', ( #19914 ), #14572, .F. ) ;
#27883=CARTESIAN_POINT ( 'NONE',  ( 24.37450210455010335, -13.36961646745188759, 6.095967861000000987 ) ) ;
#27890=CARTESIAN_POINT ( 'NONE',  ( -17.80313299384375370, 11.53824530455753283, -0.6999999999999785283 ) ) ;
#27915=CARTESIAN_POINT ( 'NONE',  ( -18.97090238747512458, 21.26865671932805313, 0.7595836940000044724 ) ) ;
#27918=CARTESIAN_POINT ( 'NONE',  ( -23.81776757772072983, -15.65134804123479917, 4.999998581000003384 ) ) ;
#27923=EDGE_CURVE ( 'NONE', #21696, #19663, #21850, .T. ) ;
#27930=CARTESIAN_POINT ( 'NONE',  ( 26.68292649568627084, 9.659560297568411613, 1.000000000000000888 ) ) ;
#27932=CARTESIAN_POINT ( 'NONE',  ( -17.62526623054365871, -8.236462051082252600, 0.000000000000000000 ) ) ;
#27936=CARTESIAN_POINT ( 'NONE',  ( 23.92481352790954929, -14.15879618172946408, 4.239732040000027347 ) ) ;
#27937=CARTESIAN_POINT ( 'NONE',  ( 18.26639035964474900, 11.02001161816309072, -1.000005633855494125E-09 ) ) ;
#27956=CARTESIAN_POINT ( 'NONE',  ( -0.5968465743326634154, -28.49391676915515603, 4.791896188000022150 ) ) ;
#27957=CARTESIAN_POINT ( 'NONE',  ( -16.34545256226243382, -9.995493785995851255, 0.000000000000000000 ) ) ;
#27961=CARTESIAN_POINT ( 'NONE',  ( 27.75695160390876737, 2.618790587933454983, 8.000000000000007105 ) ) ;
#27966=CARTESIAN_POINT ( 'NONE',  ( 23.35349940196098828, 15.08195766973940266, 4.323494425288421539 ) ) ;
#27981=PRODUCT_CONTEXT ( 'NONE', #12183, 'mechanical' ) ;
#27997=CARTESIAN_POINT ( 'NONE',  ( 28.54410101353736806, -9.901582551596423087, 0.2374258030000131470 ) ) ;
#27999=CARTESIAN_POINT ( 'NONE',  ( -7.974365406319376071, -26.79131034418178814, 8.000000000000007105 ) ) ;
#28003=CARTESIAN_POINT ( 'NONE',  ( 27.21178567695783812, 4.999345137307622089, -0.6577119969999878357 ) ) ;
#28005=CARTESIAN_POINT ( 'NONE',  ( -22.97593529893700648, 15.65128280014837081, 8.000000000000007105 ) ) ;
#28010=DIRECTION ( 'NONE',  ( 0.000000000000000000, 0.000000000000000000, -1.000000000000000000 ) ) ;
#28026=CARTESIAN_POINT ( 'NONE',  ( 24.32472724076343695, -13.45989056521276872, 3.899998581000013509 ) ) ;
#28050=ORIENTED_EDGE ( 'NONE', *, *, #795, .F. ) ;
#28061=ADVANCED_FACE ( 'NONE', ( #6673 ), #257, .F. ) ;
#28069=CARTESIAN_POINT ( 'NONE',  ( -20.30403093151401706, 20.00000000001585221, 0.8732882910316148717 ) ) ;
#28076=CARTESIAN_POINT ( 'NONE',  ( 0.9758793680739014098, -27.78334643823060546, 3.997481721999984750 ) ) ;
#28077=CARTESIAN_POINT ( 'NONE',  ( 18.26375984408715425, 11.16458205341174192, -0.6999999999999783062 ) ) ;
#28079=CARTESIAN_POINT ( 'NONE',  ( 27.52676963214412353, 0.5008603480660110963, 0.2686740700000300741 ) ) ;
#28083=CARTESIAN_POINT ( 'NONE',  ( -23.25311087912443853, -15.23597700045676895, 5.310552105000033052 ) ) ;
#28086=CARTESIAN_POINT ( 'NONE',  ( 24.30808045080437907, -13.48997717272881047, 3.899998581000013509 ) ) ;
#28104=CARTESIAN_POINT ( 'NONE',  ( -26.66783967069105898, -7.507193849635574345, 0.000000000000000000 ) ) ;
#28110=CARTESIAN_POINT ( 'NONE',  ( -3.448453739143383601, 0.7497105383095263864, 0.000000000000000000 ) ) ;
#28111=CARTESIAN_POINT ( 'NONE',  ( 0.4125558677724673329, -28.49726274111925761, 3.904047916000019658 ) ) ;
#28115=VERTEX_POINT ( 'NONE', #14546 ) ;
#28116=CARTESIAN_POINT ( 'NONE',  ( 0.000000000000000000, 0.000000000000000000, -0.6999999999999784173 ) ) ;
#28123=CARTESIAN_POINT ( 'NONE',  ( 23.23277120357798964, 15.26692725135965745, 4.999998581000003384 ) ) ;
#28128=CARTESIAN_POINT ( 'NONE',  ( 25.46368747440213198, -12.80129684534102807, 4.999998581000003384 ) ) ;
#28130=CARTESIAN_POINT ( 'NONE',  ( -17.49164322995629917, 10.10662636424719807, 0.000000000000000000 ) ) ;
#28132=ORIENTED_EDGE ( 'NONE', *, *, #21946, .F. ) ;
#28134=EDGE_LOOP ( 'NONE', ( #13731, #27655, #30549, #10915 ) ) ;
#28141=ORIENTED_EDGE ( 'NONE', *, *, #9395, .F. ) ;
#28148=CARTESIAN_POINT ( 'NONE',  ( -17.52531973950389244, 11.86718987797331160, -4.336808689942017736E-16 ) ) ;
#28157=CARTESIAN_POINT ( 'NONE',  ( 26.97469346668950152, -9.357175201752722771, -0.6999999999999784173 ) ) ;
#28158=CARTESIAN_POINT ( 'NONE',  ( -19.76607646299421361, 19.51851687837242366, 0.7753390690000139251 ) ) ;
#28159=CARTESIAN_POINT ( 'NONE',  ( -28.49530731802708061, -0.5184832703812680688, 8.000000000000007105 ) ) ;
#28161=CARTESIAN_POINT ( 'NONE',  ( 27.35479945376024347, 9.902747534584010580, 1.000000000000000888 ) ) ;
#28163=CARTESIAN_POINT ( 'NONE',  ( -0.3000709590666145732, -27.79870762326800104, 4.240370246000018994 ) ) ;
#28166=ORIENTED_EDGE ( 'NONE', *, *, #14593, .F. ) ;
#28173=ORIENTED_EDGE ( 'NONE', *, *, #25272, .F. ) ;
#28174=ORIENTED_EDGE ( 'NONE', *, *, #7753, .F. ) ;
#28176=EDGE_LOOP ( 'NONE', ( #5371, #11681, #19397, #22675 ) ) ;
#28179=CARTESIAN_POINT ( 'NONE',  ( -24.36375418918093061, -14.78716628874576244, 3.904032100999987875 ) ) ;
#28181=CARTESIAN_POINT ( 'NONE',  ( 17.82645929464983681, -8.108213974639840060, -4.336808689942018722E-16 ) ) ;
#28196=CARTESIAN_POINT ( 'NONE',  ( 1.632956991020356519, -28.45346066249067007, 5.208113774000016960 ) ) ;
#28203=CARTESIAN_POINT ( 'NONE',  ( 0.5890437901233029905, -28.49417040867363227, 3.901346086000012647 ) ) ;
#28222=ORIENTED_EDGE ( 'NONE', *, *, #3307, .T. ) ;
#28223=CARTESIAN_POINT ( 'NONE',  ( -19.20306644830689891, 20.00029701457494369, -0.4291057264425030549 ) ) ;
#28230=CARTESIAN_POINT ( 'NONE',  ( 18.11692203337192097, 11.57288288306469148, -0.6999999999999784173 ) ) ;
#28232=CARTESIAN_POINT ( 'NONE',  ( -23.81776757772072983, -15.65134804123479917, 4.999998581000003384 ) ) ;
#28245=B_SPLINE_CURVE_WITH_KNOTS ( 'NONE', 1,
 ( #10053, #16811 ),
 .UNSPECIFIED., .F., .F.,
 ( 2, 2 ),
 ( -2.557301831960000071E-06, 0.7000000000009999335 ),
 .UNSPECIFIED. ) ;
#28251=CARTESIAN_POINT ( 'NONE',  ( -17.83930458849792089, 19.99999999999597478, -1.000005633855494125E-09 ) ) ;
#28273=CARTESIAN_POINT ( 'NONE',  ( 23.67037533738476540, 14.57986020592288234, 3.928017074518106888 ) ) ;
#28286=ORIENTED_EDGE ( 'NONE', *, *, #12985, .T. ) ;
#28290=ORIENTED_EDGE ( 'NONE', *, *, #5748, .T. ) ;
#28297=CARTESIAN_POINT ( 'NONE',  ( 27.98121187870611593, -9.706323496128696604, 8.000000000000007105 ) ) ;
#28303=CARTESIAN_POINT ( 'NONE',  ( 25.46368747440213198, -12.80129684534102807, 4.999998581000003384 ) ) ;
#28307=CARTESIAN_POINT ( 'NONE',  ( 28.03861306157277866, 0.5101735396241827702, -0.2432540810000105580 ) ) ;
#28309=CARTESIAN_POINT ( 'NONE',  ( -25.43411672857565264, -11.59571042436485655, 8.000000000000007105 ) ) ;
#28327=ADVANCED_FACE ( 'NONE', ( #1927 ), #5014, .F. ) ;
#28328=ORIENTED_EDGE ( 'NONE', *, *, #15423, .F. ) ;
#28332=FACE_OUTER_BOUND ( 'NONE', #25710, .T. ) ;
#28333=CARTESIAN_POINT ( 'NONE',  ( -23.81776757772072983, -15.65134804123479917, 4.895813258999987205 ) ) ;
#28335=CARTESIAN_POINT ( 'NONE',  ( 17.87667150816518102, 20.00000000000230926, -0.6999999999999783062 ) ) ;
#28341=ORIENTED_EDGE ( 'NONE', *, *, #30113, .T. ) ;
#28348=FACE_BOUND ( 'NONE', #27468, .T. ) ;
#28361=ORIENTED_EDGE ( 'NONE', *, *, #27923, .F. ) ;
#28382=DIRECTION ( 'NONE',  ( 0.000000000000000000, 0.000000000000000000, -1.000000000000000000 ) ) ;
#28387=CARTESIAN_POINT ( 'NONE',  ( -18.77172700302876507, 19.99998314052377069, -0.5795685437816225916 ) ) ;
#28394=CARTESIAN_POINT ( 'NONE',  ( 1.495522319887057749, -27.76012052182125345, 4.493506933999996455 ) ) ;
#28405=( GEOMETRIC_REPRESENTATION_CONTEXT ( 3 ) GLOBAL_UNCERTAINTY_ASSIGNED_CONTEXT ( ( #24818 ) ) GLOBAL_UNIT_ASSIGNED_CONTEXT ( ( #13550, #14027, #9130 ) ) REPRESENTATION_CONTEXT ( 'NONE', 'WORKASPACE' ) );
#28420=CARTESIAN_POINT ( 'NONE',  ( -0.3000709590666145732, -27.79870762326800104, 4.240370246000018994 ) ) ;
#28423=CARTESIAN_POINT ( 'NONE',  ( -23.55444264242456498, 16.04540112444970390, 8.000000000000007105 ) ) ;
#28425=CARTESIAN_POINT ( 'NONE',  ( -1.776062861149290062E-14, -3.231615895114969171E-16, -0.5999999999999894307 ) ) ;
#28429=ADVANCED_FACE ( 'NONE', ( #7710 ), #24369, .T. ) ;
#28431=CARTESIAN_POINT ( 'NONE',  ( 17.18658402241074867, -10.09981795543446736, -0.6999999999999784173 ) ) ;
#28434=CARTESIAN_POINT ( 'NONE',  ( -24.37450209798932477, 13.36961646417070249, 3.904029301000005781 ) ) ;
#28441=ORIENTED_EDGE ( 'NONE', *, *, #3459, .T. ) ;
#28446=ORIENTED_EDGE ( 'NONE', *, *, #29847, .F. ) ;
#28452=CARTESIAN_POINT ( 'NONE',  ( -27.79539923781684863, -0.5057481689249068157, 5.200000000000009948 ) ) ;
#28463=CARTESIAN_POINT ( 'NONE',  ( 26.07698513492398718, 11.88166128046557546, 8.000000000000007105 ) ) ;
#28465=CARTESIAN_POINT ( 'NONE',  ( 28.68577476828162531, -9.950727360111285336, 1.000000000000000888 ) ) ;
#28488=VERTEX_POINT ( 'NONE', #29735 ) ;
#28489=CARTESIAN_POINT ( 'NONE',  ( 17.29283780772782819, 12.10247952218883682, -0.6999999999999784173 ) ) ;
#28490=CARTESIAN_POINT ( 'NONE',  ( 23.39354070784786543, 15.01969649483752001, 4.239862992999999136 ) ) ;
#28494=CARTESIAN_POINT ( 'NONE',  ( 19.40803489293128692, 20.00003047048157256, -0.3219712011826995068 ) ) ;
#28512=B_SPLINE_CURVE_WITH_KNOTS ( 'NONE', 1,
 ( #6718, #16322 ),
 .UNSPECIFIED., .F., .F.,
 ( 2, 2 ),
 ( -3.500000000000000000, 3.500000000000000000 ),
 .UNSPECIFIED. ) ;
#28515=CARTESIAN_POINT ( 'NONE',  ( 18.24300304067004674, 10.73161574555001607, -4.336808689942017243E-16 ) ) ;
#28527=DIRECTION ( 'NONE',  ( 0.6941258031311203780, 0.7198537139083029945, 0.000000000000000000 ) ) ;
#28538=CARTESIAN_POINT ( 'NONE',  ( -19.58511357176576340, 20.00016057457926522, -0.2119832659756666626 ) ) ;
#28540=CARTESIAN_POINT ( 'NONE',  ( 18.26905192694325208, -9.126265403884737282, -0.6999999999999784173 ) ) ;
#28551=EDGE_CURVE ( 'NONE', #25281, #30700, #7567, .T. ) ;
#28560=CARTESIAN_POINT ( 'NONE',  ( -27.79539923781684863, -0.5057481689248934931, 1.000000000000000888 ) ) ;
#28562=B_SPLINE_CURVE_WITH_KNOTS ( 'NONE', 5,
 ( #8550, #6038, #13119, #15958, #20520, #30120, #18148, #1494, #10765, #25089, #29798, #27752, #6200, #8232, #3847 ),
 .UNSPECIFIED., .F., .F.,
 ( 6, 3, 3, 3, 6 ),
 ( 0.000000000000000000, 0.1000000000028631597, 0.3999999999999999667, 0.7000000000005724976, 1.000000000000000000 ),
 .UNSPECIFIED. ) ;
#28571=CARTESIAN_POINT ( 'NONE',  ( -26.84172470026987867, 2.049348509503662097, 0.000000000000000000 ) ) ;
#28576=VECTOR ( 'NONE', #27282, 1000.000000000000000 ) ;
#28580=CARTESIAN_POINT ( 'NONE',  ( -0.5716039300045591132, -28.49445895580208443, 4.689815098000011062 ) ) ;
#28588=CARTESIAN_POINT ( 'NONE',  ( 16.50668551557458485, -9.891786026617527483, -0.6999999999999784173 ) ) ;
#28597=CARTESIAN_POINT ( 'NONE',  ( -16.74153468538860068, -7.902894514795387515, 0.000000000000000000 ) ) ;
#28612=ADVANCED_FACE ( 'NONE', ( #9108 ), #14829, .F. ) ;
#28616=CARTESIAN_POINT ( 'NONE',  ( -20.30403093128963476, 20.00000000003735323, 1.000000000000000888 ) ) ;
#28620=DIRECTION ( 'NONE',  ( 0.000000000000000000, 0.000000000000000000, -1.000000000000000000 ) ) ;
#28623=CARTESIAN_POINT ( 'NONE',  ( 24.82162974202869421, -12.51998933900577349, 5.310645680000003921 ) ) ;
#28626=CARTESIAN_POINT ( 'NONE',  ( -19.76607646299421361, 19.51851687837242366, 0.7753390690000139251 ) ) ;
#28632=EDGE_LOOP ( 'NONE', ( #3506, #29434, #27012, #16551, #20244, #2097, #10413, #16709 ) ) ;
#28634=CARTESIAN_POINT ( 'NONE',  ( -15.75643827102668482, -9.267172193162394933, -0.6999999999999784173 ) ) ;
#28645=FACE_OUTER_BOUND ( 'NONE', #20504, .T. ) ;
#28646=CARTESIAN_POINT ( 'NONE',  ( 23.81866173088643635, 14.33570044285385947, 3.899998581000013509 ) ) ;
#28650=CARTESIAN_POINT ( 'NONE',  ( 19.40179356770304864, 20.00003053714920043, -0.3254732509765126403 ) ) ;
#28653=FACE_OUTER_BOUND ( 'NONE', #27090, .T. ) ;
#28656=CARTESIAN_POINT ( 'NONE',  ( -16.06988964647317886, -8.208161364834239748, 0.000000000000000000 ) ) ;
#28659=EDGE_CURVE ( 'NONE', #12806, #17991, #13921, .T. ) ;
#28660=CARTESIAN_POINT ( 'NONE',  ( 24.14840829003134104, 13.77363891352294267, 5.901294549000013490 ) ) ;
#28666=CARTESIAN_POINT ( 'NONE',  ( 16.09014176753201752, 11.26838425375450115, -4.336808689942017243E-16 ) ) ;
#28672=VERTEX_POINT ( 'NONE', #17846 ) ;
#28674=CARTESIAN_POINT ( 'NONE',  ( 23.83861932470720291, 15.61961844235199948, 4.689445052000001724 ) ) ;
#28679=ORIENTED_EDGE ( 'NONE', *, *, #3232, .F. ) ;
#28692=CARTESIAN_POINT ( 'NONE',  ( -19.73536700009918121, 20.00033765927653917, -0.09955921259694186509 ) ) ;
#28702=B_SPLINE_CURVE_WITH_KNOTS ( 'NONE', 3,
 ( #15088, #777, #27044, #29398, #20121, #15233 ),
 .UNSPECIFIED., .F., .F.,
 ( 4, 2, 4 ),
 ( 0.000000000000000000, 0.5000000000000000000, 1.000000000000000000 ),
 .UNSPECIFIED. ) ;
#28704=CARTESIAN_POINT ( 'NONE',  ( 17.18658402241074867, -10.09981795543446736, -0.6999999999999784173 ) ) ;
#28707=CARTESIAN_POINT ( 'NONE',  ( 17.14656078602323319, -7.900182044548062166, -0.6999999999999784173 ) ) ;
#28708=CARTESIAN_POINT ( 'NONE',  ( -17.40631047800548004, -8.049650370842703850, -0.6999999999999784173 ) ) ;
#28709=CARTESIAN_POINT ( 'NONE',  ( -27.61317819196527878, 4.248065245814218294, 0.2686740700000300741 ) ) ;
#28720=EDGE_CURVE ( 'NONE', #25281, #26584, #5274, .T. ) ;
#28731=CARTESIAN_POINT ( 'NONE',  ( -15.73360964098195147, -8.979988381493612337, 0.000000000000000000 ) ) ;
#28733=CARTESIAN_POINT ( 'NONE',  ( 16.63016908727803056, -9.971084190299466243, -0.6999999999999784173 ) ) ;
#28755=CARTESIAN_POINT ( 'NONE',  ( -27.79539923781684507, -0.5057481689249112566, 2.400000000000013234 ) ) ;
#28756=CARTESIAN_POINT ( 'NONE',  ( -23.55444264242456498, 16.04540112444970390, 8.000000000000007105 ) ) ;
#28757=CARTESIAN_POINT ( 'NONE',  ( 19.80526555972147307, 19.50877392102524155, 3.000000000000002665 ) ) ;
#28766=CARTESIAN_POINT ( 'NONE',  ( 24.34137756859324853, -13.42980563341176037, 6.099998581000020792 ) ) ;
#28771=CARTESIAN_POINT ( 'NONE',  ( -24.98081131316241255, -13.71897606304888662, 4.999998581000003384 ) ) ;
#28772=CARTESIAN_POINT ( 'NONE',  ( -24.92639508767336309, -13.81781708088548122, 5.506973469000003618 ) ) ;
#28782=ORIENTED_EDGE ( 'NONE', *, *, #30813, .T. ) ;
#28790=FACE_BOUND ( 'NONE', #21255, .T. ) ;
#28792=CARTESIAN_POINT ( 'NONE',  ( 19.84014010780992621, 20.00037855652159990, -0.006061537342544804675 ) ) ;
#28793=CARTESIAN_POINT ( 'NONE',  ( -24.81746041937532965, 14.01353061208509310, 6.079865099000020479 ) ) ;
#28801=CARTESIAN_POINT ( 'NONE',  ( 19.49313413869766620, 19.58644549600961327, 0.4409083710000261114 ) ) ;
#28802=CARTESIAN_POINT ( 'NONE',  ( -16.85343921394901301, 12.09981795542885585, -0.6999999999999784173 ) ) ;
#28807=CARTESIAN_POINT ( 'NONE',  ( 23.78820504408419723, -14.38694252465835710, 5.289459540744400279 ) ) ;
#28812=CARTESIAN_POINT ( 'NONE',  ( 0.5537481963838299936, -28.49486543565701169, 3.899998581000013509 ) ) ;
#28816=CARTESIAN_POINT ( 'NONE',  ( 24.29089620522634263, 14.90695587088477581, 3.920145809000019632 ) ) ;
#28819=ORIENTED_EDGE ( 'NONE', *, *, #12985, .F. ) ;
#28833=CARTESIAN_POINT ( 'NONE',  ( 19.49313413869766620, 19.58644549600961327, 0.4409083710000261114 ) ) ;
#28837=CARTESIAN_POINT ( 'NONE',  ( -20.50713102034104551, 18.79635956957924492, 4.000000085000010586 ) ) ;
#28838=B_SPLINE_SURFACE_WITH_KNOTS ( 'NONE', 5, 1, ( 
 ( #29255, #2987 ),
 ( #12577, #4888 ),
 ( #5953, #24857 ),
 ( #946, #25318 ),
 ( #10535, #15402 ),
 ( #3132, #8306 ),
 ( #22646, #3286 ),
 ( #12890, #1089 ),
 ( #792, #27506 ),
 ( #17901, #27057 ),
 ( #13037, #12732 ),
 ( #25002, #29722 ),
 ( #5494, #22497 ),
 ( #5804, #13352 ),
 ( #10680, #15550 ) ),
 .UNSPECIFIED., .F., .F., .F.,
 ( 6, 3, 3, 3, 6 ),
 ( 2, 2 ),
 ( 0.000000000000000000, 0.5239010160460000343, 1.047802032090000113, 1.571703048140000059, 1.746336720149999966 ),
 ( -0.7000000000009999335, 2.556026163500000058E-06 ),
 .UNSPECIFIED. ) ;
#28848=EDGE_CURVE ( 'NONE', #11577, #27319, #16276, .T. ) ;
#28869=CARTESIAN_POINT ( 'NONE',  ( 0.9758793680739014098, -27.78334643823060546, 3.997481721999984750 ) ) ;
#28870=VERTEX_POINT ( 'NONE', #28704 ) ;
#28880=CARTESIAN_POINT ( 'NONE',  ( -23.57322167415998138, -14.73624932338542060, 3.997250019000003540 ) ) ;
#28887=CARTESIAN_POINT ( 'NONE',  ( 24.32472724076343695, -13.45989056521276872, 6.099998581000020792 ) ) ;
#28897=CYLINDRICAL_SURFACE ( 'NONE', #10750, 1.100000000000002309 ) ;
#28901=CARTESIAN_POINT ( 'NONE',  ( 23.23277120357798964, 15.26692725135965745, 4.999998581000003384 ) ) ;
#28904=EDGE_CURVE ( 'NONE', #20192, #14021, #21941, .T. ) ;
#28918=CARTESIAN_POINT ( 'NONE',  ( -24.37165444408190851, 14.77472139917419369, 4.895781291000017355 ) ) ;
#28920=B_SPLINE_CURVE_WITH_KNOTS ( 'NONE', 3,
 ( #30822, #1875, #25323, #21076, #28148, #16032 ),
 .UNSPECIFIED., .F., .F.,
 ( 4, 2, 4 ),
 ( 0.000000000000000000, 0.5000000000000000000, 1.000000000000000000 ),
 .UNSPECIFIED. ) ;
#28926=CYLINDRICAL_SURFACE ( 'NONE', #9984, 1.100000000000002309 ) ;
#28934=B_SPLINE_CURVE_WITH_KNOTS ( 'NONE', 3,
 ( #1550, #30959, #14596, #7350, #7190, #5299 ),
 .UNSPECIFIED., .F., .F.,
 ( 4, 2, 4 ),
 ( 0.000000000000000000, 0.5000000000000000000, 1.000000000000000000 ),
 .UNSPECIFIED. ) ;
#28938=CARTESIAN_POINT ( 'NONE',  ( -24.97472003774791816, -13.73006752753317450, 5.208359076000035337 ) ) ;
#28945=VERTEX_POINT ( 'NONE', #25538 ) ;
#28946=CARTESIAN_POINT ( 'NONE',  ( 25.35851007746311581, -13.00862288856444238, 4.319165765000021473 ) ) ;
#28958=CARTESIAN_POINT ( 'NONE',  ( 20.30396079652883756, 20.00000000004620304, 1.000000000000000888 ) ) ;
#28959=CARTESIAN_POINT ( 'NONE',  ( -24.27467683362817397, 13.55001165674122987, 6.095967889000020179 ) ) ;
#28967=CARTESIAN_POINT ( 'NONE',  ( 23.83006841374216833, -14.31758446293960141, 5.507121129000008608 ) ) ;
#28968=CARTESIAN_POINT ( 'NONE',  ( 19.36636234657989775, 19.99999973364792538, -0.3591601440000036227 ) ) ;
#28978=CARTESIAN_POINT ( 'NONE',  ( 18.03540948973492775, -8.309720466357155999, -0.6999999999999784173 ) ) ;
#28983=VERTEX_POINT ( 'NONE', #27417 ) ;
#28984=ORIENTED_EDGE ( 'NONE', *, *, #28720, .F. ) ;
#28996=ORIENTED_EDGE ( 'NONE', *, *, #29785, .T. ) ;
#28997=ADVANCED_FACE ( 'NONE', ( #8999 ), #26622, .T. ) ;
#28998=CARTESIAN_POINT ( 'NONE',  ( -21.17688367750145773, 18.05241592653123206, 5.000000064000004407 ) ) ;
#29006=CARTESIAN_POINT ( 'NONE',  ( -24.39492853991606225, 13.33306305658284430, 3.899998581000068132 ) ) ;
#29011=ORIENTED_EDGE ( 'NONE', *, *, #21350, .F. ) ;
#29014=CARTESIAN_POINT ( 'NONE',  ( -26.93696268452645981, -0.4901285798021789986, 0.000000000000000000 ) ) ;
#29023=CARTESIAN_POINT ( 'NONE',  ( 0.8794532062878365197, -27.78659480101269708, 3.957673652000032405 ) ) ;
#29030=B_SPLINE_SURFACE_WITH_KNOTS ( 'NONE', 5, 1, ( 
 ( #17467, #18076 ),
 ( #15116, #4088 ),
 ( #20764, #9110 ),
 ( #16197, #11169 ),
 ( #18710, #1581 ),
 ( #23610, #20606 ),
 ( #3934, #30372 ),
 ( #21235, #18232 ),
 ( #15891, #8800 ),
 ( #27841, #11016 ),
 ( #6598, #18402 ),
 ( #13527, #15721 ),
 ( #1885, #25811 ),
 ( #8959, #30834 ),
 ( #16046, #27999 ),
 ( #20927, #30529 ),
 ( #23139, #1422 ),
 ( #21087, #6443 ),
 ( #30204, #4246 ),
 ( #8636, #25658 ),
 ( #2046, #28309 ),
 ( #23289, #13367 ),
 ( #25335, #6292 ),
 ( #1734, #13686 ),
 ( #25962, #13845 ),
 ( #11330, #18558 ),
 ( #28159, #11636 ) ),
 .UNSPECIFIED., .F., .F., .F.,
 ( 6, 3, 3, 3, 3, 3, 3, 3, 6 ),
 ( 2, 2 ),
 ( 0.000000000000000000, 12.04914910469999967, 24.12830621100000172, 36.22018076730000047, 48.28758829720000278, 60.33208762030000116, 72.38455155859999479, 84.43687076610000020, 88.75867308210000317 ),
 ( -2.393070191420000080E-05, 0.7036780443879999680 ),
 .UNSPECIFIED. ) ;
#29039=CARTESIAN_POINT ( 'NONE',  ( -24.22405393111669980, -13.63981656684929078, 5.760125276000005456 ) ) ;
#29046=CARTESIAN_POINT ( 'NONE',  ( -20.77600556902951823, -21.68409854416798410, 0.7595836940000044724 ) ) ;
#29049=CARTESIAN_POINT ( 'NONE',  ( -4.785279987099964494, -31.71089578132184883, 8.000000000000007105 ) ) ;
#29062=VERTEX_POINT ( 'NONE', #11524 ) ;
#29063=VERTEX_POINT ( 'NONE', #26312 ) ;
#29069=CARTESIAN_POINT ( 'NONE',  ( -24.52721838136531574, 14.51532614515681097, 4.239732039000021047 ) ) ;
#29071=CARTESIAN_POINT ( 'NONE',  ( -19.80535357377644701, 19.50875577052588739, 1.400000021000019634 ) ) ;
#29075=DIRECTION ( 'NONE',  ( -0.7198537139083028835, 0.6941258031311204890, 0.000000000000000000 ) ) ;
#29076=CARTESIAN_POINT ( 'NONE',  ( -24.61381496313306982, -14.36755986783020056, 3.957524336000023624 ) ) ;
#29077=ADVANCED_FACE ( 'NONE', ( #20811 ), #21862, .T. ) ;
#29082=B_SPLINE_CURVE_WITH_KNOTS ( 'NONE', 3,
 ( #7425, #26624, #14675, #24261, #2706, #4456 ),
 .UNSPECIFIED., .F., .F.,
 ( 4, 2, 4 ),
 ( 0.000000000000000000, 0.5000000000000000000, 1.000000000000000000 ),
 .UNSPECIFIED. ) ;
#29097=ORIENTED_EDGE ( 'NONE', *, *, #15087, .F. ) ;
#29104=ORIENTED_EDGE ( 'NONE', *, *, #7045, .F. ) ;
#29105=CARTESIAN_POINT ( 'NONE',  ( 27.79539923781684507, 0.5057481689249130330, 1.000000000000000888 ) ) ;
#29112=CARTESIAN_POINT ( 'NONE',  ( -24.49145440957854802, 14.57548795260905550, 5.680829343999993952 ) ) ;
#29119=CARTESIAN_POINT ( 'NONE',  ( 24.52721838744800920, -14.51532614964689394, 5.760265122000007842 ) ) ;
#29120=CARTESIAN_POINT ( 'NONE',  ( 23.94167923218613225, 14.12976891125826029, 6.079852602000002548 ) ) ;
#29123=CARTESIAN_POINT ( 'NONE',  ( 1.311146135488785669, -27.76947565999227763, 5.759639119000015128 ) ) ;
#29140=CARTESIAN_POINT ( 'NONE',  ( -16.29518228970498583, 11.96970539749145068, -0.6999999999999785283 ) ) ;
#29164=CARTESIAN_POINT ( 'NONE',  ( -26.79556473285982321, -0.4875557887251183442, -0.6999999999999784173 ) ) ;
#29172=ORIENTED_EDGE ( 'NONE', *, *, #2374, .T. ) ;
#29183=ORIENTED_EDGE ( 'NONE', *, *, #3459, .F. ) ;
#29190=CARTESIAN_POINT ( 'NONE',  ( -17.05870563379187033, -7.915918418981195970, 0.000000000000000000 ) ) ;
#29192=CARTESIAN_POINT ( 'NONE',  ( -25.36600720539997766, -15.15696894355576241, -0.2432540810000105580 ) ) ;
#29200=EDGE_LOOP ( 'NONE', ( #19578, #13184, #3257, #2514 ) ) ;
#29202=CARTESIAN_POINT ( 'NONE',  ( 20.30396079662882158, 20.00000000004802203, 1.400000000000012346 ) ) ;
#29203=DIRECTION ( 'NONE',  ( 1.000000000000000000, 0.000000000000000000, 0.000000000000000000 ) ) ;
#29214=CARTESIAN_POINT ( 'NONE',  ( -24.00289803497245700, 14.02635913871703011, 4.098597478000010064 ) ) ;
#29236=CARTESIAN_POINT ( 'NONE',  ( -24.93720648713954446, 13.79881813474513486, 6.099998581000020792 ) ) ;
#29242=VERTEX_POINT ( 'NONE', #27228 ) ;
#29245=CARTESIAN_POINT ( 'NONE',  ( 25.12046395012945155, -13.46291002088068289, 3.957489296000010981 ) ) ;
#29248=EDGE_CURVE ( 'NONE', #25714, #28115, #12753, .T. ) ;
#29251=ORIENTED_EDGE ( 'NONE', *, *, #24471, .T. ) ;
#29255=CARTESIAN_POINT ( 'NONE',  ( 24.98081130624543889, 13.71897605842228529, 4.999998581000003384 ) ) ;
#29268=CARTESIAN_POINT ( 'NONE',  ( 24.20792487550426841, -13.66932880343719781, 6.079865098000015067 ) ) ;
#29273=CARTESIAN_POINT ( 'NONE',  ( 1.157672466183025994, -27.77645868488734138, 5.900907654000003610 ) ) ;
#29275=CARTESIAN_POINT ( 'NONE',  ( -24.34942396232675321, -13.41447636113284680, 4.689458291000009105 ) ) ;
#29291=EDGE_LOOP ( 'NONE', ( #3273, #28984, #26782, #1152 ) ) ;
#29296=CARTESIAN_POINT ( 'NONE',  ( -25.12046394328145382, 13.46291001830483580, 6.042507865999996675 ) ) ;
#29307=CARTESIAN_POINT ( 'NONE',  ( 23.34136241352823404, 16.91641428746209286, 1.000000000000000888 ) ) ;
#29315=B_SPLINE_CURVE_WITH_KNOTS ( 'NONE', 3,
 ( #18837, #18528, #20737, #1391, #28130, #30804 ),
 .UNSPECIFIED., .F., .F.,
 ( 4, 2, 4 ),
 ( 0.000000000000000000, 0.5000000000000000000, 1.000000000000000000 ),
 .UNSPECIFIED. ) ;
#29317=CARTESIAN_POINT ( 'NONE',  ( 22.63260994176697238, -19.28417101125922883, -0.6999999999999784173 ) ) ;
#29332=CARTESIAN_POINT ( 'NONE',  ( -25.45339887876027163, 13.89659413885661365, 0.2374258030000131470 ) ) ;
#29338=AXIS2_PLACEMENT_3D ( 'NONE', #18164, #20222, #20535 ) ;
#29343=AXIS2_PLACEMENT_3D ( 'NONE', #1384, #30496, #30166 ) ;
#29346=CARTESIAN_POINT ( 'NONE',  ( -23.83861932771936765, -15.61961844720760340, 5.310552105000033052 ) ) ;
#29348=CARTESIAN_POINT ( 'NONE',  ( -24.33897390745588751, -13.43341002469357548, 4.640669265424538281 ) ) ;
#29352=CARTESIAN_POINT ( 'NONE',  ( 14.53700916270368459, -27.90446693802870826, 0.2374258030000131470 ) ) ;
#29357=CARTESIAN_POINT ( 'NONE',  ( -0.6094664100040195764, -28.49364619262437870, 4.999998581000003384 ) ) ;
#29373=CARTESIAN_POINT ( 'NONE',  ( -24.30808044443811156, 13.48997716914403533, 3.899998581000013509 ) ) ;
#29377=CARTESIAN_POINT ( 'NONE',  ( 24.34137756859324853, -13.42980563341176037, 6.099998581000020792 ) ) ;
#29384=CARTESIAN_POINT ( 'NONE',  ( -24.98081131316241255, -13.71897606304888662, 4.895818166000015736 ) ) ;
#29398=CARTESIAN_POINT ( 'NONE',  ( -17.36983091284663061, -9.971084190247578860, -0.6999999999999784173 ) ) ;
#29403=CARTESIAN_POINT ( 'NONE',  ( 24.78870453580057998, -12.58522324566301620, 4.492873455000018446 ) ) ;
#29405=ORIENTED_EDGE ( 'NONE', *, *, #11241, .F. ) ;
#29408=ORIENTED_EDGE ( 'NONE', *, *, #24170, .F. ) ;
#29411=CARTESIAN_POINT ( 'NONE',  ( 28.68577476828162531, -9.950727360111285336, 1.000000000000000888 ) ) ;
#29414=B_SPLINE_CURVE_WITH_KNOTS ( 'NONE', 3,
 ( #23541, #14241, #14400, #28708, #9350, #21477 ),
 .UNSPECIFIED., .F., .F.,
 ( 4, 2, 4 ),
 ( 0.000000000000000000, 0.5000000000000000000, 1.000000000000000000 ),
 .UNSPECIFIED. ) ;
#29426=CARTESIAN_POINT ( 'NONE',  ( 24.30808045080437907, -13.48997717272881047, 6.099998581000020792 ) ) ;
#29431=CARTESIAN_POINT ( 'NONE',  ( 1.605176535610508326, -27.75389821387976852, 4.999998581000003384 ) ) ;
#29433=CARTESIAN_POINT ( 'NONE',  ( 22.97695743748386832, 16.89262754991261062, 7.000000000000006217 ) ) ;
#29434=ORIENTED_EDGE ( 'NONE', *, *, #2843, .T. ) ;
#29445=ORIENTED_EDGE ( 'NONE', *, *, #12099, .F. ) ;
#29452=CARTESIAN_POINT ( 'NONE',  ( 16.08958307947758470, -8.732827806336466381, -0.6999999999999784173 ) ) ;
#29455=CARTESIAN_POINT ( 'NONE',  ( -24.06826084733133797, 20.50742046740553093, 8.000000000000007105 ) ) ;
#29479=ORIENTED_EDGE ( 'NONE', *, *, #22964, .F. ) ;
#29488=CARTESIAN_POINT ( 'NONE',  ( 16.06675444873834380, 10.97998838177521286, -1.000005633855494125E-09 ) ) ;
#29492=EDGE_LOOP ( 'NONE', ( #4067, #14137, #27470, #2853 ) ) ;
#29495=CARTESIAN_POINT ( 'NONE',  ( 24.60726958085803417, -14.37955347769869263, 4.098597479000015475 ) ) ;
#29502=CARTESIAN_POINT ( 'NONE',  ( -21.71008920740291259, 18.50699696262706695, 5.000000064000004407 ) ) ;
#29508=CARTESIAN_POINT ( 'NONE',  ( 14.60916111670818474, -28.04296597385482315, 1.000000000000000888 ) ) ;
#29515=CARTESIAN_POINT ( 'NONE',  ( -0.5821515579339680002, -27.79407096281863687, 5.208100973000007627 ) ) ;
#29524=CARTESIAN_POINT ( 'NONE',  ( 26.79556473285982321, 0.4875557887250580036, 0.000000000000000000 ) ) ;
#29534=AXIS2_PLACEMENT_3D ( 'NONE', #2885, #21779, #21629 ) ;
#29535=CARTESIAN_POINT ( 'NONE',  ( 24.83272649506304219, -12.49791454618707398, 5.208434320000010942 ) ) ;
#29540=CARTESIAN_POINT ( 'NONE',  ( -24.98081131316241255, -13.71897606304888662, 4.999998581000003384 ) ) ;
#29552=EDGE_CURVE ( 'NONE', #10592, #6458, #15357, .T. ) ;
#29555=ORIENTED_EDGE ( 'NONE', *, *, #7045, .T. ) ;
#29557=VECTOR ( 'NONE', #16190, 1000.000000000000000 ) ;
#29562=EDGE_CURVE ( 'NONE', #16870, #20235, #16973, .T. ) ;
#29565=EDGE_LOOP ( 'NONE', ( #4915, #367, #28679, #8851 ) ) ;
#29568=CARTESIAN_POINT ( 'NONE',  ( -17.62053209685469923, -9.769114620074489608, 0.000000000000000000 ) ) ;
#29582=CARTESIAN_POINT ( 'NONE',  ( 16.40303402077768169, -9.791839085275103827, -0.6999999989999727834 ) ) ;
#29587=CARTESIAN_POINT ( 'NONE',  ( -20.30403093128963476, 20.00000000003735323, 3.000000106999994642 ) ) ;
#29592=AXIS2_PLACEMENT_3D ( 'NONE', #17572, #20406, #15217 ) ;
#29595=ORIENTED_EDGE ( 'NONE', *, *, #30961, .F. ) ;
#29602=EDGE_CURVE ( 'NONE', #2709, #28983, #25510, .T. ) ;
#29607=CARTESIAN_POINT ( 'NONE',  ( 17.04201355691706610, -10.10244847084225484, 0.000000000000000000 ) ) ;
#29609=CARTESIAN_POINT ( 'NONE',  ( 16.27441336928229276, -8.340546694414939566, -0.6999999999999783062 ) ) ;
#29611=CARTESIAN_POINT ( 'NONE',  ( -24.95427444319612675, 13.76797446832583560, 6.099998581000020792 ) ) ;
#29612=CARTESIAN_POINT ( 'NONE',  ( -23.81866442513004856, -14.33570206453694240, 6.099998581000020792 ) ) ;
#29616=ORIENTED_EDGE ( 'NONE', *, *, #21380, .T. ) ;
#29628=CARTESIAN_POINT ( 'NONE',  ( -0.8926240818011654810, 3.415131430766678022, -0.6999999999999784173 ) ) ;
#29637=CARTESIAN_POINT ( 'NONE',  ( -27.85782817081202012, 2.925281790394680836, 8.000000000000007105 ) ) ;
#29646=CARTESIAN_POINT ( 'NONE',  ( 23.62421573330318836, 14.65442405561991634, 6.042470792000015578 ) ) ;
#29650=CARTESIAN_POINT ( 'NONE',  ( -28.44355746342733227, 4.375812428242645602, 0.2374258030000131470 ) ) ;
#29655=CARTESIAN_POINT ( 'NONE',  ( 16.47468026044998268, -8.132810122024002553, -4.336808689942017736E-16 ) ) ;
#29662=CARTESIAN_POINT ( 'NONE',  ( -24.29748893039695545, -13.50839063705114995, 4.437671896236813573 ) ) ;
#29666=CARTESIAN_POINT ( 'NONE',  ( -28.35455043824866550, -0.5159221438580923191, 0.2374258030000131470 ) ) ;
#29669=CARTESIAN_POINT ( 'NONE',  ( 24.39135169767337885, -14.74223403355047068, 4.689353541000001790 ) ) ;
#29672=DIRECTION ( 'NONE',  ( 0.000000000000000000, 0.000000000000000000, -1.000000000000000000 ) ) ;
#29684=CARTESIAN_POINT ( 'NONE',  ( 27.71261514784112379, 0.5042418800004094814, 0.5514269430000329208 ) ) ;
#29688=CARTESIAN_POINT ( 'NONE',  ( 25.32653163311281830, -13.07087917458821202, 4.239730452999995514 ) ) ;
#29689=CARTESIAN_POINT ( 'NONE',  ( -22.90527192528401201, 16.36193184990112570, 8.000000000000007105 ) ) ;
#29692=CARTESIAN_POINT ( 'NONE',  ( 24.37165445055180157, -14.77472140295711434, 4.999998581000003384 ) ) ;
#29693=CARTESIAN_POINT ( 'NONE',  ( 16.37473331889771089, 11.76353838340827984, -0.6999999989999727834 ) ) ;
#29696=CARTESIAN_POINT ( 'NONE',  ( 24.41841038956698640, 14.69667349781389376, 3.899998581000013509 ) ) ;
#29699=CARTESIAN_POINT ( 'NONE',  ( 28.49528339128749366, 0.5184828350247886464, 8.000000000000007105 ) ) ;
#29721=ORIENTED_EDGE ( 'NONE', *, *, #4535, .T. ) ;
#29722=CARTESIAN_POINT ( 'NONE',  ( 23.87170004953230773, 14.24726900334573187, 3.904031772999999816 ) ) ;
#29731=B_SPLINE_CURVE_WITH_KNOTS ( 'NONE', 3,
 ( #27109, #22396, #22695, #3642, #3333, #5543, #17352, #12942, #25209, #1301 ),
 .UNSPECIFIED., .F., .F.,
 ( 4, 2, 2, 2, 4 ),
 ( 0.000000000000000000, 0.2500000000000000000, 0.5000000000000000000, 0.7500000000000000000, 1.000000000000000000 ),
 .UNSPECIFIED. ) ;
#29735=CARTESIAN_POINT ( 'NONE',  ( -17.59696554489119080, -9.791838634853515799, 0.000000000000000000 ) ) ;
#29741=CARTESIAN_POINT ( 'NONE',  ( 21.13530760622606763, 17.06006193239099034, -0.6999999999999784173 ) ) ;
#29743=CARTESIAN_POINT ( 'NONE',  ( 23.55411374389282386, 16.04538543799059980, 8.000000000000007105 ) ) ;
#29749=CARTESIAN_POINT ( 'NONE',  ( 17.83929309184204826, 20.00000000005427125, -0.3499999999999892086 ) ) ;
#29753=ORIENTED_EDGE ( 'NONE', *, *, #23158, .T. ) ;
#29754=ORIENTED_EDGE ( 'NONE', *, *, #29552, .T. ) ;
#29761=CARTESIAN_POINT ( 'NONE',  ( -0.3076636919214117971, -28.49867017228250177, 5.759626916000016195 ) ) ;
#29769=CARTESIAN_POINT ( 'NONE',  ( 16.37473331889771089, 11.76353838340827984, 0.000000000000000000 ) ) ;
#29780=DIRECTION ( 'NONE',  ( 0.000000000000000000, 0.000000000000000000, -1.000000000000000000 ) ) ;
#29785=EDGE_CURVE ( 'NONE', #18702, #19859, #16861, .T. ) ;
#29790=ORIENTED_EDGE ( 'NONE', *, *, #12310, .F. ) ;
#29791=CARTESIAN_POINT ( 'NONE',  ( -24.81746041937532965, 14.01353061208509310, 3.920132063000014710 ) ) ;
#29795=CARTESIAN_POINT ( 'NONE',  ( -22.59122543795706051, 17.98290286765915980, 0.5017677510000262409 ) ) ;
#29798=CARTESIAN_POINT ( 'NONE',  ( -25.41286868644903763, 12.90211872717319430, 4.492873454000012146 ) ) ;
#29806=CARTESIAN_POINT ( 'NONE',  ( 17.14656078602323319, -7.900182044548062166, -0.6999999999999784173 ) ) ;
#29807=CARTESIAN_POINT ( 'NONE',  ( -16.85343921394901301, 12.09981795542885585, -0.6999999999999784173 ) ) ;
#29809=CARTESIAN_POINT ( 'NONE',  ( 24.08512461539509175, 13.58911351521636490, 0.02487527300001901587 ) ) ;
#29815=FACE_OUTER_BOUND ( 'NONE', #27498, .T. ) ;
#29820=CARTESIAN_POINT ( 'NONE',  ( -0.5944614571882205212, -27.79380703160649446, 5.104049977999985721 ) ) ;
#29827=ORIENTED_EDGE ( 'NONE', *, *, #11639, .T. ) ;
#29829=EDGE_CURVE ( 'NONE', #7420, #21140, #25111, .T. ) ;
#29831=CARTESIAN_POINT ( 'NONE',  ( -4.667733413579616908, -30.93201666723582122, 1.000000002999990034 ) ) ;
#29838=CARTESIAN_POINT ( 'NONE',  ( -19.80535357367646654, 19.50875577052770993, 6.600000000000022737 ) ) ;
#29842=CARTESIAN_POINT ( 'NONE',  ( 25.05552768372066907, -13.58331698798256504, 6.079865069000017996 ) ) ;
#29847=EDGE_CURVE ( 'NONE', #25327, #3809, #28512, .T. ) ;
#29849=CARTESIAN_POINT ( 'NONE',  ( 27.77990052945810362, 1.357541147587897568, 8.000000000000007105 ) ) ;
#29868=ORIENTED_EDGE ( 'NONE', *, *, #11490, .T. ) ;
#29869=SHAPE_DEFINITION_REPRESENTATION ( #20370, #3523 ) ;
#29874=ORIENTED_EDGE ( 'NONE', *, *, #25816, .T. ) ;
#29875=CARTESIAN_POINT ( 'NONE',  ( 24.06826093652101051, -20.50742065841456707, 1.000000000000000888 ) ) ;
#29876=CARTESIAN_POINT ( 'NONE',  ( -0.4781950147703600273, -27.79606941020783140, 5.495819603435045053 ) ) ;
#29878=CARTESIAN_POINT ( 'NONE',  ( -27.77052805885580966, -0.5052956280425524582, 0.7069222069999991920 ) ) ;
#29883=AXIS2_PLACEMENT_3D ( 'NONE', #23807, #4596, #14203 ) ;
#29894=CARTESIAN_POINT ( 'NONE',  ( -25.77914833267782413, -15.40383343775964065, 8.000000000000007105 ) ) ;
#29904=CARTESIAN_POINT ( 'NONE',  ( 23.35655559247464907, 15.07705663187610945, 5.680691777000007825 ) ) ;
#29920=CARTESIAN_POINT ( 'NONE',  ( -24.32472894358752313, 13.45989150749028873, 6.099998581000020792 ) ) ;
#29921=CARTESIAN_POINT ( 'NONE',  ( -24.29460412914614764, -13.51351735463393311, 5.558304235695046280 ) ) ;
#29955=CARTESIAN_POINT ( 'NONE',  ( -21.67076946895560852, 17.25020827395983503, -0.6577119969999878357 ) ) ;
#29966=CARTESIAN_POINT ( 'NONE',  ( -21.02347494288676444, 19.26966991725469214, 4.000000085000010586 ) ) ;
#29967=CARTESIAN_POINT ( 'NONE',  ( 27.79539923781770483, 0.5057481688777585305, 1.000000000000000888 ) ) ;
#29972=ORIENTED_EDGE ( 'NONE', *, *, #10437, .T. ) ;
#29978=CARTESIAN_POINT ( 'NONE',  ( -24.05209696821570731, 13.94187115378248976, 5.961515049095109653 ) ) ;
#29986=CARTESIAN_POINT ( 'NONE',  ( 27.98121187870611593, -9.706323496128696604, 1.000000000000000888 ) ) ;
#29990=CARTESIAN_POINT ( 'NONE',  ( 0.01829671460970255098, 3.547951512854722100, 0.000000000000000000 ) ) ;
#29991=CARTESIAN_POINT ( 'NONE',  ( -26.79566689313578109, 10.13197864253886848, 8.000000000000007105 ) ) ;
#29995=CARTESIAN_POINT ( 'NONE',  ( -14.60916135985672071, 28.04296594682689658, 8.000000000000007105 ) ) ;
#30026=VERTEX_POINT ( 'NONE', #23183 ) ;
#30029=CARTESIAN_POINT ( 'NONE',  ( -17.93031264004542891, -9.094488044133550275, 0.000000000000000000 ) ) ;
#30031=CARTESIAN_POINT ( 'NONE',  ( -0.6094664100040195764, -28.49364619262437870, 4.999998581000003384 ) ) ;
#30056=CARTESIAN_POINT ( 'NONE',  ( 23.94466869970572986, 15.45669658583985751, 5.680691777000007825 ) ) ;
#30082=CARTESIAN_POINT ( 'NONE',  ( 23.77684695985370311, -14.40559418229910449, 4.854156763425871546 ) ) ;
#30090=CARTESIAN_POINT ( 'NONE',  ( -26.02053815395284175, 12.91565460411935895, 1.000000000000000888 ) ) ;
#30102=CARTESIAN_POINT ( 'NONE',  ( -23.77308074856162889, 14.41182440783502550, 4.853949414814223040 ) ) ;
#30112=FACE_OUTER_BOUND ( 'NONE', #15678, .T. ) ;
#30113=EDGE_CURVE ( 'NONE', #25714, #20192, #22888, .T. ) ;
#30120=CARTESIAN_POINT ( 'NONE',  ( -25.12046394328327281, 13.46291001840482160, 3.957489296000010981 ) ) ;
#30124=CARTESIAN_POINT ( 'NONE',  ( 24.37165445055180157, -14.77472140295711434, 4.895781291000017355 ) ) ;
#30127=CARTESIAN_POINT ( 'NONE',  ( 17.14656078599760392, 12.09981795542235439, -1.000005633855494125E-09 ) ) ;
#30130=CARTESIAN_POINT ( 'NONE',  ( 24.63996007208032779, 13.90215428157462263, 0.5514267500000280542 ) ) ;
#30135=CARTESIAN_POINT ( 'NONE',  ( 24.27467683999808301, -13.55001166052597128, 3.904029272000009154 ) ) ;
#30139=B_SPLINE_CURVE_WITH_KNOTS ( 'NONE', 5,
 ( #833, #15139, #5385, #3025, #22541, #10576, #12618, #20170, #29761, #8191, #17795, #8664, #18261, #17942, #27555 ),
 .UNSPECIFIED., .F., .F.,
 ( 6, 3, 3, 3, 6 ),
 ( 0.000000000000000000, 0.09999999999828219910, 0.3999999999988547716, 0.6999999999999999556, 1.000000000000000000 ),
 .UNSPECIFIED. ) ;
#30147=FACE_OUTER_BOUND ( 'NONE', #12571, .T. ) ;
#30149=CARTESIAN_POINT ( 'NONE',  ( -20.20536873837831493, -21.08852116449837766, 0.5514282400000125595 ) ) ;
#30153=CARTESIAN_POINT ( 'NONE',  ( 25.41286869299526074, -12.90211872965451079, 4.492873455000018446 ) ) ;
#30154=CARTESIAN_POINT ( 'NONE',  ( -23.55444264242456498, 16.04540112444970390, 8.000000000000007105 ) ) ;
#30155=CARTESIAN_POINT ( 'NONE',  ( -24.72757892072304742, 14.23267199169132979, 8.000000000000007105 ) ) ;
#30158=ORIENTED_EDGE ( 'NONE', *, *, #4629, .F. ) ;
#30160=CARTESIAN_POINT ( 'NONE',  ( 1.060521003860056405E-06, 19.99999999974424725, -0.6999999999999784173 ) ) ;
#30166=DIRECTION ( 'NONE',  ( 0.7198537139083028835, -0.6941258031311204890, 0.000000000000000000 ) ) ;
#30168=CARTESIAN_POINT ( 'NONE',  ( -26.66783967069105898, -7.507193849635574345, 0.000000000000000000 ) ) ;
#30172=CARTESIAN_POINT ( 'NONE',  ( 26.93696268452645626, 0.4901285798022169127, 0.000000000000000000 ) ) ;
#30203=CARTESIAN_POINT ( 'NONE',  ( -19.68703433251029722, 19.53817007346649248, 0.6302326600000074386 ) ) ;
#30204=CARTESIAN_POINT ( 'NONE',  ( -20.59280845669432836, -19.92816138975910434, 8.000000000000007105 ) ) ;
#30206=CARTESIAN_POINT ( 'NONE',  ( 25.21071572825679752, 14.22418740194451914, 0.2374258030000131470 ) ) ;
#30211=CARTESIAN_POINT ( 'NONE',  ( 23.39354070784786543, 15.01969649483752001, 5.760134169000008519 ) ) ;
#30215=CARTESIAN_POINT ( 'NONE',  ( 3.040504021322313122, 1.733590290792417887, -0.5999999999999894307 ) ) ;
#30219=DIRECTION ( 'NONE',  ( 0.000000000000000000, 0.000000000000000000, -1.000000000000000000 ) ) ;
#30231=CARTESIAN_POINT ( 'NONE',  ( -0.5716039300045591132, -28.49445895580208443, 4.689815098000011062 ) ) ;
#30240=EDGE_CURVE ( 'NONE', #24241, #17421, #8850, .T. ) ;
#30241=CARTESIAN_POINT ( 'NONE',  ( 24.32472724076343695, -13.45989056521276872, 6.099998581000020792 ) ) ;
#30262=VECTOR ( 'NONE', #8016, 1000.000000000000000 ) ;
#30263=EDGE_LOOP ( 'NONE', ( #25121, #12, #30724, #6027 ) ) ;
#30288=CARTESIAN_POINT ( 'NONE',  ( 24.22335707914676206, 13.66710489523639716, 0.08279771000002655867 ) ) ;
#30292=CARTESIAN_POINT ( 'NONE',  ( -23.23955040174346465, -15.25661106733265981, 5.208368890000008911 ) ) ;
#30298=B_SPLINE_CURVE_WITH_KNOTS ( 'NONE', 3,
 ( #4933, #2575, #2730, #21934, #28540, #24445 ),
 .UNSPECIFIED., .F., .F.,
 ( 4, 2, 4 ),
 ( 0.000000000000000000, 0.5000000000000000000, 1.000000000000000000 ),
 .UNSPECIFIED. ) ;
#30316=EDGE_CURVE ( 'NONE', #2709, #2704, #24113, .T. ) ;
#30320=CARTESIAN_POINT ( 'NONE',  ( -19.80535357377644701, 19.50875577052588739, 3.000000106999994642 ) ) ;
#30327=CARTESIAN_POINT ( 'NONE',  ( -28.49530731802708416, -0.5184832703812605192, 8.000000000000007105 ) ) ;
#30328=CARTESIAN_POINT ( 'NONE',  ( -16.04158896040112126, -9.763537949678049443, 0.000000000000000000 ) ) ;
#30349=EDGE_CURVE ( 'NONE', #19387, #8936, #6567, .T. ) ;
#30352=VERTEX_POINT ( 'NONE', #19857 ) ;
#30359=CARTESIAN_POINT ( 'NONE',  ( -16.70716219490313392, -7.897520476984252191, -0.6999999999999784173 ) ) ;
#30363=CARTESIAN_POINT ( 'NONE',  ( 25.26019821377178687, -13.19871658671780246, 5.889015030805896167 ) ) ;
#30369=CARTESIAN_POINT ( 'NONE',  ( 24.15916138403057190, 13.75451189100735050, 4.118302008711519413 ) ) ;
#30372=CARTESIAN_POINT ( 'NONE',  ( 21.99937703061004513, -17.24463697064632228, 8.000000000000007105 ) ) ;
#30379=CARTESIAN_POINT ( 'NONE',  ( -17.80451178537096979, 11.53640331829313581, -4.336808689942018722E-16 ) ) ;
#30412=ADVANCED_FACE ( 'NONE', ( #27688 ), #1114, .F. ) ;
#30418=CARTESIAN_POINT ( 'NONE',  ( 0.9758793681798838549, -27.78334643822867633, 6.002515439000016606 ) ) ;
#30425=EDGE_LOOP ( 'NONE', ( #9847, #16785, #28441, #24084 ) ) ;
#30455=CARTESIAN_POINT ( 'NONE',  ( 27.08859402333795785, 0.4928875713623736554, 0.02487529600000981667 ) ) ;
#30457=B_SPLINE_CURVE_WITH_KNOTS ( 'NONE', 3,
 ( #11380, #30102, #13580, #20821, #23506, #30582, #25229, #9009, #6648, #23031 ),
 .UNSPECIFIED., .F., .F.,
 ( 4, 2, 2, 2, 4 ),
 ( 0.000000000000000000, 0.2500000000000000000, 0.5000000000000000000, 0.7500000000000000000, 1.000000000000000000 ),
 .UNSPECIFIED. ) ;
#30472=VERTEX_POINT ( 'NONE', #25031 ) ;
#30474=ADVANCED_FACE ( 'NONE', ( #3785 ), #7527, .T. ) ;
#30477=CARTESIAN_POINT ( 'NONE',  ( -27.11420065481265951, -7.632847749032011464, 0.08279779300002232389 ) ) ;
#30481=B_SPLINE_CURVE_WITH_KNOTS ( 'NONE', 5,
 ( #5095, #17515, #3344, #20187, #852, #21945 ),
 .UNSPECIFIED., .F., .F.,
 ( 6, 6 ),
 ( 65.40639850639999509, 88.32365686489998780 ),
 .UNSPECIFIED. ) ;
#30482=CARTESIAN_POINT ( 'NONE',  ( -23.29312071521372118, -15.17488101142239643, 4.493007575000013354 ) ) ;
#30484=CARTESIAN_POINT ( 'NONE',  ( -15.73360964037622622, -8.979988381802643360, -0.6999999989999727834 ) ) ;
#30486=CARTESIAN_POINT ( 'NONE',  ( 0.4368970292349217965, -27.79681690464249044, 3.901345920999998995 ) ) ;
#30487=CARTESIAN_POINT ( 'NONE',  ( -16.81341597784800967, -10.09981795476353739, 0.000000000000000000 ) ) ;
#30488=CARTESIAN_POINT ( 'NONE',  ( -22.97593529893700648, 15.65128280014837081, 8.000000000000007105 ) ) ;
#30490=FACE_OUTER_BOUND ( 'NONE', #30263, .T. ) ;
#30493=CARTESIAN_POINT ( 'NONE',  ( -17.93302393987574206, -8.945477793833122249, 0.000000000000000000 ) ) ;
#30496=DIRECTION ( 'NONE',  ( 0.000000000000000000, 0.000000000000000000, -1.000000000000000000 ) ) ;
#30497=CARTESIAN_POINT ( 'NONE',  ( -15.96459051028835674, -8.309720466557573459, -0.6999999999999784173 ) ) ;
#30505=ORIENTED_EDGE ( 'NONE', *, *, #23099, .F. ) ;
#30523=ORIENTED_EDGE ( 'NONE', *, *, #28904, .T. ) ;
#30527=CARTESIAN_POINT ( 'NONE',  ( 23.96481830933180035, 14.09066012006225854, 3.927868778737001243 ) ) ;
#30528=CARTESIAN_POINT ( 'NONE',  ( -19.29841003509485375, 19.63499152630128108, 0.3044381840000276451 ) ) ;
#30529=CARTESIAN_POINT ( 'NONE',  ( -10.23626208557738515, -26.01105658336103943, 8.000000000000007105 ) ) ;
#30532=CARTESIAN_POINT ( 'NONE',  ( 27.21969913503883731, 9.853839689487985609, 0.2374258030000131470 ) ) ;
#30534=CARTESIAN_POINT ( 'NONE',  ( -22.03724970760471180, 17.02913761663678827, 6.333333369000054169 ) ) ;
#30549=ORIENTED_EDGE ( 'NONE', *, *, #24471, .F. ) ;
#30551=CARTESIAN_POINT ( 'NONE',  ( 23.69427943123108093, 14.54081805611945910, 3.920145809000019632 ) ) ;
#30568=CARTESIAN_POINT ( 'NONE',  ( -25.07525407549810836, 13.54704386626776547, 6.073823031254199201 ) ) ;
#30570=CARTESIAN_POINT ( 'NONE',  ( 24.32472724076343695, -13.45989056521276872, 6.099998581000020792 ) ) ;
#30582=CARTESIAN_POINT ( 'NONE',  ( -23.99220715881088495, 14.04440917687116475, 4.117401770955998686 ) ) ;
#30588=CARTESIAN_POINT ( 'NONE',  ( 24.81746042555073117, -14.01353061617342455, 6.079865098000015067 ) ) ;
#30596=CARTESIAN_POINT ( 'NONE',  ( -18.87720858757026576, 21.16361474422994604, 0.2374258030000131470 ) ) ;
#30600=CARTESIAN_POINT ( 'NONE',  ( -20.06472444662395560, 19.99998854834754525, 0.2590520886679497647 ) ) ;
#30617=CARTESIAN_POINT ( 'NONE',  ( 16.19686700502921539, 11.53824530203521448, -0.6999999999999785283 ) ) ;
#30629=CARTESIAN_POINT ( 'NONE',  ( 24.73369734551975085, -12.69281744145431290, 4.322410792677205293 ) ) ;
#30632=CARTESIAN_POINT ( 'NONE',  ( -27.39555917266975982, -7.712052243925962891, 0.2686740700000300741 ) ) ;
#30638=CARTESIAN_POINT ( 'NONE',  ( -1.758512962375676780, 3.081546181689937658, 0.000000000000000000 ) ) ;
#30639=CARTESIAN_POINT ( 'NONE',  ( 0.03549436698350039859, -27.80040766163043031, 3.997479608999987555 ) ) ;
#30650=CARTESIAN_POINT ( 'NONE',  ( -16.06988921239048551, -8.208160914692745891, -0.6999999989999727834 ) ) ;
#30656=LINE ( 'NONE', #25778, #10798 ) ;
#30671=CARTESIAN_POINT ( 'NONE',  ( 1.645560275461343203, -28.45273235261698019, 4.999998581000003384 ) ) ;
#30672=CARTESIAN_POINT ( 'NONE',  ( -26.93696268452645981, -0.4901285798020276196, 0.000000000000000000 ) ) ;
#30677=CARTESIAN_POINT ( 'NONE',  ( 25.33388806075444322, -13.05639290569185285, 5.735287129097097925 ) ) ;
#30680=CARTESIAN_POINT ( 'NONE',  ( 27.03594125075309762, 0.4919295335571094996, -0.6999999999999784173 ) ) ;
#30683=CARTESIAN_POINT ( 'NONE',  ( -20.30403093138962234, 20.00000000003553424, 1.000000000000000888 ) ) ;
#30686=CARTESIAN_POINT ( 'NONE',  ( 0.2655682516278248806, -27.79918151443105856, 3.920205022000022854 ) ) ;
#30689=EDGE_LOOP ( 'NONE', ( #6611, #12727, #28290, #20083, #13757, #20633, #7773, #23734 ) ) ;
#30690=CARTESIAN_POINT ( 'NONE',  ( 22.97559295455008765, 15.65128684778802715, 8.000000000000007105 ) ) ;
#30700=VERTEX_POINT ( 'NONE', #25230 ) ;
#30702=SURFACE_STYLE_USAGE ( .BOTH. , #11350 ) ;
#30710=ORIENTED_EDGE ( 'NONE', *, *, #10606, .T. ) ;
#30721=CARTESIAN_POINT ( 'NONE',  ( 23.91557559422898649, -14.17419444102282000, 5.732984736081180976 ) ) ;
#30724=ORIENTED_EDGE ( 'NONE', *, *, #27575, .F. ) ;
#30730=CARTESIAN_POINT ( 'NONE',  ( -19.80535357377644701, 19.50875577052588739, 3.000000106999994642 ) ) ;
#30737=CARTESIAN_POINT ( 'NONE',  ( 26.79556473285982321, 0.4875557887249851730, -0.6999999999999784173 ) ) ;
#30747=CARTESIAN_POINT ( 'NONE',  ( -18.65448805331473991, 19.99991030667355218, -0.6087647090073780021 ) ) ;
#30752=EDGE_LOOP ( 'NONE', ( #11615, #6697, #23027, #26109 ) ) ;
#30754=CARTESIAN_POINT ( 'NONE',  ( 1.605176535610508326, -27.75389821387976852, 4.895940783000013674 ) ) ;
#30776=B_SPLINE_CURVE_WITH_KNOTS ( 'NONE', 3,
 ( #14080, #2281, #4793, #16726, #7301, #7143, #9033, #4478, #30913, #6830, #18942, #6672 ),
 .UNSPECIFIED., .F., .F.,
 ( 4, 2, 2, 2, 2, 4 ),
 ( 0.000000000000000000, 0.2500000000000006661, 0.5000000000000013323, 0.6250000000000016653, 0.7500000000000019984, 1.000000000000000000 ),
 .UNSPECIFIED. ) ;
#30781=CARTESIAN_POINT ( 'NONE',  ( -23.83861932771936765, -15.61961844720760340, 4.689445057000002137 ) ) ;
#30797=FACE_OUTER_BOUND ( 'NONE', #17410, .T. ) ;
#30800=EDGE_CURVE ( 'NONE', #30026, #18612, #30986, .T. ) ;
#30804=CARTESIAN_POINT ( 'NONE',  ( -17.59696597919420213, 10.20816091468181774, 0.000000000000000000 ) ) ;
#30813=EDGE_CURVE ( 'NONE', #170, #14439, #29082, .T. ) ;
#30817=CARTESIAN_POINT ( 'NONE',  ( -27.07233446881437899, 8.380004974182886812, 6.600000000000022737 ) ) ;
#30819=VECTOR ( 'NONE', #22528, 1000.000000000000000 ) ;
#30821=CARTESIAN_POINT ( 'NONE',  ( 27.98121187870611593, -9.706323496128696604, 1.000000000000000888 ) ) ;
#30822=CARTESIAN_POINT ( 'NONE',  ( -16.85343921394901301, 12.09981795542885585, -1.000005633855494125E-09 ) ) ;
#30824=AXIS2_PLACEMENT_3D ( 'NONE', #17770, #27846, #20149 ) ;
#30830=CARTESIAN_POINT ( 'NONE',  ( 24.92257222434601616, 14.03654374138045213, 8.000000000000007105 ) ) ;
#30832=CARTESIAN_POINT ( 'NONE',  ( 28.68577476828162531, -9.950727360111285336, 0.7595836940000044724 ) ) ;
#30833=CARTESIAN_POINT ( 'NONE',  ( -19.56375666326936269, 19.56885676738829005, 0.5004811919999962999 ) ) ;
#30834=CARTESIAN_POINT ( 'NONE',  ( -3.313783883474008984, -27.85733552065744334, 8.000000000000007105 ) ) ;
#30836=CARTESIAN_POINT ( 'NONE',  ( 26.95478617150206802, 4.952129227130185107, -0.6999999999999784173 ) ) ;
#30855=VERTEX_POINT ( 'NONE', #7875 ) ;
#30857=CARTESIAN_POINT ( 'NONE',  ( 23.35655559247464907, 15.07705663187610945, 4.319305385000027364 ) ) ;
#30862=CARTESIAN_POINT ( 'NONE',  ( 19.39238560432175973, 20.00003183196481871, -0.3307242700730367857 ) ) ;
#30863=EDGE_CURVE ( 'NONE', #26866, #4259, #25035, .T. ) ;
#30873=CARTESIAN_POINT ( 'NONE',  ( -1.790201522669007561, -3.063245535112757434, 0.000000000000000000 ) ) ;
#30879=CARTESIAN_POINT ( 'NONE',  ( 1.645560275461343203, -28.45273235261698019, 4.999998581000003384 ) ) ;
#30908=CARTESIAN_POINT ( 'NONE',  ( -20.22090452287337925, 20.00040987029326800, 0.5517657372802144966 ) ) ;
#30913=CARTESIAN_POINT ( 'NONE',  ( -23.29644702443709292, -15.16961937508697922, 4.504162582432789996 ) ) ;
#30924=CARTESIAN_POINT ( 'NONE',  ( 16.10061776502996622, -9.307365792519414427, -0.6999999999999784173 ) ) ;
#30940=CARTESIAN_POINT ( 'NONE',  ( -19.80535397421925481, 19.50875616500616871, 0.9999999989999952543 ) ) ;
#30941=LINE ( 'NONE', #26068, #22555 ) ;
#30954=CARTESIAN_POINT ( 'NONE',  ( -25.32653162617393861, 13.07087917251410403, 4.239730451999990102 ) ) ;
#30959=CARTESIAN_POINT ( 'NONE',  ( 18.05873143885011345, 10.34054669329053944, -0.6999999999999783062 ) ) ;
#30961=EDGE_CURVE ( 'NONE', #6970, #28945, #9945, .T. ) ;
#30973=CARTESIAN_POINT ( 'NONE',  ( -27.87609112763809449, 3.928995115440388375, 8.000000000000007105 ) ) ;
#30976=CARTESIAN_POINT ( 'NONE',  ( -27.79539923781770483, -0.5057481688778081574, 1.000000000000000888 ) ) ;
#30984=CARTESIAN_POINT ( 'NONE',  ( 28.34729902996195250, 3.134625972213187062, 8.000000000000007105 ) ) ;
#30985=CARTESIAN_POINT ( 'NONE',  ( 24.35797964201644561, -13.39969403546014703, 6.098655031999994591 ) ) ;
#30986=B_SPLINE_CURVE_WITH_KNOTS ( 'NONE', 5,
 ( #21443, #4914, #2095, #11686, #28816, #9793, #12143, #31041, #26165, #21751, #4599, #28674, #7118, #26320, #24118 ),
 .UNSPECIFIED., .F., .F.,
 ( 6, 3, 3, 3, 6 ),
 ( 0.000000000000000000, 0.1000000000045810078, 0.4000000000011452173, 0.7000000000005727196, 1.000000000000000000 ),
 .UNSPECIFIED. ) ;
#30988=CARTESIAN_POINT ( 'NONE',  ( -15.73360964098195147, -8.979988381493612337, 0.000000000000000000 ) ) ;
#30998=VERTEX_POINT ( 'NONE', #11340 ) ;
#31007=CARTESIAN_POINT ( 'NONE',  ( -17.12044415977894474, -10.06939460809101305, 0.000000000000000000 ) ) ;
#31010=CARTESIAN_POINT ( 'NONE',  ( 23.47637528925400474, 14.89020703987135086, 4.098700193000015091 ) ) ;
#31013=CARTESIAN_POINT ( 'NONE',  ( 18.62931254531553549, 19.99998787143272949, -0.6145042232417567973 ) ) ;
#31023=FACE_OUTER_BOUND ( 'NONE', #3613, .T. ) ;
#31036=CARTESIAN_POINT ( 'NONE',  ( 18.13765659361598281, 10.46359668135569976, -4.336808689942018722E-16 ) ) ;
#31038=EDGE_LOOP ( 'NONE', ( #15399, #1026, #15669, #25420 ) ) ;
#31041=CARTESIAN_POINT ( 'NONE',  ( 24.06750537026301018, 15.26514225575822081, 4.098700193000015091 ) ) ;
#31043=EDGE_LOOP ( 'NONE', ( #28782, #19966, #21519, #29172, #850, #29251, #16016, #7390 ) ) ;
#31048=CARTESIAN_POINT ( 'NONE',  ( 28.35455043824866550, 0.5159221438580617880, 0.2374258030000131470 ) ) ;
#31068=FACE_OUTER_BOUND ( 'NONE', #748, .T. ) ;
#31085=CARTESIAN_POINT ( 'NONE',  ( 23.80092420482279891, 14.36517094565843777, 6.099998581000020792 ) ) ;
#31087=CARTESIAN_POINT ( 'NONE',  ( -20.80531994253358974, 17.08514196121145545, 0.000000000000000000 ) ) ;
#31104=CARTESIAN_POINT ( 'NONE',  ( 22.03727920249266248, 17.02869341850189855, 6.333333333333394322 ) ) ;
ENDSEC;
END-ISO-10303-21;
